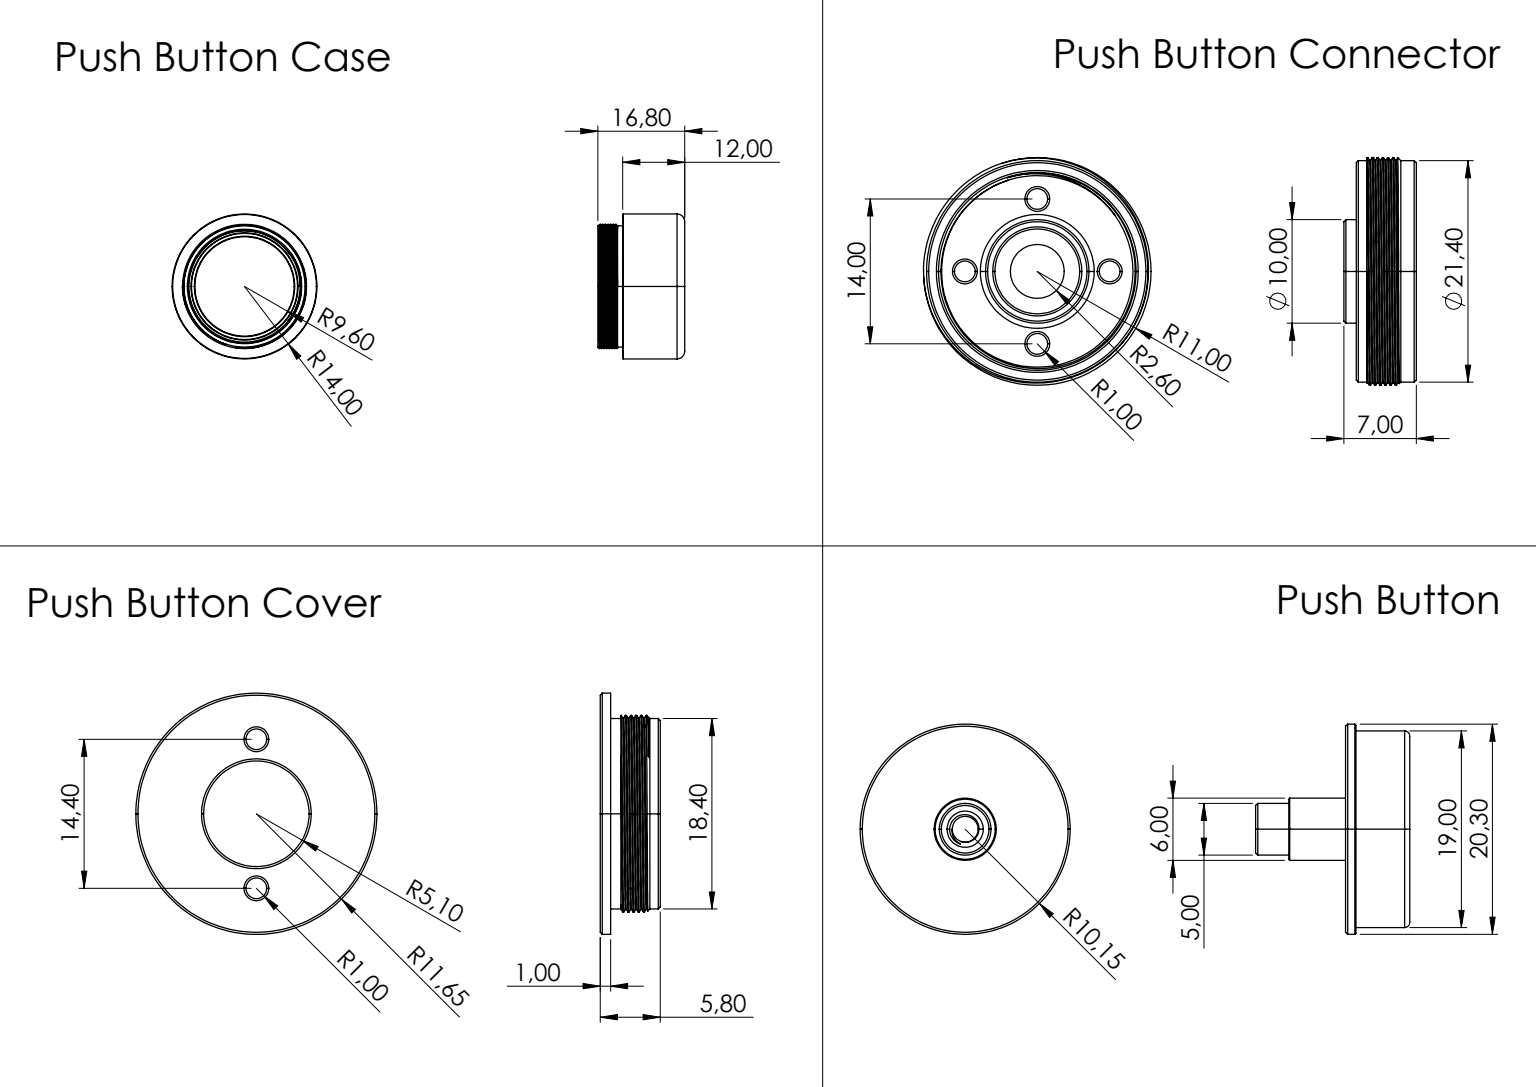
ISO-10303-21;
HEADER;
FILE_DESCRIPTION (('STEP AP214'),
    '1' );
FILE_NAME ('Push Button Connector.step',
    '2026-10-07T19:06:49',
    ( '' ),
    ( '' ),
    'SwSTEP 2.0',
    'SolidWorks 2020',
    '' );
FILE_SCHEMA (( 'AUTOMOTIVE_DESIGN' ));
ENDSEC;

DATA;
#1=CIRCLE ( 'NONE', #2803, 1.199999999999999956 ) ;
#7=CARTESIAN_POINT ( 'NONE',  ( 5.443609589771999602, -77.26340414414998747, 9.675369385899999841 ) ) ;
#13=CARTESIAN_POINT ( 'NONE',  ( 8.944729675425000082, -79.55274183760799644, 3.923329690209000908 ) ) ;
#25=CARTESIAN_POINT ( 'NONE',  ( 8.240135455977000589, -77.95571942709864288, -5.125512367919999868 ) ) ;
#26=CARTESIAN_POINT ( 'NONE',  ( 6.712914363625387182, -79.91051976297769954, 6.366836982130202216 ) ) ;
#27=CARTESIAN_POINT ( 'NONE',  ( -10.75000000000000000, -80.44999999999998863, 5.225043809877999334E-10 ) ) ;
#29=CARTESIAN_POINT ( 'NONE',  ( 7.764258067048000811, -77.05084123326183487, 5.767450660628000492 ) ) ;
#34=B_SPLINE_SURFACE_WITH_KNOTS ( 'NONE', 3, 3, ( 
 ( #2089, #37490, #2662, #20656, #6495, #56101, #24505, #42521, #42233, #28631, #6789, #20087, #38079, #55512, #1505, #24796, #1797, #15059, #42810, #33053, #25080, #24214, #38655, #46967, #15646, #19794, #43104, #51683, #56674, #55808, #19495, #11231, #29210, #7079, #2374 ),
 ( #11521, #15360, #29498, #51101, #47553, #10652, #47257, #41935, #28333, #32758, #46681, #50806, #38365, #51387, #56387, #15937, #33925, #6201, #33354, #10944, #10350, #46384, #5908, #23917, #28924, #44244, #34791, #3513, #4087, #3796, #20938, #21798, #39803, #57525, #44532 ),
 ( #52815, #57816, #48399, #17375, #35362, #53387, #12933, #7650, #48682, #38940, #56957, #21514, #30931, #16518, #48971, #8512, #21224, #17086, #26506, #43963, #3233, #22085, #35069, #40099, #16230, #34209, #53105, #12654, #52246, #30648, #12085, #8226, #43380, #12370, #11803 ),
 ( #39520, #25649, #48118, #7364, #26228, #34499, #29777, #47833, #43675, #25364, #2939, #39229, #52528, #30067, #57242, #16806, #30358, #7936, #25938, #36844, #4690, #584, #41281, #27399, #45139, #46026, #18566, #5547, #54856, #9997, #36557, #54579, #14403, #14119, #53990 ) ),
 .UNSPECIFIED., .F., .F., .F.,
 ( 4, 4 ),
 ( 4, 1, 1, 1, 1, 1, 1, 1, 1, 1, 1, 1, 1, 1, 1, 1, 1, 1, 1, 1, 1, 1, 1, 1, 1, 1, 1, 1, 1, 1, 1, 1, 4 ),
 ( -0.1387574078320999993, 1.138757407831999968 ),
 ( 0.3298824860954999716, 0.3512342696267000131, 0.3725860531579999746, 0.3939378366892999916, 0.4152896202206000087, 0.4366414037517999946, 0.4579931872831000117, 0.4793449708143999732, 0.5006967543456000147, 0.5220485378768999762, 0.5434003214082000488, 0.5647521049395000103, 0.5861038884707000518, 0.6074556720019999023, 0.6288074555332999749, 0.6501592390646000474, 0.6715110225957999779, 0.6928628061271000504, 0.7142145896584000120, 0.7355663731896000535, 0.7569181567209000150, 0.7782699402522000875, 0.7996217237835000491, 0.8209735073147000906, 0.8423252908460000521, 0.8636770743773000136, 0.8850288579085000551, 0.9063806414398000166, 0.9277324249710999782, 0.9490842085024000507, 0.9704359920335999812, 0.9917877755649000537, 1.013139559096000175 ),
 .UNSPECIFIED. ) ;
#41=CARTESIAN_POINT ( 'NONE',  ( 9.855576673225998618, -79.76811006564999218, -5.230603033304000782 ) ) ;
#47=ORIENTED_EDGE ( 'NONE', *, *, #21166, .F. ) ;
#51=DIRECTION ( 'NONE',  ( 0.000000000000000000, 0.000000000000000000, -1.000000000000000000 ) ) ;
#66=CARTESIAN_POINT ( 'NONE',  ( -6.405050160242000246, -78.85473773677898635, 8.912875463421000788 ) ) ;
#67=CARTESIAN_POINT ( 'NONE',  ( 11.00000000000000000, -79.34999999999999432, -1.064824513673000067E-14 ) ) ;
#79=CARTESIAN_POINT ( 'NONE',  ( -5.793600105730999594, -78.22586176634699484, 9.408086495002001115 ) ) ;
#108=CARTESIAN_POINT ( 'NONE',  ( -6.065106684382000068, -77.35143450949497890, 9.224892016835999797 ) ) ;
#116=CARTESIAN_POINT ( 'NONE',  ( 9.009247259181924150, -78.72916666666665719, -2.421167930323326001 ) ) ;
#118=ORIENTED_EDGE ( 'NONE', *, *, #11311, .T. ) ;
#125=EDGE_CURVE ( 'NONE', #28960, #7174, #2934, .T. ) ;
#130=CARTESIAN_POINT ( 'NONE',  ( 11.22519961651999942, -80.38483504313998651, 1.998589004412999692 ) ) ;
#158=CARTESIAN_POINT ( 'NONE',  ( 0.000000000000000000, -75.19999999999998863, -4.999999999999962697 ) ) ;
#163=CARTESIAN_POINT ( 'NONE',  ( -5.539808784079908399, -79.51666666666666572, 9.611650271896829523 ) ) ;
#170=AXIS2_PLACEMENT_3D ( 'NONE', #825, #36799, #54241 ) ;
#173=CARTESIAN_POINT ( 'NONE',  ( -6.000000000000000000, -81.99999999999998579, 0.000000000000000000 ) ) ;
#189=CARTESIAN_POINT ( 'NONE',  ( -7.843978203195000276, -77.65945010111499869, 5.713380375430999969 ) ) ;
#192=DIRECTION ( 'NONE',  ( 0.000000000000000000, -1.000000000000000000, 0.000000000000000000 ) ) ;
#206=CYLINDRICAL_SURFACE ( 'NONE', #36450, 4.100000000000000533 ) ;
#224=CARTESIAN_POINT ( 'NONE',  ( -0.5444512524326000635, -78.07738533478699594, -9.506521396690999381 ) ) ;
#235=CARTESIAN_POINT ( 'NONE',  ( 3.166366903731000271, -79.72244757809599491, 10.47195928638999973 ) ) ;
#236=LINE ( 'NONE', #58354, #29407 ) ;
#244=ORIENTED_EDGE ( 'NONE', *, *, #50771, .T. ) ;
#256=CARTESIAN_POINT ( 'NONE',  ( 7.620617093578522905, -78.80203626096795233, -5.244489908162002223 ) ) ;
#258=CARTESIAN_POINT ( 'NONE',  ( -7.396886230003165252, -77.65219327641052871, -5.684603129138253053 ) ) ;
#262=VECTOR ( 'NONE', #19954, 1000.000000000000000 ) ;
#267=EDGE_CURVE ( 'NONE', #43339, #56949, #56033, .T. ) ;
#271=CARTESIAN_POINT ( 'NONE',  ( 8.599926684958175471, -79.81921486858095705, -3.562059774102686038 ) ) ;
#279=FACE_OUTER_BOUND ( 'NONE', #48060, .T. ) ;
#291=CARTESIAN_POINT ( 'NONE',  ( 0.8649477812003000254, -78.46126277754198952, -9.701111330267998767 ) ) ;
#292=VECTOR ( 'NONE', #35631, 1000.000000000000227 ) ;
#312=CARTESIAN_POINT ( 'NONE',  ( 8.944729675425000082, -79.61304476327899238, 3.923329690209000908 ) ) ;
#323=CARTESIAN_POINT ( 'NONE',  ( -7.203390125892000562, -78.80843430096776103, -6.502451851937000704 ) ) ;
#324=CARTESIAN_POINT ( 'NONE',  ( 8.238920321119756807, -79.88802510210236107, 4.204434926243399318 ) ) ;
#327=CARTESIAN_POINT ( 'NONE',  ( -9.497876546326999403, -77.25168256874098915, -0.2008509664869000122 ) ) ;
#328=CARTESIAN_POINT ( 'NONE',  ( 0.09829970619593025871, -77.22591789683764318, -9.271508350125035491 ) ) ;
#330=AXIS2_PLACEMENT_3D ( 'NONE', #48177, #7132, #57011 ) ;
#349=CARTESIAN_POINT ( 'NONE',  ( -7.229693382246000333, -78.82924743682598034, -6.526195624661000672 ) ) ;
#358=CARTESIAN_POINT ( 'NONE',  ( -9.091539081997000338, -78.88283009111098920, 6.148815634104000338 ) ) ;
#369=CARTESIAN_POINT ( 'NONE',  ( -7.138937464960999790, -79.17331078153999613, 8.574798629027000629 ) ) ;
#390=CARTESIAN_POINT ( 'NONE',  ( -3.539318067648058452, -78.19389790816430263, -8.545993076014068990 ) ) ;
#396=CARTESIAN_POINT ( 'NONE',  ( 1.433348699817989180, -77.46263244500043754, 9.138269204909326149 ) ) ;
#397=CARTESIAN_POINT ( 'NONE',  ( 7.528714304401000312, -78.05456459179299600, -8.074838600060001426 ) ) ;
#399=CARTESIAN_POINT ( 'NONE',  ( 4.186942200393000135, -78.55095460635199345, -8.754440266352000677 ) ) ;
#404=CARTESIAN_POINT ( 'NONE',  ( -10.78159125964999987, -79.41561974942199242, 1.856099740267000087 ) ) ;
#409=VERTEX_POINT ( 'NONE', #50221 ) ;
#410=EDGE_CURVE ( 'NONE', #18942, #44068, #5336, .T. ) ;
#420=CARTESIAN_POINT ( 'NONE',  ( -11.13667185325999931, -80.13800688576898779, -2.444338232200999439 ) ) ;
#426=AXIS2_PLACEMENT_3D ( 'NONE', #17397, #35382, #53716 ) ;
#427=CARTESIAN_POINT ( 'NONE',  ( 9.684822944874866835, -77.90969691107382289, -5.379607873393639217 ) ) ;
#435=AXIS2_PLACEMENT_3D ( 'NONE', #56778, #6892, #24899 ) ;
#444=CARTESIAN_POINT ( 'NONE',  ( 7.559982449049000408, -77.02655527933319490, -6.032732969207000195 ) ) ;
#448=DIRECTION ( 'NONE',  ( 0.000000000000000000, -1.000000000000000000, 0.000000000000000000 ) ) ;
#458=ORIENTED_EDGE ( 'NONE', *, *, #10797, .T. ) ;
#474=CARTESIAN_POINT ( 'NONE',  ( -1.959694873104000257, -77.31836415156699616, -9.504225410855001499 ) ) ;
#491=CARTESIAN_POINT ( 'NONE',  ( 10.25292700656883760, -77.20000000000000284, -3.413936412999044823 ) ) ;
#498=FACE_OUTER_BOUND ( 'NONE', #54806, .T. ) ;
#499=CARTESIAN_POINT ( 'NONE',  ( 3.414307247564000392, -79.67572032229998058, 9.134133468150000823 ) ) ;
#500=EDGE_CURVE ( 'NONE', #21107, #21244, #3663, .T. ) ;
#507=FACE_OUTER_BOUND ( 'NONE', #47869, .T. ) ;
#510=CARTESIAN_POINT ( 'NONE',  ( 1.825776387079000029, -78.88028063292298953, 9.234594473601999809 ) ) ;
#518=PRODUCT_DEFINITION ( 'UNKNOWN', '', #41419, #21544 ) ;
#522=CARTESIAN_POINT ( 'NONE',  ( -10.75843888410000027, -79.38533932610398836, -1.985902594052000092 ) ) ;
#541=CARTESIAN_POINT ( 'NONE',  ( 0.000000000000000000, -74.99999999999998579, 0.000000000000000000 ) ) ;
#547=CARTESIAN_POINT ( 'NONE',  ( -1.374291557126987362, -78.71317509820548253, -9.148177845238967265 ) ) ;
#552=CARTESIAN_POINT ( 'NONE',  ( -9.250401410528953150, -77.61051319238347901, -1.210813435511432834 ) ) ;
#560=CARTESIAN_POINT ( 'NONE',  ( 2.902193781656972504, -80.00000000000000000, 8.901354151454830443 ) ) ;
#568=EDGE_CURVE ( 'NONE', #9279, #11445, #48735, .T. ) ;
#575=B_SPLINE_SURFACE_WITH_KNOTS ( 'NONE', 3, 3, ( 
 ( #12579, #9256, #48608, #54128, #29991, #34424, #52454, #57162, #48044, #8155, #7577, #25576, #21148, #39156, #26155, #46752, #46163, #1286, #33424, #51461, #37270, #11015, #28406, #50289, #28112, #9843, #10723, #36691, #23698, #15430, #1871, #41125, #19565, #36981, #27823, #50582, #28999, #41711, #18989, #45869, #28701, #19280, #54994, #47039, #33127, #19865, #5688, #1004, #6271, #24287, #10136, #23410, #6569, #55285, #42304, #14833, #37859, #55880, #719, #18697, #37566, #14543, #51169, #54706, #14250, #32536, #32830 ),
 ( #50875, #10421, #32246, #46453, #5402, #23988, #5981, #42004, #1572, #41421, #55581, #15129, #56458, #34575, #29282, #39020, #12159, #52608, #20445, #20159, #21300, #11301, #39308, #34863, #48195, #11594, #57318, #2158, #43753, #38441, #47910, #38148, #16012, #25728, #21014, #12443, #25441, #52893, #29855, #34001, #52037, #15718, #43460, #47331, #42886, #34289, #56748, #42596, #2732, #7149, #29570, #20731, #57032, #33714, #47626, #25151, #52323, #6860, #30438, #38729, #7442, #43177, #48469, #11877, #16308, #3017, #16591 ),
 ( #30145, #7727, #3306, #16882, #24580, #56170, #51751, #24868, #2443, #13596, #18336, #36328, #4752, #39595, #49044, #30719, #31886, #48754, #44315, #44035, #40764, #8301, #40472, #8590, #4460, #45204, #54353, #66, #358, #54060, #57892, #53767, #13892, #3871, #22754, #22460, #26578, #31593, #36036, #9182, #21871, #17448, #13006, #8012, #44905, #35736, #44612, #4167, #53464, #22165, #13303, #26009, #49635, #12726, #27167, #3585, #49340, #21588, #40172, #57598, #26301, #17159, #35145, #53176, #39879, #35435, #31006 ),
 ( #58185, #17748, #31296, #8886, #26881, #18044, #32756, #41932, #10348, #1217, #23914, #27461, #41637, #50509, #55510, #46676, #28331, #46381, #6199, #5905, #45796, #1503, #18630, #28042, #24212, #45499, #5331, #5614, #1795, #14179, #42231, #19493, #37199, #14758, #50803, #37488, #19208, #55212, #645, #51098, #15057, #33051, #10649, #28629, #19792, #46088, #37786, #23625, #54641, #36907, #55806, #15358, #49930, #9475, #23044, #32463, #32176, #5046, #50216, #27752, #41059, #36622, #9764, #23338, #10062, #41350, #932 ) ),
 .UNSPECIFIED., .F., .F., .F.,
 ( 4, 4 ),
 ( 4, 1, 1, 1, 1, 1, 1, 1, 1, 1, 1, 1, 1, 1, 1, 1, 1, 1, 1, 1, 1, 1, 1, 1, 1, 1, 1, 1, 1, 1, 1, 1, 1, 1, 1, 1, 1, 1, 1, 1, 1, 1, 1, 1, 1, 1, 1, 1, 1, 1, 1, 1, 1, 1, 1, 1, 1, 1, 1, 1, 1, 1, 1, 1, 4 ),
 ( -0.4045438850611000059, 1.404543885061000141 ),
 ( -0.02000000000000000042, -0.003749999999999999861, 0.01250000000000000069, 0.02875000000000000125, 0.04499999999999999833, 0.06124999999999999889, 0.07749999999999999944, 0.09375000000000000000, 0.1100000000000000006, 0.1262500000000000011, 0.1424999999999999878, 0.1587500000000000022, 0.1749999999999999889, 0.1912500000000000033, 0.2074999999999999900, 0.2237500000000000044, 0.2399999999999999911, 0.2562499999999999778, 0.2725000000000000200, 0.2887500000000000067, 0.3049999999999999933, 0.3212499999999999800, 0.3375000000000000222, 0.3537500000000000089, 0.3699999999999999956, 0.3862499999999999822, 0.4025000000000000244, 0.4187500000000000111, 0.4349999999999999978, 0.4512499999999999845, 0.4675000000000000266, 0.4837500000000000133, 0.5000000000000000000, 0.5162499999999999867, 0.5324999999999999734, 0.5487499999999999600, 0.5649999999999999467, 0.5812500000000000444, 0.5975000000000000311, 0.6137500000000000178, 0.6300000000000000044, 0.6462499999999999911, 0.6624999999999999778, 0.6787499999999999645, 0.6949999999999999512, 0.7112500000000000488, 0.7275000000000000355, 0.7437500000000000222, 0.7600000000000000089, 0.7762499999999999956, 0.7924999999999999822, 0.8087499999999999689, 0.8249999999999999556, 0.8412500000000000533, 0.8575000000000000400, 0.8737500000000000266, 0.8900000000000000133, 0.9062500000000000000, 0.9224999999999999867, 0.9387499999999999734, 0.9549999999999999600, 0.9712499999999999467, 0.9875000000000000444, 1.003749999999999920, 1.020000000000000018 ),
 .UNSPECIFIED. ) ;
#577=AXIS2_PLACEMENT_3D ( 'NONE', #17957, #12922, #35948 ) ;
#582=CARTESIAN_POINT ( 'NONE',  ( -8.623695280723000067, -78.29071980276798115, 4.526762133323999571 ) ) ;
#584=CARTESIAN_POINT ( 'NONE',  ( 5.916979755548000597, -79.44684362032798219, -7.926218594775000348 ) ) ;
#591=ADVANCED_FACE ( 'NONE', ( #7938 ), #54289, .F. ) ;
#596=CARTESIAN_POINT ( 'NONE',  ( -7.370930946996000266, -78.06097405823999225, -8.448440252239999282 ) ) ;
#603=CARTESIAN_POINT ( 'NONE',  ( -4.465297566879000257, -79.92309116543150083, 8.686876450551999085 ) ) ;
#604=VERTEX_POINT ( 'NONE', #30650 ) ;
#614=CARTESIAN_POINT ( 'NONE',  ( 7.027773501905277165, -79.90642805933067905, 6.014294227121073533 ) ) ;
#617=CARTESIAN_POINT ( 'NONE',  ( 2.632967082928999947, -77.10305996719816335, 9.306700570505000769 ) ) ;
#638=CARTESIAN_POINT ( 'NONE',  ( -9.375068251199000002, -78.22531894259199703, -2.204836785425999590 ) ) ;
#645=CARTESIAN_POINT ( 'NONE',  ( 10.74341457190999982, -79.22405656010899122, -2.245675826504000216 ) ) ;
#658=CARTESIAN_POINT ( 'NONE',  ( 10.92979202429999930, -79.06863239632698992, 1.617881315982000245 ) ) ;
#661=VECTOR ( 'NONE', #54709, 1000.000000000000000 ) ;
#665=CARTESIAN_POINT ( 'NONE',  ( 8.318716844523411424, -78.25665627052904938, 7.160083125396178083 ) ) ;
#668=ORIENTED_EDGE ( 'NONE', *, *, #34683, .T. ) ;
#684=ORIENTED_EDGE ( 'NONE', *, *, #58361, .T. ) ;
#687=CARTESIAN_POINT ( 'NONE',  ( -1.468596516428545717, -77.48775315375499417, 9.132634440082403771 ) ) ;
#688=CARTESIAN_POINT ( 'NONE',  ( -10.79754810892000094, -77.44686363549098473, -2.301543980133000211 ) ) ;
#690=CARTESIAN_POINT ( 'NONE',  ( 7.405962610586999340, -77.52424149029599221, -6.270759699041999369 ) ) ;
#695=CARTESIAN_POINT ( 'NONE',  ( -3.661365483191000081, -79.33134268642398013, 10.30932680317000028 ) ) ;
#707=CARTESIAN_POINT ( 'NONE',  ( 0.000000000000000000, -75.19999999999998863, 0.000000000000000000 ) ) ;
#710=CARTESIAN_POINT ( 'NONE',  ( -9.163349670171998085, -78.09756746102598868, -2.155044623588000086 ) ) ;
#719=CARTESIAN_POINT ( 'NONE',  ( 9.233664981878000333, -79.60499486974998717, 5.933249305785000871 ) ) ;
#720=CIRCLE ( 'NONE', #32727, 1.000000000000000000 ) ;
#728=CARTESIAN_POINT ( 'NONE',  ( -11.25716098398999954, -78.18238734777798982, -0.4530573336216000002 ) ) ;
#731=CARTESIAN_POINT ( 'NONE',  ( 7.764258067048000811, -77.13099274720589449, 5.767450660628000492 ) ) ;
#734=CARTESIAN_POINT ( 'NONE',  ( -1.297526016723000053, -78.46556992798305430, -10.89864408161000142 ) ) ;
#735=DIRECTION ( 'NONE',  ( -1.000000000000000000, 0.000000000000000000, 0.000000000000000000 ) ) ;
#753=CARTESIAN_POINT ( 'NONE',  ( 3.185848383111141935, -78.25305747739967899, -8.692436244180706595 ) ) ;
#763=CARTESIAN_POINT ( 'NONE',  ( 2.260091721765999928, -78.85325092453199147, -9.437303113984999214 ) ) ;
#779=CARTESIAN_POINT ( 'NONE',  ( 0.04837777540751588695, -77.19999999999998863, -10.99285280508881080 ) ) ;
#780=EDGE_LOOP ( 'NONE', ( #684, #45447, #45553, #30245 ) ) ;
#781=CARTESIAN_POINT ( 'NONE',  ( -1.439896632895311113, -78.31458333333333144, -11.00000000000000355 ) ) ;
#784=CARTESIAN_POINT ( 'NONE',  ( 5.348414924440999307, -79.50038437275298975, -8.153793349671000001 ) ) ;
#787=EDGE_CURVE ( 'NONE', #12448, #10446, #50841, .T. ) ;
#789=CYLINDRICAL_SURFACE ( 'NONE', #25534, 11.00000000000000000 ) ;
#792=CARTESIAN_POINT ( 'NONE',  ( -11.06454125523000087, -77.73236022357899344, 1.497041118686999850 ) ) ;
#795=CARTESIAN_POINT ( 'NONE',  ( 4.459991035765999534, -77.79314704349698673, 8.413017068390001185 ) ) ;
#804=EDGE_LOOP ( 'NONE', ( #53108, #929, #5072, #12373 ) ) ;
#825=CARTESIAN_POINT ( 'NONE',  ( 0.000000000000000000, -74.64999999999999147, 0.000000000000000000 ) ) ;
#833=CARTESIAN_POINT ( 'NONE',  ( 0.03267024647290020511, -78.72542977318258295, -9.249861488902391571 ) ) ;
#836=CARTESIAN_POINT ( 'NONE',  ( -9.170121691637055150, -80.14671525588798318, -6.075096402074364299 ) ) ;
#841=CIRCLE ( 'NONE', #12100, 9.250000000000000000 ) ;
#854=FACE_OUTER_BOUND ( 'NONE', #17770, .T. ) ;
#870=VECTOR ( 'NONE', #48376, 1000.000000000000000 ) ;
#878=CARTESIAN_POINT ( 'NONE',  ( 8.003872304214999289, -77.24441679105500214, -8.008117534469000987 ) ) ;
#884=CARTESIAN_POINT ( 'NONE',  ( 6.728605944993000243, -79.69578255762351660, -7.080011783993000130 ) ) ;
#897=CARTESIAN_POINT ( 'NONE',  ( 9.249687267056886597, -79.85225412240586707, 0.2014328667283708241 ) ) ;
#910=CARTESIAN_POINT ( 'NONE',  ( 9.386754667005000385, -79.85238712864799027, 6.031619700400000283 ) ) ;
#922=ADVANCED_FACE ( 'NONE', ( #50957, #28492, #5484, #46543, #10509, #6065 ), #55373, .F. ) ;
#925=CARTESIAN_POINT ( 'NONE',  ( 8.177883213696999221, -77.91265682217398592, -5.086790354254000057 ) ) ;
#929=ORIENTED_EDGE ( 'NONE', *, *, #4950, .T. ) ;
#931=CARTESIAN_POINT ( 'NONE',  ( 5.684875707061095795, -77.92308321104999891, 7.397310562483891516 ) ) ;
#932=CARTESIAN_POINT ( 'NONE',  ( -10.69701368780000017, -79.98255012709098821, 1.066019776055000090 ) ) ;
#933=CARTESIAN_POINT ( 'NONE',  ( -10.71369944335147473, -79.12083333333333712, -2.879226727952079123 ) ) ;
#951=CARTESIAN_POINT ( 'NONE',  ( -2.421167930323375295, -79.89583333333331439, 9.009247259181911716 ) ) ;
#952=CARTESIAN_POINT ( 'NONE',  ( -0.5194061720425894313, -79.07133454617610369, -10.96348649343952353 ) ) ;
#955=EDGE_LOOP ( 'NONE', ( #118, #10532, #10822 ) ) ;
#960=CARTESIAN_POINT ( 'NONE',  ( 10.63539757175482059, -80.28072916675431259, -2.857308679526295414 ) ) ;
#971=CARTESIAN_POINT ( 'NONE',  ( 8.041760575514985021, -77.39131006114457989, 4.573409923808502420 ) ) ;
#972=CARTESIAN_POINT ( 'NONE',  ( -11.00724581733999941, -77.92400926547099971, 0.8512868710715000287 ) ) ;
#979=DIRECTION ( 'NONE',  ( 0.000000000000000000, 0.000000000000000000, -1.000000000000000000 ) ) ;
#980=CARTESIAN_POINT ( 'NONE',  ( 5.312973029106999867, -78.26383322178199364, 9.563478878364000124 ) ) ;
#988=FACE_OUTER_BOUND ( 'NONE', #44636, .T. ) ;
#994=FACE_OUTER_BOUND ( 'NONE', #35902, .T. ) ;
#997=FACE_OUTER_BOUND ( 'NONE', #46850, .T. ) ;
#999=ORIENTED_EDGE ( 'NONE', *, *, #41614, .F. ) ;
#1000=EDGE_CURVE ( 'NONE', #57298, #36426, #32062, .T. ) ;
#1001=CARTESIAN_POINT ( 'NONE',  ( 0.000000000000000000, -77.49999999999998579, 0.000000000000000000 ) ) ;
#1004=CARTESIAN_POINT ( 'NONE',  ( -10.81649518602000093, -79.29597897209099244, 1.862108609190000097 ) ) ;
#1033=VERTEX_POINT ( 'NONE', #32844 ) ;
#1040=CARTESIAN_POINT ( 'NONE',  ( 6.432069509746887626, -78.28619479064511211, -6.649389305992823296 ) ) ;
#1043=VERTEX_POINT ( 'NONE', #41143 ) ;
#1049=CARTESIAN_POINT ( 'NONE',  ( 4.545264886168000729, -77.60605771026999378, 8.573871732259998879 ) ) ;
#1065=B_SPLINE_CURVE_WITH_KNOTS ( 'NONE', 3,
 ( #13567, #49605, #16421, #24978, #38844, #21128, #30263, #34404, #16710, #29972, #33825, #29683, #34692, #38265, #33540, #29398, #51864, #11709, #47158 ),
 .UNSPECIFIED., .F., .F.,
 ( 4, 1, 1, 1, 1, 1, 1, 1, 1, 1, 1, 1, 1, 1, 1, 1, 4 ),
 ( 0.000000000000000000, 0.04500013125675292325, 0.1100001148193760075, 0.1750000983819555711, 0.2400000819445786693, 0.3050000655072017119, 0.3700000490698248656, 0.4350000326324479638, 0.5000000161948968680, 0.5649999997576505839, 0.6299999833204042998, 0.6949999668831581268, 0.7599999504454763022, 0.8249999340082300181, 0.8899999175709837340, 0.9549999011333020205, 1.000000000000000000 ),
 .UNSPECIFIED. ) ;
#1066=VERTEX_POINT ( 'NONE', #5137 ) ;
#1072=CARTESIAN_POINT ( 'NONE',  ( -0.09271117443256000901, -79.70494298055800186, 9.750963687110999700 ) ) ;
#1077=DIRECTION ( 'NONE',  ( 0.000000000000000000, 0.000000000000000000, -1.000000000000000000 ) ) ;
#1078=CARTESIAN_POINT ( 'NONE',  ( 4.884263559594000270, -77.83984273478799309, -10.16119218727999929 ) ) ;
#1079=EDGE_CURVE ( 'NONE', #43122, #24529, #36790, .T. ) ;
#1083=CARTESIAN_POINT ( 'NONE',  ( 3.151000900302999952, -78.36865170860198759, 8.870309342620000592 ) ) ;
#1088=CARTESIAN_POINT ( 'NONE',  ( 0.000000000000000000, -80.99999999999998579, 0.000000000000000000 ) ) ;
#1094=ORIENTED_EDGE ( 'NONE', *, *, #7570, .F. ) ;
#1108=CIRCLE ( 'NONE', #35958, 5.000000000000000000 ) ;
#1111=CARTESIAN_POINT ( 'NONE',  ( 6.983681292383111305, -78.53882967120196668, -6.738102358712994011 ) ) ;
#1117=CARTESIAN_POINT ( 'NONE',  ( 0.3203968975889366910, -78.72793535945164933, -9.244731248301008009 ) ) ;
#1121=CARTESIAN_POINT ( 'NONE',  ( -9.147467037885974150, -80.14699925185365714, -6.109202993256466208 ) ) ;
#1129=CARTESIAN_POINT ( 'NONE',  ( 9.499693205731109202, -80.00008708754018016, -1.997583897032410100E-06 ) ) ;
#1131=EDGE_CURVE ( 'NONE', #31999, #28960, #48632, .T. ) ;
#1138=CARTESIAN_POINT ( 'NONE',  ( 10.68454778250440640, -77.21060221147246239, 1.377222071623238620 ) ) ;
#1141=CARTESIAN_POINT ( 'NONE',  ( -2.928603948516999900, -78.74649347130959143, 10.57767911663000149 ) ) ;
#1148=CARTESIAN_POINT ( 'NONE',  ( 8.244325742278693525, -78.31259323136428918, -4.194771269908470934 ) ) ;
#1152=CARTESIAN_POINT ( 'NONE',  ( 1.867960828343000035, -78.75252915135698117, 9.447959161044998666 ) ) ;
#1153=DIRECTION ( 'NONE',  ( 0.000000000000000000, -1.000000000000000000, 0.000000000000000000 ) ) ;
#1165=CARTESIAN_POINT ( 'NONE',  ( -11.07550907487999936, -77.92372890012597964, 0.7607607059370000702 ) ) ;
#1172=CARTESIAN_POINT ( 'NONE',  ( 9.523132023602000729, -80.26946618684752366, 1.108936319727999997 ) ) ;
#1178=EDGE_CURVE ( 'NONE', #29062, #16887, #38796, .T. ) ;
#1183=CARTESIAN_POINT ( 'NONE',  ( 9.707557378189999753, -77.00399869373629258, -2.082535605504000298 ) ) ;
#1207=CARTESIAN_POINT ( 'NONE',  ( -2.552693750765000047, -78.31059042997900121, -9.286385980553001573 ) ) ;
#1211=ORIENTED_EDGE ( 'NONE', *, *, #32322, .T. ) ;
#1214=CARTESIAN_POINT ( 'NONE',  ( 4.658318423525466656, -77.93349885897991669, 8.082338094468221712 ) ) ;
#1217=CARTESIAN_POINT ( 'NONE',  ( -5.755176823513999729, -78.40937828446098479, 9.345691860246999383 ) ) ;
#1224=AXIS2_PLACEMENT_3D ( 'NONE', #7015, #33862, #6432 ) ;
#1231=CARTESIAN_POINT ( 'NONE',  ( 0.000000000000000000, -77.19999999999998863, 0.000000000000000000 ) ) ;
#1236=CARTESIAN_POINT ( 'NONE',  ( 9.694993915875986801, -79.66127398716234609, -5.145377715137363417 ) ) ;
#1237=LINE ( 'NONE', #18653, #57315 ) ;
#1238=ORIENTED_EDGE ( 'NONE', *, *, #38746, .F. ) ;
#1256=CARTESIAN_POINT ( 'NONE',  ( 8.765487326333861517, -77.37590140598007338, 2.954454027020771978 ) ) ;
#1264=LINE ( 'NONE', #48090, #9187 ) ;
#1265=CARTESIAN_POINT ( 'NONE',  ( 7.294482259529999624, -79.61226622975098621, -8.153425347847999660 ) ) ;
#1274=CARTESIAN_POINT ( 'NONE',  ( 0.000000000000000000, -80.35000000001998899, 0.000000000000000000 ) ) ;
#1277=CARTESIAN_POINT ( 'NONE',  ( -2.495045882587000108, -78.18283894841299286, -9.076670124625998426 ) ) ;
#1286=CARTESIAN_POINT ( 'NONE',  ( 2.550499813263000348, -78.45320834210998839, -10.67515654612000020 ) ) ;
#1288=EDGE_CURVE ( 'NONE', #26886, #33815, #5598, .T. ) ;
#1297=CARTESIAN_POINT ( 'NONE',  ( -2.226613147434000073, -78.07001793044798887, 11.04405396508999893 ) ) ;
#1305=VECTOR ( 'NONE', #37563, 1000.000000000000000 ) ;
#1308=CONICAL_SURFACE ( 'NONE', #57824, 9.431249999994999911, 0.7853981633972997312 ) ;
#1313=EDGE_LOOP ( 'NONE', ( #17606, #9356, #29670, #17047, #4604 ) ) ;
#1316=ORIENTED_EDGE ( 'NONE', *, *, #31004, .F. ) ;
#1323=CARTESIAN_POINT ( 'NONE',  ( 1.902005808056935310, -78.24161995856391627, -9.052334553967094521 ) ) ;
#1327=CARTESIAN_POINT ( 'NONE',  ( -8.805853231905880207, -77.57526559296016444, 2.831825794683833220 ) ) ;
#1331=CARTESIAN_POINT ( 'NONE',  ( -6.766389538252999714, -77.83344834330198125, -6.956053621355001049 ) ) ;
#1332=DIRECTION ( 'NONE',  ( -1.000000000000000000, 0.000000000000000000, 0.000000000000000000 ) ) ;
#1346=CARTESIAN_POINT ( 'NONE',  ( -1.210648453353548426, -79.48564454928481382, 9.248615044363743820 ) ) ;
#1349=CARTESIAN_POINT ( 'NONE',  ( 9.865351076058296087, -77.19999999999998863, -4.411030472467261987 ) ) ;
#1350=EDGE_LOOP ( 'NONE', ( #56104, #21727, #7177, #50239 ) ) ;
#1353=CARTESIAN_POINT ( 'NONE',  ( 1.439896632895317108, -79.06458333333331723, 10.99999999999999822 ) ) ;
#1357=DIRECTION ( 'NONE',  ( 0.000000000000000000, 0.000000000000000000, -1.000000000000000000 ) ) ;
#1359=CARTESIAN_POINT ( 'NONE',  ( -6.565417933280000895, -77.81803934957498825, -9.031084880605000365 ) ) ;
#1363=CARTESIAN_POINT ( 'NONE',  ( -8.420145992286000691, -77.48751300560297750, 3.744741888101000171 ) ) ;
#1383=ORIENTED_EDGE ( 'NONE', *, *, #50103, .T. ) ;
#1385=ORIENTED_EDGE ( 'NONE', *, *, #17552, .F. ) ;
#1394=CARTESIAN_POINT ( 'NONE',  ( 9.703646361260002351, -77.60084330994595803, 0.1143463288009116258 ) ) ;
#1397=B_SPLINE_CURVE_WITH_KNOTS ( 'NONE', 3,
 ( #16488, #34467, #48651, #35328, #26198, #53356, #25907, #12337, #48937, #12902, #30902, #39194, #43644, #8479, #43930, #16776, #22052, #21193, #52497, #39491, #48088, #57493, #3202, #12622, #30326, #40061, #48367, #17056, #35037, #53072, #14366, #49826, #14656, #54541, #37096, #41243, #23523, #9372, #40663, #36227, #35927, #27939, #54249, #256, #32654, #50706, #18239, #55112, #58374, #10246, #45987, #41534, #13782, #5233, #53957, #40957, #28229, #19104, #17936, #36805, #31783, #27362, #4942, #46281, #54824, #45694, #13494, #5806, #5514, #18524, #23237, #23813, #1117, #4655, #31485, #49530, #833, #9076, #36516, #27063, #22653, #32077, #45101, #45399, #22947, #547, #14082, #32366, #50118, #9662, #18814, #27652, #50409, #9959, #20561, #46867, #42711, #24982, #11138, #28818, #29685, #42127, #11711, #47737, #33828, #51866, #41831, #15252, #11419, #46575, #56289, #29400, #47453, #37687, #37388, #38559, #28526, #56575, #52153, #6978, #19987, #16133, #7270, #10842, #34110, #32949, #6394, #6101, #37976, #15840, #50993, #24409, #33244, #29114, #24110, #1405, #19396, #15546, #6690, #33542, #51581, #47160, #24699, #10542, #43003, #2560, #55407, #1693, #14952, #19686, #2277, #42425, #55703, #20274, #51287, #1994, #55999, #38268, #25271, #3704, #21130, #34695, #30265, #17578, #21708, #12562, #43290, #44438, #53299, #43874, #30560, #13130, #12844, #29974, #30843, #48877, #8137, #53591, #3423, #40001, #48025, #57439, #26416, #3990, #8419, #21993, #16712, #57719, #7559, #25558, #48591, #58016, #43578, #35565 ),
 .UNSPECIFIED., .F., .F.,
 ( 4, 2, 2, 1, 1, 1, 1, 1, 2, 2, 2, 2, 2, 1, 1, 1, 1, 1, 2, 2, 2, 2, 2, 1, 1, 1, 1, 2, 2, 2, 2, 2, 2, 2, 2, 1, 1, 1, 1, 2, 2, 2, 2, 2, 2, 2, 1, 1, 1, 1, 1, 2, 2, 2, 2, 2, 1, 1, 1, 2, 2, 2, 2, 1, 1, 1, 2, 2, 2, 2, 1, 1, 1, 1, 1, 2, 2, 2, 2, 2, 1, 1, 1, 2, 2, 2, 1, 2, 2, 1, 1, 2, 2, 2, 2, 2, 1, 2, 2, 2, 2, 2, 2, 2, 2, 1, 1, 1, 2, 2, 2, 2, 2, 2, 2, 2, 1, 1, 2, 4 ),
 ( 0.000000000000000000, 0.03124999999998840511, 0.04687499999998261807, 0.05468749999997975231, 0.05859374999997830208, 0.06054687499997758043, 0.06152343749997721267, 0.06201171874997703226, 0.06225585937497695593, 0.06249999999997687961, 0.09374999999996236344, 0.1093749999999550915, 0.1171874999999514694, 0.1210937499999496514, 0.1230468749999487216, 0.1240234374999482914, 0.1245117187499480693, 0.1247558593749479861, 0.1248779296874479167, 0.1249999999999478612, 0.1562499999999539535, 0.1718749999999570344, 0.1796874999999586442, 0.1835937499999594491, 0.1855468749999598932, 0.1865234374999601152, 0.1870117187499601985, 0.1872558593749602263, 0.1874999999999602263, 0.2031249999999644174, 0.2109374999999664713, 0.2148437499999675537, 0.2187499999999686362, 0.2343749999999729661, 0.2421874999999751310, 0.2460937499999762690, 0.2480468749999769074, 0.2490234374999772959, 0.2495117187499775180, 0.2497558593749775180, 0.2499999999999775180, 0.3124999999999837352, 0.3749999999999899525, 0.4374999999999962252, 0.4687499999999993894, 0.4843750000000009437, 0.4921875000000017208, 0.4960937500000021094, 0.4980468750000022760, 0.4990234375000023870, 0.4995117187500023870, 0.4997558593750024425, 0.5000000000000024425, 0.5312500000000072164, 0.5468750000000095479, 0.5546875000000107692, 0.5585937500000113243, 0.5605468750000116573, 0.5615234375000117684, 0.5620117187500118794, 0.5625000000000118794, 0.5937500000000155431, 0.6093750000000173195, 0.6171875000000182077, 0.6210937500000186517, 0.6230468750000188738, 0.6240234375000189848, 0.6250000000000189848, 0.6562500000000210942, 0.6718750000000220934, 0.6796875000000224265, 0.6835937500000226485, 0.6855468750000228706, 0.6865234375000229816, 0.6870117187500229816, 0.6872558593750229816, 0.6875000000000229816, 0.7187500000000279776, 0.7343750000000304201, 0.7421875000000316414, 0.7460937500000323075, 0.7480468750000325295, 0.7490234375000327516, 0.7495117187500327516, 0.7500000000000327516, 0.7812500000000329736, 0.7851562500000329736, 0.7856445312500329736, 0.7861328125000330846, 0.7871093750000330846, 0.7890625000000331957, 0.7968750000000335287, 0.8125000000000343059, 0.8203125000000346390, 0.8212890625000344169, 0.8222656250000343059, 0.8242187500000338618, 0.8281250000000331957, 0.8437500000000311973, 0.8515625000000301981, 0.8593750000000291989, 0.8750000000000273115, 0.8906250000000254241, 0.8925781250000250910, 0.8930664062500248690, 0.8935546875000247580, 0.8945312500000244249, 0.8984375000000235367, 0.9062500000000217604, 0.9375000000000144329, 0.9453125000000125455, 0.9492187500000116573, 0.9531250000000107692, 0.9687500000000071054, 0.9726562500000062172, 0.9736328125000059952, 0.9746093750000057732, 0.9765625000000053291, 0.9843750000000035527, 1.000000000000000000 ),
 .UNSPECIFIED. ) ;
#1398=CARTESIAN_POINT ( 'NONE',  ( -8.771427373352999268, -77.78517645232463451, -4.151237309591000013 ) ) ;
#1405=CARTESIAN_POINT ( 'NONE',  ( -7.198099468258734035, -78.65408334510459554, -5.809580251814940866 ) ) ;
#1408=DIRECTION ( 'NONE',  ( 1.000000000000000000, 0.000000000000000000, 0.000000000000000000 ) ) ;
#1418=CARTESIAN_POINT ( 'NONE',  ( 1.101534974885716833, -79.99999999999997158, 9.249201346533595824 ) ) ;
#1423=CARTESIAN_POINT ( 'NONE',  ( 9.250054636821570142, -79.84526209104460293, -0.6055073710143449306 ) ) ;
#1431=CARTESIAN_POINT ( 'NONE',  ( 9.233664981878000333, -79.64544880995556753, 5.933249305785000871 ) ) ;
#1436=CARTESIAN_POINT ( 'NONE',  ( 7.548260755434943903, -78.30112507871334060, -5.346425350760562800 ) ) ;
#1440=CARTESIAN_POINT ( 'NONE',  ( 6.930806504809000401, -78.58198617658298701, -6.687086896242999678 ) ) ;
#1442=CARTESIAN_POINT ( 'NONE',  ( -1.000000000000000000, -81.99999999999998579, -7.000000000000000000 ) ) ;
#1443=DIRECTION ( 'NONE',  ( 0.000000000000000000, 1.000000000000000000, 0.000000000000000000 ) ) ;
#1447=ORIENTED_EDGE ( 'NONE', *, *, #10114, .F. ) ;
#1453=CARTESIAN_POINT ( 'NONE',  ( -8.699139934798001406, -77.54738813692499377, -7.073312318721999503 ) ) ;
#1461=CARTESIAN_POINT ( 'NONE',  ( -9.687172913667000174, -80.02050914020550465, -1.248753675804000096 ) ) ;
#1465=EDGE_CURVE ( 'NONE', #49740, #9279, #54779, .T. ) ;
#1471=CARTESIAN_POINT ( 'NONE',  ( -1.850935023731000051, -77.10928756760588954, 9.663325317366000533 ) ) ;
#1489=CARTESIAN_POINT ( 'NONE',  ( 7.792609338710000166, -77.13002767319579789, 5.788510568612999840 ) ) ;
#1494=CARTESIAN_POINT ( 'NONE',  ( -4.491587152465999822, -78.85767126595499121, -8.642068059767000321 ) ) ;
#1501=CARTESIAN_POINT ( 'NONE',  ( 9.250000000000000000, -77.84999999999999432, 0.000000000000000000 ) ) ;
#1503=CARTESIAN_POINT ( 'NONE',  ( 10.94409238582999855, -78.74648653645297713, 0.8311789410725000105 ) ) ;
#1505=CARTESIAN_POINT ( 'NONE',  ( -6.756755724436000143, -79.51665000578398690, 6.762936965852000881 ) ) ;
#1509=ADVANCED_FACE ( 'NONE', ( #10204 ), #6533, .F. ) ;
#1520=CARTESIAN_POINT ( 'NONE',  ( 10.92224869643393070, -78.20263265991563628, 0.3426835237561569047 ) ) ;
#1524=VERTEX_POINT ( 'NONE', #16378 ) ;
#1541=CARTESIAN_POINT ( 'NONE',  ( 8.744325593625859483, -77.37646171839476494, 3.016781543199777094 ) ) ;
#1544=CARTESIAN_POINT ( 'NONE',  ( 4.545264886168000729, -77.72666356161099088, 8.573871732259998879 ) ) ;
#1549=CARTESIAN_POINT ( 'NONE',  ( -6.447812191272999982, -78.91764840355199340, 8.972380486426999369 ) ) ;
#1562=CARTESIAN_POINT ( 'NONE',  ( -9.411482030169999291, -78.58077255621898871, -0.1876179646513999877 ) ) ;
#1572=CARTESIAN_POINT ( 'NONE',  ( -2.169167664939000151, -78.26068007878699007, 10.75912301088999889 ) ) ;
#1573=DIRECTION ( 'NONE',  ( 0.000000000000000000, -1.000000000000000000, 0.000000000000000000 ) ) ;
#1585=CARTESIAN_POINT ( 'NONE',  ( 9.267785752250999209, -77.88273556822998955, -6.128505448192000493 ) ) ;
#1590=DIRECTION ( 'NONE',  ( -1.000000000000000000, 0.000000000000000000, 0.000000000000000000 ) ) ;
#1603=VERTEX_POINT ( 'NONE', #57101 ) ;
#1609=CARTESIAN_POINT ( 'NONE',  ( 6.558477970958472625, -78.28771851464713905, -6.522947137475199497 ) ) ;
#1611=EDGE_CURVE ( 'NONE', #3961, #32937, #13372, .T. ) ;
#1613=VERTEX_POINT ( 'NONE', #15795 ) ;
#1620=CARTESIAN_POINT ( 'NONE',  ( 9.051070938631999852, -77.54921005201198625, 3.499832029064999794 ) ) ;
#1638=DIRECTION ( 'NONE',  ( 0.000000000000000000, 1.000000000000000000, 0.000000000000000000 ) ) ;
#1640=CARTESIAN_POINT ( 'NONE',  ( 3.469760739495959978, -77.20000000000000284, -10.38643556155824577 ) ) ;
#1645=CARTESIAN_POINT ( 'NONE',  ( 6.760013919724070064, -79.02291666666666003, 8.796335266379978535 ) ) ;
#1647=CARTESIAN_POINT ( 'NONE',  ( 1.640398859540999954, -80.09569838644598860, -9.391438764149000917 ) ) ;
#1653=CARTESIAN_POINT ( 'NONE',  ( -8.051994348227001552, -77.30396459359899097, -7.735023745693999864 ) ) ;
#1656=CARTESIAN_POINT ( 'NONE',  ( -5.004442145019999622, -77.60120832211899256, -7.972877152348999630 ) ) ;
#1662=VECTOR ( 'NONE', #23671, 1000.000000000000000 ) ;
#1664=DIRECTION ( 'NONE',  ( 0.000000000000000000, 0.000000000000000000, -1.000000000000000000 ) ) ;
#1680=ORIENTED_EDGE ( 'NONE', *, *, #30027, .T. ) ;
#1689=CARTESIAN_POINT ( 'NONE',  ( 7.658860137759998743, -78.55261983880677690, 5.959242465009999989 ) ) ;
#1693=CARTESIAN_POINT ( 'NONE',  ( -7.826484408841155371, -78.64491150884613546, -4.930180270834215506 ) ) ;
#1696=CYLINDRICAL_SURFACE ( 'NONE', #3139, 1.000000000000000000 ) ;
#1697=CARTESIAN_POINT ( 'NONE',  ( -3.823994368487737994, -80.19708611470613846, -10.32339281103722328 ) ) ;
#1706=CARTESIAN_POINT ( 'NONE',  ( 0.7369903609914696396, -80.00000000000000000, 9.280290198084212960 ) ) ;
#1716=CARTESIAN_POINT ( 'NONE',  ( 6.075386672233462626, -78.12318722923399150, -8.895901220742821636 ) ) ;
#1719=CARTESIAN_POINT ( 'NONE',  ( 6.718030245586000149, -79.02741701463656909, -8.679405866825000260 ) ) ;
#1729=CARTESIAN_POINT ( 'NONE',  ( -3.549595971449000409, -78.23387214450998783, 9.069733410961998032 ) ) ;
#1741=DIRECTION ( 'NONE',  ( 0.000000000000000000, 1.000000000000000000, 0.000000000000000000 ) ) ;
#1744=CARTESIAN_POINT ( 'NONE',  ( -8.784718048239000154, -77.61126387770899271, -7.142896292375000122 ) ) ;
#1751=CARTESIAN_POINT ( 'NONE',  ( 8.249323304235000265, -80.09549224630299591, -5.229696851825000437 ) ) ;
#1763=CARTESIAN_POINT ( 'NONE',  ( -1.834092791198999928, -77.05770150572999455, 9.575395719654000715 ) ) ;
#1785=CARTESIAN_POINT ( 'NONE',  ( 9.546865209729000767, -78.00495639208598675, -1.927967938976999918 ) ) ;
#1788=CARTESIAN_POINT ( 'NONE',  ( 3.747727186550271483, -77.85250684441733426, -10.42547443909606919 ) ) ;
#1795=CARTESIAN_POINT ( 'NONE',  ( -9.091539081997000338, -78.94313301678198513, 6.148815634104000338 ) ) ;
#1797=CARTESIAN_POINT ( 'NONE',  ( 1.463649432154999985, -79.44195468926798753, 9.447158020454001104 ) ) ;
#1815=CARTESIAN_POINT ( 'NONE',  ( 0.9090516009123569274, -78.81850335718206679, 10.93807314156140542 ) ) ;
#1817=ORIENTED_EDGE ( 'NONE', *, *, #6048, .F. ) ;
#1818=ORIENTED_EDGE ( 'NONE', *, *, #32581, .T. ) ;
#1823=ADVANCED_FACE ( 'NONE', ( #39668 ), #54136, .F. ) ;
#1829=CARTESIAN_POINT ( 'NONE',  ( -11.00000000000000000, -77.19999999999998863, 5.688460190305999883E-13 ) ) ;
#1833=DIRECTION ( 'NONE',  ( 0.7071067811865474617, -0.7071067811865474617, 3.010143267812197750E-10 ) ) ;
#1835=CARTESIAN_POINT ( 'NONE',  ( 9.215540093376933584, -77.35694448704265369, 0.7975452914727456655 ) ) ;
#1836=CARTESIAN_POINT ( 'NONE',  ( -0.5413127449341000874, -78.11155102580298148, -11.02683867434999954 ) ) ;
#1845=CARTESIAN_POINT ( 'NONE',  ( 11.04877620194000087, -78.24343189956698552, 0.05135089858452999978 ) ) ;
#1851=CARTESIAN_POINT ( 'NONE',  ( -10.82422835087974278, -77.20000000000001705, 1.830986660789992504 ) ) ;
#1859=CARTESIAN_POINT ( 'NONE',  ( -6.987523971486999663, -78.63762021447698203, -6.307590925213999888 ) ) ;
#1871=CARTESIAN_POINT ( 'NONE',  ( -10.90760146693999921, -78.81840894843499257, -1.219937219691999974 ) ) ;
#1890=CIRCLE ( 'NONE', #16031, 9.549999999999998934 ) ;
#1898=ORIENTED_EDGE ( 'NONE', *, *, #44653, .F. ) ;
#1907=CARTESIAN_POINT ( 'NONE',  ( 6.614009670233677696, -78.28839456110405592, -6.466760316368186601 ) ) ;
#1909=ORIENTED_EDGE ( 'NONE', *, *, #16619, .F. ) ;
#1916=CARTESIAN_POINT ( 'NONE',  ( 4.186942200393000135, -78.43034875501000158, -8.754440266352000677 ) ) ;
#1931=DIRECTION ( 'NONE',  ( 0.000000000000000000, 1.000000000000000000, 0.000000000000000000 ) ) ;
#1938=CARTESIAN_POINT ( 'NONE',  ( 9.611650271896843734, -78.40833333333330302, -5.539808784079876425 ) ) ;
#1942=CARTESIAN_POINT ( 'NONE',  ( -9.629491761460998944, -79.38892416398799412, 0.5011777547001000643 ) ) ;
#1947=FACE_OUTER_BOUND ( 'NONE', #780, .T. ) ;
#1948=CARTESIAN_POINT ( 'NONE',  ( -7.895114074556000006, -77.43171607516499932, -7.584319138910000646 ) ) ;
#1953=CARTESIAN_POINT ( 'NONE',  ( -9.163349670171998085, -78.53919468337598175, -2.155044623588000086 ) ) ;
#1961=CARTESIAN_POINT ( 'NONE',  ( 4.999999999872000167, -80.49999999987198862, -4.857398774947999725E-10 ) ) ;
#1988=CARTESIAN_POINT ( 'NONE',  ( 0.8618009059429999619, -78.38207686403322327, -9.665816497589000633 ) ) ;
#1994=CARTESIAN_POINT ( 'NONE',  ( -8.040862526687783784, -78.64132310946500581, -4.575129970445035887 ) ) ;
#1997=CARTESIAN_POINT ( 'NONE',  ( -7.031989167851816269, -80.17030741383769055, -8.461875502256187787 ) ) ;
#2006=CARTESIAN_POINT ( 'NONE',  ( -6.969094100096229205, -79.65772208930626164, -6.112482804795786429 ) ) ;
#2012=CARTESIAN_POINT ( 'NONE',  ( 0.3028628213633383637, -77.57767551470611522, -10.76873991355842008 ) ) ;
#2014=CARTESIAN_POINT ( 'NONE',  ( 3.915498778898000687, -79.19597114063257948, 10.25343288338999947 ) ) ;
#2019=CARTESIAN_POINT ( 'NONE',  ( 9.235083398947233846, -78.34478105551114879, -0.6060572195536756412 ) ) ;
#2023=CARTESIAN_POINT ( 'NONE',  ( 9.546865209729000767, -78.06332916973599367, -1.927967938976999918 ) ) ;
#2027=ORIENTED_EDGE ( 'NONE', *, *, #34529, .T. ) ;
#2031=CARTESIAN_POINT ( 'NONE',  ( -1.306188688584000168, -78.42250824667499387, -10.97140668998000024 ) ) ;
#2032=CARTESIAN_POINT ( 'NONE',  ( -3.586137557470999937, -80.27811558971397687, -10.61272749461999965 ) ) ;
#2036=CARTESIAN_POINT ( 'NONE',  ( -2.871267467966999831, -78.16153450768899802, -10.95208408865000216 ) ) ;
#2044=CARTESIAN_POINT ( 'NONE',  ( 9.226480760116999136, -79.24116534201449724, -2.263195259622999611 ) ) ;
#2045=ORIENTED_EDGE ( 'NONE', *, *, #38374, .F. ) ;
#2049=AXIS2_PLACEMENT_3D ( 'NONE', #57784, #26474, #30619 ) ;
#2057=CARTESIAN_POINT ( 'NONE',  ( -6.202661310057998811, -77.14850630154218436, 7.637685261898999656 ) ) ;
#2059=CARTESIAN_POINT ( 'NONE',  ( -10.71369944335147117, -79.62083333333332291, -2.879226727952084453 ) ) ;
#2069=MECHANICAL_DESIGN_GEOMETRIC_PRESENTATION_REPRESENTATION('',(#22777),#23708);
#2074=DIRECTION ( 'NONE',  ( 0.000000000000000000, 1.000000000000000000, 0.000000000000000000 ) ) ;
#2078=CARTESIAN_POINT ( 'NONE',  ( -6.791097082272000485, -77.83441341731199259, -6.981453725808999700 ) ) ;
#2080=CARTESIAN_POINT ( 'NONE',  ( 8.140362823347699006, -77.89063355552166001, -7.514683589434229205 ) ) ;
#2088=CARTESIAN_POINT ( 'NONE',  ( -10.95971813569178188, -80.09360419250441510, 0.9376767887256405309 ) ) ;
#2089=CARTESIAN_POINT ( 'NONE',  ( -5.225954845719999575, -80.00216956313799699, 7.590213850110999694 ) ) ;
#2124=CARTESIAN_POINT ( 'NONE',  ( 9.218103714844254171, -77.35667536906545649, 0.7669798150075999299 ) ) ;
#2125=CARTESIAN_POINT ( 'NONE',  ( 10.71768947918000059, -78.22818662424299418, -1.656903943290000125 ) ) ;
#2132=CARTESIAN_POINT ( 'NONE',  ( -4.306297750730000651, -79.08620252954798957, -10.17515077672999979 ) ) ;
#2138=CARTESIAN_POINT ( 'NONE',  ( -10.81093112166862724, -77.19999999999998863, 1.902172181339564450 ) ) ;
#2147=CARTESIAN_POINT ( 'NONE',  ( 7.038692338534999315, -77.38697173280098696, 6.250440358128999563 ) ) ;
#2158=CARTESIAN_POINT ( 'NONE',  ( -6.405050160242000246, -78.79443481110797620, 8.912875463421000788 ) ) ;
#2161=EDGE_CURVE ( 'NONE', #4986, #1613, #46217, .T. ) ;
#2169=CARTESIAN_POINT ( 'NONE',  ( 11.16390912141999792, -79.41845093841598668, -1.515278025736000123 ) ) ;
#2171=DIRECTION ( 'NONE',  ( 1.000000000000000000, 0.000000000000000000, 0.000000000000000000 ) ) ;
#2177=VERTEX_POINT ( 'NONE', #16317 ) ;
#2179=AXIS2_PLACEMENT_3D ( 'NONE', #21470, #21177, #30603 ) ;
#2181=DIRECTION ( 'NONE',  ( 0.000000000000000000, 0.000000000000000000, -1.000000000000000000 ) ) ;
#2186=CARTESIAN_POINT ( 'NONE',  ( 7.733411907489287529, -79.95018592149614278, -5.588733307671408745 ) ) ;
#2202=CARTESIAN_POINT ( 'NONE',  ( -4.475245744599999576, -78.85670619194497988, -8.610626265545000990 ) ) ;
#2208=EDGE_CURVE ( 'NONE', #30305, #55096, #33018, .T. ) ;
#2211=AXIS2_PLACEMENT_3D ( 'NONE', #47537, #6478, #46952 ) ;
#2215=CARTESIAN_POINT ( 'NONE',  ( 7.000000000000000000, -81.10000000285099020, -1.099999997148999986 ) ) ;
#2218=CARTESIAN_POINT ( 'NONE',  ( 10.78580061008000079, -80.22182239623498390, -2.949165541278000013 ) ) ;
#2226=CARTESIAN_POINT ( 'NONE',  ( 9.223408614079000145, -79.68658117083499803, -2.412288579557000379 ) ) ;
#2233=VECTOR ( 'NONE', #46759, 1000.000000000000000 ) ;
#2235=CARTESIAN_POINT ( 'NONE',  ( 10.67692985166999797, -77.60307432715698894, -2.420308236818999870 ) ) ;
#2238=CARTESIAN_POINT ( 'NONE',  ( -2.117690490098999678, -77.91387044253798422, 9.172054377053999730 ) ) ;
#2241=CARTESIAN_POINT ( 'NONE',  ( 0.000000000000000000, -80.99999999999998579, -7.000000000000000000 ) ) ;
#2262=EDGE_CURVE ( 'NONE', #3901, #1043, #4923, .T. ) ;
#2269=CARTESIAN_POINT ( 'NONE',  ( 0.000000000000000000, -81.99999999999998579, 7.000000000000000000 ) ) ;
#2277=CARTESIAN_POINT ( 'NONE',  ( -7.837416255276716370, -78.64473494204541737, -4.912785058267089333 ) ) ;
#2280=CARTESIAN_POINT ( 'NONE',  ( -3.321932689531000182, -80.44999999999998863, -10.22385755016999909 ) ) ;
#2288=CARTESIAN_POINT ( 'NONE',  ( 6.000000000000000000, -81.19999999999998863, 0.000000000000000000 ) ) ;
#2295=CARTESIAN_POINT ( 'NONE',  ( 10.75486844802039244, -77.71022976309595265, 1.335108088061891074 ) ) ;
#2297=CARTESIAN_POINT ( 'NONE',  ( -3.673218652927999539, -79.25215584929806312, 10.34270183799000087 ) ) ;
#2302=CARTESIAN_POINT ( 'NONE',  ( 8.735034027244228838, -78.32339736695811894, -3.043218161446495706 ) ) ;
#2306=CARTESIAN_POINT ( 'NONE',  ( 9.084121021304000010, -77.60854790367199030, 3.512611703280999809 ) ) ;
#2312=EDGE_CURVE ( 'NONE', #6792, #52990, #25456, .T. ) ;
#2322=CARTESIAN_POINT ( 'NONE',  ( -6.206998376855000110, -77.97811096436200273, 9.469182112634999982 ) ) ;
#2327=CARTESIAN_POINT ( 'NONE',  ( -0.6514213267380000172, -80.13032419407451812, 9.745581310452999801 ) ) ;
#2337=FACE_OUTER_BOUND ( 'NONE', #49503, .T. ) ;
#2345=EDGE_CURVE ( 'NONE', #55096, #24152, #22472, .T. ) ;
#2360=CARTESIAN_POINT ( 'NONE',  ( -6.496683922195000349, -78.20392319598897757, 7.256224481198000120 ) ) ;
#2361=EDGE_CURVE ( 'NONE', #17717, #11974, #17560, .T. ) ;
#2363=CARTESIAN_POINT ( 'NONE',  ( 4.741624722535068948, -77.03333333334457222, 8.228481285277691626 ) ) ;
#2369=CARTESIAN_POINT ( 'NONE',  ( 9.169855720791529663, -79.02165581492216972, 2.557895400793727347 ) ) ;
#2373=CARTESIAN_POINT ( 'NONE',  ( -10.47195525230314139, -80.07542197283444807, 3.366853175460504666 ) ) ;
#2374=CARTESIAN_POINT ( 'NONE',  ( 8.860884805193000702, -78.80704449888298768, -2.531140219154000004 ) ) ;
#2376=CARTESIAN_POINT ( 'NONE',  ( -9.250000000000001776, -79.01041666666667140, -1.210822168571065616 ) ) ;
#2404=ORIENTED_EDGE ( 'NONE', *, *, #30223, .T. ) ;
#2407=CARTESIAN_POINT ( 'NONE',  ( 3.850229173358457491, -77.25920432106504165, -8.419659690126449547 ) ) ;
#2417=CARTESIAN_POINT ( 'NONE',  ( 9.088959790636000236, -78.19661130901299373, -6.010253266999000310 ) ) ;
#2430=CARTESIAN_POINT ( 'NONE',  ( -1.160011803644999784, -78.75834361351799373, -9.451177169703999681 ) ) ;
#2432=EDGE_CURVE ( 'NONE', #9068, #28511, #35808, .T. ) ;
#2443=CARTESIAN_POINT ( 'NONE',  ( -2.169167664939000151, -78.32098300445798600, 10.75912301088999889 ) ) ;
#2451=CARTESIAN_POINT ( 'NONE',  ( 9.009247259181913492, -78.22916666666667140, -2.421167930323368633 ) ) ;
#2453=AXIS2_PLACEMENT_3D ( 'NONE', #33184, #1638, #41479 ) ;
#2454=CARTESIAN_POINT ( 'NONE',  ( -10.13316084080999957, -79.64318977307699754, 4.924182635666999985 ) ) ;
#2457=DIRECTION ( 'NONE',  ( 0.000000000000000000, 0.000000000000000000, -1.000000000000000000 ) ) ;
#2476=CARTESIAN_POINT ( 'NONE',  ( -9.250000000000000000, -79.49999999999998579, 1.813240672189999963E-14 ) ) ;
#2478=ORIENTED_EDGE ( 'NONE', *, *, #43659, .F. ) ;
#2479=CARTESIAN_POINT ( 'NONE',  ( -7.487847511170848236, -77.55006124278669688, 5.430885747604098590 ) ) ;
#2483=CARTESIAN_POINT ( 'NONE',  ( 6.983565664416999219, -78.51907550980999417, -6.737990796766999857 ) ) ;
#2497=CARTESIAN_POINT ( 'NONE',  ( 3.562066907208550237, -79.44390867633869391, 8.599352349090708003 ) ) ;
#2506=DIRECTION ( 'NONE',  ( 0.000000000000000000, 1.000000000000000000, 0.000000000000000000 ) ) ;
#2508=CARTESIAN_POINT ( 'NONE',  ( -8.479436900434727420, -77.15903440364206745, -3.916278883261680388 ) ) ;
#2509=CARTESIAN_POINT ( 'NONE',  ( 7.742394642564000229, -79.65735851257699096, -5.562888445052999842 ) ) ;
#2513=FACE_OUTER_BOUND ( 'NONE', #36211, .T. ) ;
#2514=CARTESIAN_POINT ( 'NONE',  ( -1.439896632895311113, -77.31458333333333144, -11.00000000000000355 ) ) ;
#2515=EDGE_CURVE ( 'NONE', #44715, #45083, #42414, .T. ) ;
#2517=CARTESIAN_POINT ( 'NONE',  ( -9.137594394056998581, -77.91723112247599659, -6.029850034859999930 ) ) ;
#2523=CARTESIAN_POINT ( 'NONE',  ( -0.8405563561534999950, -76.88792425275799758, -9.635375415708001157 ) ) ;
#2533=ORIENTED_EDGE ( 'NONE', *, *, #10356, .T. ) ;
#2535=VERTEX_POINT ( 'NONE', #33649 ) ;
#2557=CARTESIAN_POINT ( 'NONE',  ( -5.173679449032695388, -79.93013575167898921, -8.224241350002412076 ) ) ;
#2560=CARTESIAN_POINT ( 'NONE',  ( -7.779924306592839400, -78.64565599839535537, -5.003626092249043644 ) ) ;
#2568=CARTESIAN_POINT ( 'NONE',  ( -11.00000000000000000, -74.64999999999999147, 0.000000000000000000 ) ) ;
#2579=CARTESIAN_POINT ( 'NONE',  ( -0.3888001762888235735, -77.57257727438346251, -10.76536887735824877 ) ) ;
#2580=CARTESIAN_POINT ( 'NONE',  ( 1.179538764136264906, -78.23344348886517707, -11.01565543437853734 ) ) ;
#2593=CARTESIAN_POINT ( 'NONE',  ( -9.520207861471000399, -78.95852403778498285, -0.1897854149113999966 ) ) ;
#2599=CARTESIAN_POINT ( 'NONE',  ( 10.69999999999999929, -81.79999999999998295, 0.000000000000000000 ) ) ;
#2600=CARTESIAN_POINT ( 'NONE',  ( -7.000000000000000000, -81.19999999999998863, 0.000000000000000000 ) ) ;
#2603=CARTESIAN_POINT ( 'NONE',  ( 0.1299632413661999941, -79.18100181365798562, 11.04812215732000169 ) ) ;
#2609=CARTESIAN_POINT ( 'NONE',  ( -4.690256031270999770, -77.64794858637398534, -10.30503454587000078 ) ) ;
#2610=ORIENTED_EDGE ( 'NONE', *, *, #23773, .F. ) ;
#2614=CARTESIAN_POINT ( 'NONE',  ( -9.358268528169000788, -79.53341926633650871, -2.797054701638000296 ) ) ;
#2635=B_SPLINE_CURVE_WITH_KNOTS ( 'NONE', 3,
 ( #33452, #42620, #51489, #11047, #38468, #2186, #38177, #56198, #15745, #33742, #11330, #47357, #6886, #21613, #57342, #13033, #40499, #17774, #57627, #26036, #12465, #53202, #26905, #30465, #8915, #48496, #39903, #39335, #25758, #18070, #44061, #44933, #44639, #48781, #35764, #58212, #31322, #3608, #39619, #35169, #22488, #17475, #48222, #49365 ),
 .UNSPECIFIED., .F., .F.,
 ( 4, 2, 2, 2, 2, 2, 2, 2, 2, 2, 2, 2, 2, 2, 2, 2, 2, 2, 2, 2, 2, 4 ),
 ( 1.714264432196704922E-08, 0.03125001607122906977, 0.06250001499981379383, 0.09375001392839851788, 0.1250000128569832558, 0.1562500117855679937, 0.1875000107141527039, 0.2187500096427374141, 0.2500000085713221520, 0.2812500074999068067, 0.3125000064284915724, 0.3281250058927839830, 0.3437500053570763381, 0.3593750048213686932, 0.3750000042856610483, 0.3906250037499534589, 0.4062500032142458140, 0.4218750026785381690, 0.4375000021428305241, 0.4687500010714153453, 0.4843750005357077004, 0.5000000000000000000 ),
 .UNSPECIFIED. ) ;
#2649=CARTESIAN_POINT ( 'NONE',  ( -3.921497456393000292, -77.86283724644100346, -8.915242756422999904 ) ) ;
#2657=CARTESIAN_POINT ( 'NONE',  ( 0.5334414343224818111, -79.12052801969377924, 9.504702743072071414 ) ) ;
#2662=CARTESIAN_POINT ( 'NONE',  ( -1.274026893842000074, -79.96482190487999731, 9.474508900323998617 ) ) ;
#2679=CARTESIAN_POINT ( 'NONE',  ( -4.465297566879000257, -79.62232954496899140, 8.686876450551999085 ) ) ;
#2688=CARTESIAN_POINT ( 'NONE',  ( -2.879226727952121312, -77.59583333333331723, 10.71369944335146052 ) ) ;
#2693=DIRECTION ( 'NONE',  ( 0.000000000000000000, 1.000000000000000000, 0.000000000000000000 ) ) ;
#2700=CARTESIAN_POINT ( 'NONE',  ( 3.557252205646057597, -77.25651624396304840, -8.541931941478511092 ) ) ;
#2704=EDGE_CURVE ( 'NONE', #10810, #35609, #51353, .T. ) ;
#2705=FACE_OUTER_BOUND ( 'NONE', #2996, .T. ) ;
#2709=CARTESIAN_POINT ( 'NONE',  ( -3.697742159549999741, -79.39521842720699851, 10.41175280961999938 ) ) ;
#2722=CARTESIAN_POINT ( 'NONE',  ( 2.813750093493999849, -77.79193342313199366, -9.096877851405000825 ) ) ;
#2732=CARTESIAN_POINT ( 'NONE',  ( -10.79326785783000098, -79.38437425209399123, -1.992331681952000055 ) ) ;
#2740=DIRECTION ( 'NONE',  ( 0.000000000000000000, 1.000000000000000000, 0.000000000000000000 ) ) ;
#2741=CARTESIAN_POINT ( 'NONE',  ( 10.45148855949000044, -78.02152425389999735, 3.906137931512999817 ) ) ;
#2764=CARTESIAN_POINT ( 'NONE',  ( -1.769489979047951467, -78.20976201800445438, -9.079134725190300514 ) ) ;
#2768=CARTESIAN_POINT ( 'NONE',  ( -3.474029939969885739, -77.50579965437593444, 8.573561196712942589 ) ) ;
#2771=CARTESIAN_POINT ( 'NONE',  ( 3.248345031021000029, -78.17798956026199164, 9.144340540792999406 ) ) ;
#2774=CARTESIAN_POINT ( 'NONE',  ( 10.52776997023000050, -80.08830587811999635, 3.979665013433000720 ) ) ;
#2782=CARTESIAN_POINT ( 'NONE',  ( -1.210889911462935231, -78.48544186924020494, 9.249751145355588733 ) ) ;
#2785=CARTESIAN_POINT ( 'NONE',  ( 4.535769924631999572, -80.15130006555698117, -10.22046309969000077 ) ) ;
#2792=ADVANCED_FACE ( 'NONE', ( #12523 ), #11625, .F. ) ;
#2794=CARTESIAN_POINT ( 'NONE',  ( -8.024068383896736378, -77.16415510318682891, -4.770143147090037949 ) ) ;
#2796=B_SPLINE_CURVE_WITH_KNOTS ( 'NONE', 3,
 ( #22569, #49745, #9286, #40581, #8694, #50033, #26685, #58292, #17855, #27276, #35844, #45313, #5150, #55614, #51492, #20188, #45899, #24610, #37012 ),
 .UNSPECIFIED., .F., .F.,
 ( 4, 1, 1, 1, 1, 1, 1, 1, 1, 1, 1, 1, 1, 1, 1, 1, 4 ),
 ( 0.000000000000000000, 0.04500074405000878408, 0.1100006377635261434, 0.1750005314770704257, 0.2400004251906146802, 0.3050003189042128082, 0.3700002126177032169, 0.4350001063311936811, 0.5000000000446841453, 0.5649998937584436165, 0.6299997874719340807, 0.6949996811854246559, 0.7599995748989150091, 0.8249994686124054732, 0.8899993623258959374, 0.9549992560396556307, 1.000000000000000000 ),
 .UNSPECIFIED. ) ;
#2797=CARTESIAN_POINT ( 'NONE',  ( 9.328744840303000885, -79.62270543005199386, -2.439838196641999524 ) ) ;
#2800=CARTESIAN_POINT ( 'NONE',  ( -8.874863966699559015, -79.31646010331650132, 3.954991475770741172 ) ) ;
#2803=AXIS2_PLACEMENT_3D ( 'NONE', #36723, #54737, #54161 ) ;
#2806=CARTESIAN_POINT ( 'NONE',  ( -0.9683059680012998660, -77.42495975171298994, -11.01410536002000029 ) ) ;
#2813=CARTESIAN_POINT ( 'NONE',  ( -9.611650271896857944, -77.55833333333332291, 5.539808784079855997 ) ) ;
#2823=ORIENTED_EDGE ( 'NONE', *, *, #41511, .T. ) ;
#2832=VERTEX_POINT ( 'NONE', #26664 ) ;
#2835=AXIS2_PLACEMENT_3D ( 'NONE', #55220, #42238, #28637 ) ;
#2838=CIRCLE ( 'NONE', #47153, 2.799999999999999822 ) ;
#2843=CARTESIAN_POINT ( 'NONE',  ( 11.00000000000000000, -78.44999999999998863, 0.000000000000000000 ) ) ;
#2848=CARTESIAN_POINT ( 'NONE',  ( -10.90550475849158119, -80.11063224077452105, -1.438076737588118048 ) ) ;
#2868=ORIENTED_EDGE ( 'NONE', *, *, #53910, .F. ) ;
#2874=CARTESIAN_POINT ( 'NONE',  ( 8.381176496771999496, -78.18405256877699117, 4.744374615790000860 ) ) ;
#2876=DIRECTION ( 'NONE',  ( 0.000000000000000000, -1.000000000000000000, 0.000000000000000000 ) ) ;
#2885=CARTESIAN_POINT ( 'NONE',  ( 9.274475910318999539, -79.07632342844499362, -5.802750462065000114 ) ) ;
#2887=CARTESIAN_POINT ( 'NONE',  ( -10.56934456194000127, -80.33626512904898220, -4.081628045126000082 ) ) ;
#2893=CARTESIAN_POINT ( 'NONE',  ( -9.699833017908000343, -79.62079945152900962, 1.146274062705999963 ) ) ;
#2903=EDGE_CURVE ( 'NONE', #17089, #55354, #15444, .T. ) ;
#2912=CARTESIAN_POINT ( 'NONE',  ( 2.166634614239063377E-07, -77.01246206852036380, -9.437473063691797392 ) ) ;
#2920=CARTESIAN_POINT ( 'NONE',  ( 5.114889623276000385, -77.12723231992129058, -7.994241842339000037 ) ) ;
#2921=DIRECTION ( 'NONE',  ( 0.000000000000000000, 0.000000000000000000, -1.000000000000000000 ) ) ;
#2925=CARTESIAN_POINT ( 'NONE',  ( -1.966850719965000494, -77.37963215124798921, -9.538930191946999315 ) ) ;
#2930=ORIENTED_EDGE ( 'NONE', *, *, #10786, .F. ) ;
#2933=CARTESIAN_POINT ( 'NONE',  ( -0.7090885217563500653, -79.13093592298157830, 9.493073439722991225 ) ) ;
#2934=B_SPLINE_CURVE_WITH_KNOTS ( 'NONE', 3,
 ( #13704, #26114, #3969, #35246 ),
 .UNSPECIFIED., .F., .F.,
 ( 4, 4 ),
 ( 0.000000000000000000, 1.000000000000000000 ),
 .UNSPECIFIED. ) ;
#2936=CARTESIAN_POINT ( 'NONE',  ( -4.889775958634938746, -79.99999999999998579, -8.013494230838169585 ) ) ;
#2939=CARTESIAN_POINT ( 'NONE',  ( -4.561872603918999403, -79.85766786116599292, -8.776383598921000839 ) ) ;
#2940=DIRECTION ( 'NONE',  ( 0.000000000000000000, 1.000000000000000000, 0.000000000000000000 ) ) ;
#2941=CARTESIAN_POINT ( 'NONE',  ( -9.611650271896833075, -78.64166666666667993, -5.539808784079895077 ) ) ;
#2958=CARTESIAN_POINT ( 'NONE',  ( -8.448510849392999233, -79.16771232935798253, 4.901364000006999788 ) ) ;
#2965=DIRECTION ( 'NONE',  ( 9.386928511358000402E-11, -1.000000000000000000, -5.363054260619999949E-10 ) ) ;
#2969=FACE_OUTER_BOUND ( 'NONE', #53859, .T. ) ;
#2973=CARTESIAN_POINT ( 'NONE',  ( -1.180921238786448946, -79.98531230651158808, 9.176345860435365154 ) ) ;
#2978=CARTESIAN_POINT ( 'NONE',  ( 10.99934742197999960, -79.88817051509798262, 2.437886521773999782 ) ) ;
#2979=ADVANCED_FACE ( 'NONE', ( #42608, #27837 ), #24000, .F. ) ;
#2980=CARTESIAN_POINT ( 'NONE',  ( 7.560074365901553683, -77.30122887067066983, -5.329858952455061250 ) ) ;
#2987=DIRECTION ( 'NONE',  ( 1.000000000000000000, 0.000000000000000000, 0.000000000000000000 ) ) ;
#2990=CARTESIAN_POINT ( 'NONE',  ( -10.61618518222999796, -78.53204647501199531, 3.433396544298999764 ) ) ;
#2996=EDGE_LOOP ( 'NONE', ( #7749, #43806, #51269, #17557 ) ) ;
#3007=CARTESIAN_POINT ( 'NONE',  ( 9.412698430168999764, -77.33012407454400261, 0.1109178415545999941 ) ) ;
#3017=CARTESIAN_POINT ( 'NONE',  ( -10.57157196544999955, -79.85258015763899664, 2.324769239444999691 ) ) ;
#3028=B_SPLINE_CURVE_WITH_KNOTS ( 'NONE', 3,
 ( #36962, #32810, #19545, #32517, #55560, #1851, #2138, #50561, #55859, #10402, #51442, #15109, #33105, #51149, #10704, #28681, #15411, #6252, #10994, #28977, #47019, #38419, #38709, #17141, #29836, #7130, #56438, #16861, #11859, #25131, #39576, #21280, #7993, #34268, #47606, #57299, #34842, #56729, #11571, #57579, #7419, #15992, #47308, #52872, #29551, #25991 ),
 .UNSPECIFIED., .F., .F.,
 ( 4, 1, 1, 1, 1, 1, 2, 2, 1, 1, 1, 1, 1, 1, 2, 2, 1, 1, 1, 1, 2, 2, 1, 2, 2, 2, 2, 2, 2, 2, 4 ),
 ( 0.000000000000000000, 0.06249999999999175659, 0.09374999999998766265, 0.1093749999999855810, 0.1171874999999845679, 0.1210937499999840405, 0.1230468749999838324, 0.1249999999999835965, 0.1874999999999750477, 0.2187499999999706901, 0.2343749999999685807, 0.2421874999999675815, 0.2460937499999671374, 0.2480468749999668876, 0.2490234374999668598, 0.2499999999999668043, 0.3124999999999651945, 0.3437499999999644729, 0.3593749999999639733, 0.3671874999999638067, 0.3710937499999638067, 0.3749999999999638622, 0.4374999999999673594, 0.4687499999999691913, 0.4999999999999710232, 0.6249999999999783507, 0.6874999999999820144, 0.7499999999999856781, 0.8124999999999893419, 0.8749999999999928946, 1.000000000000000000 ),
 .UNSPECIFIED. ) ;
#3029=CARTESIAN_POINT ( 'NONE',  ( -11.19646453606000058, -78.68804972576597834, -1.252244488204000028 ) ) ;
#3032=DIRECTION ( 'NONE',  ( 1.000000000000000000, 0.000000000000000000, 0.000000000000000000 ) ) ;
#3055=VERTEX_POINT ( 'NONE', #8024 ) ;
#3057=CARTESIAN_POINT ( 'NONE',  ( -6.737926365805661177, -77.54008088401030818, 6.337568593985769994 ) ) ;
#3058=CARTESIAN_POINT ( 'NONE',  ( 1.160587285869999929, -77.67616457946799358, 10.97894289003999901 ) ) ;
#3060=CARTESIAN_POINT ( 'NONE',  ( -9.139898499914998808, -77.24602254130299173, 2.826942883852999966 ) ) ;
#3061=CARTESIAN_POINT ( 'NONE',  ( -1.000000000000000000, -81.19999999999998863, -7.000000000000000000 ) ) ;
#3064=CARTESIAN_POINT ( 'NONE',  ( -8.254612054926999676, -79.87482240675299749, 6.886499823760000361 ) ) ;
#3077=CARTESIAN_POINT ( 'NONE',  ( 5.389383425300000141, -80.26373015146698719, 9.671489469558000707 ) ) ;
#3087=CARTESIAN_POINT ( 'NONE',  ( 9.002331482469001500, -79.25367172123299042, -1.969766031707999909 ) ) ;
#3097=CARTESIAN_POINT ( 'NONE',  ( -10.93544969797999933, -77.37459665783399032, -0.5202540992781999885 ) ) ;
#3122=ORIENTED_EDGE ( 'NONE', *, *, #51295, .F. ) ;
#3139=AXIS2_PLACEMENT_3D ( 'NONE', #27654, #5235, #1408 ) ;
#3158=LINE ( 'NONE', #30285, #23867 ) ;
#3168=CARTESIAN_POINT ( 'NONE',  ( 8.731705537153999330, -78.67428574649498785, -3.798380529179000042 ) ) ;
#3174=CARTESIAN_POINT ( 'NONE',  ( 5.628103047462848174, -78.92394918533045711, 7.438029003534223804 ) ) ;
#3178=CARTESIAN_POINT ( 'NONE',  ( -4.428614322242999890, -79.71475654597799121, 10.12250943391000035 ) ) ;
#3181=CARTESIAN_POINT ( 'NONE',  ( 7.235133928286000327, -80.06358356157298317, 8.863387837910000400 ) ) ;
#3190=CARTESIAN_POINT ( 'NONE',  ( -4.373213035511999358, -79.71821742630301344, -8.733596771889999388 ) ) ;
#3198=DIRECTION ( 'NONE',  ( 0.000000000000000000, 1.000000000000000000, 0.000000000000000000 ) ) ;
#3202=CARTESIAN_POINT ( 'NONE',  ( 8.582624075744034187, -78.81972267989517889, -3.449750442334098555 ) ) ;
#3208=DIRECTION ( 'NONE',  ( 0.000000000000000000, 0.000000000000000000, -1.000000000000000000 ) ) ;
#3211=CARTESIAN_POINT ( 'NONE',  ( 4.299999999999999822, -74.99999999999998579, 0.000000000000000000 ) ) ;
#3215=CARTESIAN_POINT ( 'NONE',  ( 2.583569908777999746, -77.30999788869900158, 9.132097282893997914 ) ) ;
#3216=LINE ( 'NONE', #11785, #35157 ) ;
#3229=CARTESIAN_POINT ( 'NONE',  ( -9.499162930933517046, -79.25065129256583418, -0.07774627389065781602 ) ) ;
#3230=CARTESIAN_POINT ( 'NONE',  ( -6.855033324489887114, -79.99999999999998579, -6.359874399135010847 ) ) ;
#3233=CARTESIAN_POINT ( 'NONE',  ( 8.763152011282000942, -79.42031553780299191, -4.343982967351999847 ) ) ;
#3235=CARTESIAN_POINT ( 'NONE',  ( 9.250000000000001776, -79.23958333333332860, -1.210822168571047186 ) ) ;
#3246=CARTESIAN_POINT ( 'NONE',  ( 0.3759584291129999811, -77.55688181347299803, -11.09523831386000126 ) ) ;
#3252=CARTESIAN_POINT ( 'NONE',  ( 3.269429986698999979, -79.55738422845298885, 9.203886808668999109 ) ) ;
#3255=VERTEX_POINT ( 'NONE', #8313 ) ;
#3260=CARTESIAN_POINT ( 'NONE',  ( 6.760013919724038978, -77.52291666666664582, 8.796335266380001627 ) ) ;
#3267=CARTESIAN_POINT ( 'NONE',  ( 1.443912542026016155, -79.96302067931829072, 9.136300447085167420 ) ) ;
#3269=CARTESIAN_POINT ( 'NONE',  ( -10.82575263932852572, -79.93590035623954293, 1.999893313492130620 ) ) ;
#3271=CARTESIAN_POINT ( 'NONE',  ( 7.994753734545000157, -78.93303046778699184, 7.938063182512999916 ) ) ;
#3272=CARTESIAN_POINT ( 'NONE',  ( 7.757711236729307736, -77.30428715488800151, -5.039461175929132786 ) ) ;
#3278=CARTESIAN_POINT ( 'NONE',  ( 10.71369944335146762, -78.37083333333333712, 2.879226727952103548 ) ) ;
#3281=CARTESIAN_POINT ( 'NONE',  ( 10.14733453800999996, -78.84106237267099004, 4.639310447764000145 ) ) ;
#3285=DIRECTION ( 'NONE',  ( 0.000000000000000000, -1.000000000000000000, 0.000000000000000000 ) ) ;
#3296=CARTESIAN_POINT ( 'NONE',  ( 7.742244746672000133, -78.84361510090498371, -5.543281135378999913 ) ) ;
#3306=CARTESIAN_POINT ( 'NONE',  ( 10.31626776183999894, -78.15242887846198983, -3.746764721243999841 ) ) ;
#3314=CARTESIAN_POINT ( 'NONE',  ( -5.684557159767971157, -78.07291666666667140, -7.396918292183161547 ) ) ;
#3315=CARTESIAN_POINT ( 'NONE',  ( -10.61618518222999796, -78.21817073422899114, 3.433396544298999764 ) ) ;
#3327=ORIENTED_EDGE ( 'NONE', *, *, #33623, .T. ) ;
#3340=CARTESIAN_POINT ( 'NONE',  ( -5.503123143393462868, -77.52574563389143236, 7.434945069734956391 ) ) ;
#3341=CARTESIAN_POINT ( 'NONE',  ( -5.876696946710000091, -77.45018012715098621, -9.346046374399000101 ) ) ;
#3344=CARTESIAN_POINT ( 'NONE',  ( -9.669247687117000112, -77.83690361071398911, -0.8224101967608999919 ) ) ;
#3348=CARTESIAN_POINT ( 'NONE',  ( -10.55592303174000079, -79.95834473742999648, -3.904632140253000205 ) ) ;
#3350=FACE_OUTER_BOUND ( 'NONE', #46619, .T. ) ;
#3356=CARTESIAN_POINT ( 'NONE',  ( -5.684148906237979304, -78.52710219421626903, 7.396423488596521878 ) ) ;
#3359=CARTESIAN_POINT ( 'NONE',  ( -0.2870568347697000089, -80.17991464100198584, -11.28808005806000025 ) ) ;
#3372=CARTESIAN_POINT ( 'NONE',  ( 9.243445784771999740, -79.26341260731899752, -0.8678123785519999966 ) ) ;
#3375=CARTESIAN_POINT ( 'NONE',  ( 7.803382786781845049, -77.28749999999999432, -7.800872125332472429 ) ) ;
#3386=CARTESIAN_POINT ( 'NONE',  ( -0.8405563561534999950, -76.82762132708718639, -9.635375415708001157 ) ) ;
#3410=ORIENTED_EDGE ( 'NONE', *, *, #33798, .F. ) ;
#3416=EDGE_CURVE ( 'NONE', #34022, #43554, #16610, .T. ) ;
#3418=FACE_BOUND ( 'NONE', #15827, .T. ) ;
#3423=CARTESIAN_POINT ( 'NONE',  ( -9.122985626357428046, -78.61336444762311260, -1.527181035531375297 ) ) ;
#3425=CARTESIAN_POINT ( 'NONE',  ( -10.30336598198321951, -80.12884657563031965, -3.851716267939166549 ) ) ;
#3445=CARTESIAN_POINT ( 'NONE',  ( -8.527407416480999203, -78.35459554355099954, 4.476218573567000369 ) ) ;
#3450=AXIS2_PLACEMENT_3D ( 'NONE', #57488, #3198, #29175 ) ;
#3451=CARTESIAN_POINT ( 'NONE',  ( -11.00000000000000000, -78.71041666666667425, -1.439896632895320217 ) ) ;
#3455=CARTESIAN_POINT ( 'NONE',  ( -6.384381598444999639, -78.79539988511800175, 8.884114358872000849 ) ) ;
#3457=FACE_OUTER_BOUND ( 'NONE', #8183, .T. ) ;
#3459=ORIENTED_EDGE ( 'NONE', *, *, #1178, .F. ) ;
#3465=CARTESIAN_POINT ( 'NONE',  ( -0.5483576180056000116, -79.87054292801151689, -9.751923335751000010 ) ) ;
#3468=ORIENTED_EDGE ( 'NONE', *, *, #12887, .F. ) ;
#3493=CARTESIAN_POINT ( 'NONE',  ( -0.4970193761121000087, -77.33610725566698818, 9.477499788518001012 ) ) ;
#3508=CARTESIAN_POINT ( 'NONE',  ( 8.495067938628560356, -79.03726686963507575, 4.296429619035287750 ) ) ;
#3511=CARTESIAN_POINT ( 'NONE',  ( -6.760013919724099374, -79.02708333333332291, 8.796335266379958995 ) ) ;
#3513=CARTESIAN_POINT ( 'NONE',  ( -7.959955112152999668, -79.09500618921398996, 5.491262329125000008 ) ) ;
#3523=ORIENTED_EDGE ( 'NONE', *, *, #28250, .F. ) ;
#3530=CARTESIAN_POINT ( 'NONE',  ( -9.358268528169000788, -79.35326349721498218, -2.797054701638000296 ) ) ;
#3547=CARTESIAN_POINT ( 'NONE',  ( 1.444432371921226865, -79.96301603591265916, 9.136218687011998796 ) ) ;
#3548=CARTESIAN_POINT ( 'NONE',  ( -9.813001901106970237, -79.91600936110660314, 4.522963347059401507 ) ) ;
#3550=CARTESIAN_POINT ( 'NONE',  ( -9.332307860560000279, -79.07349223945099936, 6.311653060910999535 ) ) ;
#3551=CARTESIAN_POINT ( 'NONE',  ( 5.130170376780485597, -77.27182112023126592, -7.706256298038600683 ) ) ;
#3554=DIRECTION ( 'NONE',  ( -1.000000000000000000, 0.000000000000000000, 0.000000000000000000 ) ) ;
#3560=CARTESIAN_POINT ( 'NONE',  ( 4.105747930350998942, -79.71192535698398274, -10.37470161445000016 ) ) ;
#3561=EDGE_CURVE ( 'NONE', #38384, #40940, #53340, .T. ) ;
#3564=CARTESIAN_POINT ( 'NONE',  ( 0.000000000000000000, -74.64999999999999147, 0.000000000000000000 ) ) ;
#3575=CARTESIAN_POINT ( 'NONE',  ( 5.376158796547000129, -78.87906701255899122, -7.990628517496999983 ) ) ;
#3585=CARTESIAN_POINT ( 'NONE',  ( 9.694840914897000062, -79.64132365809399516, -5.145296513660000848 ) ) ;
#3593=CARTESIAN_POINT ( 'NONE',  ( 5.539808784079905735, -77.76666666666665151, -9.611650271896829523 ) ) ;
#3594=CARTESIAN_POINT ( 'NONE',  ( 9.791822688510999129, -79.03284900987598860, 5.349000663092000174 ) ) ;
#3596=CARTESIAN_POINT ( 'NONE',  ( 10.69999999999999929, -77.19999999999998863, 0.000000000000000000 ) ) ;
#3608=CARTESIAN_POINT ( 'NONE',  ( 6.152927464707564020, -79.56974109780976789, 7.410766869306328886 ) ) ;
#3614=CARTESIAN_POINT ( 'NONE',  ( -6.538910319532891258, -78.16269370453200338, -6.542411771513464203 ) ) ;
#3619=CARTESIAN_POINT ( 'NONE',  ( -5.441782793747363733, -77.52508094701889263, 7.479905722084790654 ) ) ;
#3620=CARTESIAN_POINT ( 'NONE',  ( 10.77519778174000109, -77.05057364238318485, -1.228540277667999892 ) ) ;
#3622=CARTESIAN_POINT ( 'NONE',  ( 9.662203867310999783, -79.08755209238998418, 0.9012207007054000574 ) ) ;
#3628=CARTESIAN_POINT ( 'NONE',  ( -11.09141466634999951, -79.85628064642098423, 1.909950515085000022 ) ) ;
#3632=CARTESIAN_POINT ( 'NONE',  ( -8.082524092276882399, -78.54166666666665719, -4.658475568430820779 ) ) ;
#3646=CARTESIAN_POINT ( 'NONE',  ( -6.760013919724102038, -80.12708333335245925, 8.796335266379953666 ) ) ;
#3653=CARTESIAN_POINT ( 'NONE',  ( 4.297451186800683942, -78.10789250826600494, -9.948289673926124621 ) ) ;
#3654=CARTESIAN_POINT ( 'NONE',  ( -7.313922093392000612, -79.57512096206998820, -5.944137246278000219 ) ) ;
#3663=B_SPLINE_CURVE_WITH_KNOTS ( 'NONE', 3,
 ( #11805, #3235, #52817, #16808, #29779, #42523, #47555, #52248, #42812, #24507, #25366, #21226, #43382, #43106, #51966, #30069, #2376, #7366 ),
 .UNSPECIFIED., .F., .F.,
 ( 4, 2, 2, 2, 2, 2, 2, 2, 4 ),
 ( 0.000000000000000000, 0.1250000000000000278, 0.2500000000000000555, 0.3750000000000001665, 0.5000000000000001110, 0.6250000000000001110, 0.7500000000000002220, 0.8750000000000001110, 1.000000000000000000 ),
 .UNSPECIFIED. ) ;
#3664=B_SPLINE_CURVE_WITH_KNOTS ( 'NONE', 3,
 ( #5749, #33183, #15777, #29057, #24352, #23757, #10781, #41770, #1346, #19339, #34343, #11650, #2497, #21354, #16363, #29627, #44092, #25786, #12498, #38785, #52092 ),
 .UNSPECIFIED., .F., .F.,
 ( 4, 2, 2, 2, 2, 2, 1, 2, 2, 2, 4 ),
 ( 0.000000000000000000, 0.1249999999999999167, 0.2499999999999998335, 0.3749999999999997780, 0.4999999999999996669, 0.5624999999999996669, 0.6249999999999995559, 0.6874999999999996669, 0.7499999999999996669, 0.8749999999999998890, 1.000000000000000000 ),
 .UNSPECIFIED. ) ;
#3678=ORIENTED_EDGE ( 'NONE', *, *, #787, .T. ) ;
#3680=ORIENTED_EDGE ( 'NONE', *, *, #26432, .F. ) ;
#3689=CARTESIAN_POINT ( 'NONE',  ( 10.22358047590571317, -78.07468344508760083, -3.366618272953084468 ) ) ;
#3704=CARTESIAN_POINT ( 'NONE',  ( -8.329046064005918737, -78.63589279464400761, -4.024567744346438936 ) ) ;
#3705=ADVANCED_FACE ( 'NONE', ( #39815 ), #12666, .F. ) ;
#3706=AXIS2_PLACEMENT_3D ( 'NONE', #9262, #26954, #35817 ) ;
#3710=CIRCLE ( 'NONE', #17882, 10.69999999999999929 ) ;
#3717=CARTESIAN_POINT ( 'NONE',  ( 11.00000000000000711, -79.43958333333333144, -1.439896632895300010 ) ) ;
#3730=CARTESIAN_POINT ( 'NONE',  ( 10.50000000000000000, -81.99999999999998579, 0.000000000000000000 ) ) ;
#3731=CARTESIAN_POINT ( 'NONE',  ( 6.193386186315999353, -78.21247639790598782, 7.375308638433999420 ) ) ;
#3736=LINE ( 'NONE', #52187, #48479 ) ;
#3737=CARTESIAN_POINT ( 'NONE',  ( -6.983600593180121052, -79.04328884231583174, 6.095355805603315247 ) ) ;
#3742=CARTESIAN_POINT ( 'NONE',  ( 10.70874647057999951, -79.10441578277699648, -2.238429218213000116 ) ) ;
#3744=DIRECTION ( 'NONE',  ( 0.000000000000000000, 1.000000000000000000, 0.000000000000000000 ) ) ;
#3747=ORIENTED_EDGE ( 'NONE', *, *, #22853, .F. ) ;
#3753=CARTESIAN_POINT ( 'NONE',  ( 9.630577183392999174, -79.51334368717353129, 1.628483183780000010 ) ) ;
#3761=CARTESIAN_POINT ( 'NONE',  ( 9.499178638196321245, -79.00092112126561972, 0.1004274591880019996 ) ) ;
#3764=CARTESIAN_POINT ( 'NONE',  ( 4.100000000000000533, -81.79999999999998295, 0.000000000000000000 ) ) ;
#3766=CARTESIAN_POINT ( 'NONE',  ( 0.000000000000000000, -81.19999999999998863, 7.000000000000000000 ) ) ;
#3775=CARTESIAN_POINT ( 'NONE',  ( -2.826502466506999767, -77.05760734133949086, -8.941232880334000654 ) ) ;
#3786=CARTESIAN_POINT ( 'NONE',  ( 8.000000000000000000, -81.19999999999998863, 0.000000000000000000 ) ) ;
#3796=CARTESIAN_POINT ( 'NONE',  ( -0.2732314027492999675, -79.02031087269799059, 9.666450061188999854 ) ) ;
#3800=DIRECTION ( 'NONE',  ( 0.000000000000000000, -1.000000000000000000, 0.000000000000000000 ) ) ;
#3817=CARTESIAN_POINT ( 'NONE',  ( -2.217000330786000450, -79.16306993851199536, 9.512392227823999846 ) ) ;
#3819=VERTEX_POINT ( 'NONE', #57450 ) ;
#3826=CARTESIAN_POINT ( 'NONE',  ( -9.669407782331445489, -77.85665777210621741, -0.8224238135324427601 ) ) ;
#3835=CARTESIAN_POINT ( 'NONE',  ( 3.242578276031594875, -79.94660715946710638, 8.663862471309647262 ) ) ;
#3837=ORIENTED_EDGE ( 'NONE', *, *, #36437, .T. ) ;
#3838=CARTESIAN_POINT ( 'NONE',  ( -10.40633193566000081, -78.65210692446099472, -4.317081191017999586 ) ) ;
#3844=DIRECTION ( 'NONE',  ( 0.000000000000000000, -0.7071067811866525998, -0.7071067811864425456 ) ) ;
#3846=CARTESIAN_POINT ( 'NONE',  ( -8.192247052095000370, -78.61632353800997919, -7.574872137178000564 ) ) ;
#3847=DIRECTION ( 'NONE',  ( 0.000000000000000000, 1.000000000000000000, 0.000000000000000000 ) ) ;
#3861=CARTESIAN_POINT ( 'NONE',  ( 8.977320902561999105, -78.98328771936498072, 3.091814932086999868 ) ) ;
#3871=CARTESIAN_POINT ( 'NONE',  ( -4.277738290159001089, -79.02329186277498252, -10.10766895494000117 ) ) ;
#3879=CARTESIAN_POINT ( 'NONE',  ( -2.868749083076024498, -77.39991823718625596, 8.824073868535768028 ) ) ;
#3880=CARTESIAN_POINT ( 'NONE',  ( 9.611650271896847286, -77.80833333333332291, -5.539808784079878201 ) ) ;
#3881=CARTESIAN_POINT ( 'NONE',  ( -11.03994916103999913, -78.31013882934497872, -0.4443153950920000206 ) ) ;
#3888=EDGE_LOOP ( 'NONE', ( #26253, #33918, #22380, #11114, #9128, #48558, #52479 ) ) ;
#3897=CARTESIAN_POINT ( 'NONE',  ( -3.528673621653970471, -78.19399569326179744, -8.550395938606023094 ) ) ;
#3901=VERTEX_POINT ( 'NONE', #47749 ) ;
#3903=CARTESIAN_POINT ( 'NONE',  ( 1.394768719700775872, -77.46297058018842563, 9.144265183523252460 ) ) ;
#3905=CARTESIAN_POINT ( 'NONE',  ( -1.996894868142000012, -77.19901894948809229, 10.85801781015000067 ) ) ;
#3907=CIRCLE ( 'NONE', #45448, 4.299999999999999822 ) ;
#3908=CARTESIAN_POINT ( 'NONE',  ( -7.843978203195000276, -77.84035887812699173, 5.713380375430999969 ) ) ;
#3912=CARTESIAN_POINT ( 'NONE',  ( -10.55592303174000079, -79.83773888608898517, -3.904632140253000205 ) ) ;
#3916=EDGE_LOOP ( 'NONE', ( #20829, #55857, #38689, #5037, #28740, #25102 ) ) ;
#3920=EDGE_CURVE ( 'NONE', #54465, #20866, #4378, .T. ) ;
#3925=CARTESIAN_POINT ( 'NONE',  ( -10.86942385660000099, -80.59640203517098200, 3.442886605850000059 ) ) ;
#3930=ORIENTED_EDGE ( 'NONE', *, *, #44181, .T. ) ;
#3936=CARTESIAN_POINT ( 'NONE',  ( -0.4701581901367999916, -79.39978501252298315, 9.413031935884999868 ) ) ;
#3938=CARTESIAN_POINT ( 'NONE',  ( 10.19329140123695154, -77.31875000000002274, -4.224121120694948495 ) ) ;
#3948=CARTESIAN_POINT ( 'NONE',  ( -2.880544446985999762, -76.99112385945399240, -9.112186890989001142 ) ) ;
#3950=CIRCLE ( 'NONE', #26562, 5.000000000000000000 ) ;
#3956=DIRECTION ( 'NONE',  ( 0.000000000000000000, -1.000000000000000000, 0.000000000000000000 ) ) ;
#3961=VERTEX_POINT ( 'NONE', #40013 ) ;
#3966=PRESENTATION_STYLE_ASSIGNMENT (( #45008 ) ) ;
#3969=CARTESIAN_POINT ( 'NONE',  ( -9.254189652385859333, -79.87418719991859462, 5.469689899798553689 ) ) ;
#3984=CARTESIAN_POINT ( 'NONE',  ( 9.367484565636001292, -78.93852241191899566, -2.533990228858999938 ) ) ;
#3990=CARTESIAN_POINT ( 'NONE',  ( -9.205306792771352775, -78.60791254279841667, -0.9089956325551382665 ) ) ;
#4009=ORIENTED_EDGE ( 'NONE', *, *, #33603, .T. ) ;
#4011=CARTESIAN_POINT ( 'NONE',  ( 5.626087561713998930, -77.01161118349268975, 9.492708140575000897 ) ) ;
#4014=CARTESIAN_POINT ( 'NONE',  ( 5.816771686847000744, -78.13423299304498926, -7.538935161885000014 ) ) ;
#4025=CARTESIAN_POINT ( 'NONE',  ( -7.579884289019999777, -79.80672464109399300, 7.888812675972000754 ) ) ;
#4027=CARTESIAN_POINT ( 'NONE',  ( 7.164651402987000317, -80.12745930235598735, 8.777043346749001884 ) ) ;
#4033=CIRCLE ( 'NONE', #5942, 1.000000000000000000 ) ;
#4076=EDGE_CURVE ( 'NONE', #13840, #8528, #52658, .T. ) ;
#4086=CARTESIAN_POINT ( 'NONE',  ( 2.799999999999999822, -78.69999999999998863, 0.000000000000000000 ) ) ;
#4087=CARTESIAN_POINT ( 'NONE',  ( -4.615667697956999938, -79.05765853095599027, 8.497672865486000759 ) ) ;
#4099=CARTESIAN_POINT ( 'NONE',  ( 5.272298825061000116, -77.59356652213799066, -9.769775999529000998 ) ) ;
#4106=CARTESIAN_POINT ( 'NONE',  ( 3.269429986698999979, -79.61768715412398478, 9.203886808668999109 ) ) ;
#4116=CARTESIAN_POINT ( 'NONE',  ( -9.497876546326999403, -77.35168256874098347, -0.2008509664869000122 ) ) ;
#4124=CARTESIAN_POINT ( 'NONE',  ( 1.356865283789024712, -79.96379466601229069, 9.149687343425433994 ) ) ;
#4125=CARTESIAN_POINT ( 'NONE',  ( -10.74912230115235801, -80.44221474356261581, 1.099349670086620989 ) ) ;
#4127=CARTESIAN_POINT ( 'NONE',  ( -5.907589619820999616, -78.53973750712998481, 9.593191298321000815 ) ) ;
#4128=B_SPLINE_CURVE_WITH_KNOTS ( 'NONE', 3,
 ( #5350, #6218, #1520, #19812, #665, #54658, #14490, #23644, #18651, #5065, #36639, #23062, #19514, #28353, #14198, #33071, #37509, #41369, #15074, #32483, #46698, #23358, #41075, #5927, #1815, #23932, #27772, #24233, #55527, #32195, #41951, #41657, #55231, #952, #51116, #10670, #50236, #36926, #50527, #9784, #28648, #14778, #28942, #42251, #15377, #37805, #55825, #33370, #45814, #18936, #54940, #10082, #28062, #46108, #1236, #19225, #11818, #25095, #43118, #20954, #38095, #56116, #38671, #46985, #29793 ),
 .UNSPECIFIED., .F., .F.,
 ( 4, 1, 1, 1, 1, 1, 1, 1, 1, 1, 1, 1, 1, 1, 1, 1, 1, 1, 1, 1, 1, 1, 1, 1, 1, 1, 1, 1, 1, 1, 1, 1, 1, 1, 1, 1, 1, 1, 1, 1, 1, 1, 1, 1, 1, 1, 1, 1, 1, 1, 1, 1, 1, 1, 1, 1, 1, 1, 1, 1, 1, 1, 4 ),
 ( 0.000000000000000000, 0.01249975014491727481, 0.02874975858096980377, 0.04499976701702233101, 0.06124977545307485477, 0.07749978388912738547, 0.09374979232517990924, 0.1099998007612324469, 0.1262498091972849568, 0.1424998176333374944, 0.1587498260693900320, 0.1749998345054425419, 0.1912498429414950796, 0.2074998513775475895, 0.2237498598136001271, 0.2399998682496526647, 0.2562498766857052024, 0.2724998851217577678, 0.2887498935578102777, 0.3049999019938627876, 0.3212499104299152974, 0.3374999188659678628, 0.3537499273020203727, 0.3699999357380729381, 0.3862499441741254480, 0.4024999526101780134, 0.4187499610462305233, 0.4349999694822830332, 0.4512499779183355431, 0.4674999863543881085, 0.4837499947904406183, 0.5000000032264931837, 0.5162500116625455826, 0.5325000200985980925, 0.5487500285346506024, 0.5650000369707031123, 0.5812500454067557332, 0.5975000538428082431, 0.6137500622788607529, 0.6300000707149132628, 0.6462500791509657727, 0.6625000875870183936, 0.6787500960230709035, 0.6950001044591234134, 0.7112501128951760343, 0.7275001213312285442, 0.7437501297672810541, 0.7600001382033335640, 0.7762501466393860738, 0.7925001550754385837, 0.8087501635114910936, 0.8250001719475436035, 0.8412501803835962244, 0.8575001888196487343, 0.8737501972557012442, 0.8900002056917537541, 0.9062502141278062640, 0.9225002225638587738, 0.9387502309999112837, 0.9550002394359637936, 0.9712502478720163035, 0.9875002563080689244, 1.000000000000000000 ),
 .UNSPECIFIED. ) ;
#4133=CIRCLE ( 'NONE', #14501, 1.000000000000000000 ) ;
#4135=EDGE_CURVE ( 'NONE', #8528, #52835, #23749, .T. ) ;
#4139=CARTESIAN_POINT ( 'NONE',  ( 10.92153517268999963, -79.29054004199397809, -2.282908042080999955 ) ) ;
#4149=CARTESIAN_POINT ( 'NONE',  ( -7.000000000000000000, -81.10000000285099020, 0.000000000000000000 ) ) ;
#4150=CARTESIAN_POINT ( 'NONE',  ( 5.602396075985502932, -76.95000000000000284, -7.708428217489914580 ) ) ;
#4154=CARTESIAN_POINT ( 'NONE',  ( -7.400482488103000023, -78.65167637952700375, 6.163283938603000500 ) ) ;
#4167=CARTESIAN_POINT ( 'NONE',  ( -10.81649518602000093, -79.41658482343198955, 1.862108609190000097 ) ) ;
#4179=CARTESIAN_POINT ( 'NONE',  ( 9.014082483815000657, -78.44290956889000199, -6.575554473347999362 ) ) ;
#4188=ORIENTED_EDGE ( 'NONE', *, *, #30663, .T. ) ;
#4205=CARTESIAN_POINT ( 'NONE',  ( -0.04490943164332775878, -77.47554393188570998, 9.249810934786108163 ) ) ;
#4208=CARTESIAN_POINT ( 'NONE',  ( 6.240531904507999883, -78.20986865680399092, 7.431451467605000083 ) ) ;
#4226=CARTESIAN_POINT ( 'NONE',  ( -0.2898532571746000319, -80.24379038178499002, -11.39804518048999959 ) ) ;
#4231=ORIENTED_EDGE ( 'NONE', *, *, #10356, .F. ) ;
#4237=CARTESIAN_POINT ( 'NONE',  ( -9.412027495909001118, -79.51667564555398826, 0.4898595818372999400 ) ) ;
#4256=DIRECTION ( 'NONE',  ( -1.000000000000000000, 0.000000000000000000, 0.000000000000000000 ) ) ;
#4260=CARTESIAN_POINT ( 'NONE',  ( 10.71369944335147828, -79.37083333333336554, 2.879226727952053810 ) ) ;
#4265=CARTESIAN_POINT ( 'NONE',  ( 0.000000000000000000, -76.39999999999999147, 0.000000000000000000 ) ) ;
#4277=CARTESIAN_POINT ( 'NONE',  ( -10.47078769030999901, -77.87566818494818222, -3.499536356729999742 ) ) ;
#4283=CARTESIAN_POINT ( 'NONE',  ( -6.473047519705999342, -78.14265519630798451, 7.229824698717000508 ) ) ;
#4285=FACE_OUTER_BOUND ( 'NONE', #26466, .T. ) ;
#4295=CARTESIAN_POINT ( 'NONE',  ( 11.00000000000000000, -78.44999999999998863, 0.000000000000000000 ) ) ;
#4310=CARTESIAN_POINT ( 'NONE',  ( -8.835193196228999568, -77.12585001815408248, 7.003236733173999973 ) ) ;
#4314=CARTESIAN_POINT ( 'NONE',  ( -9.487842642213001554, -77.96369001827098089, -0.8069809344749999669 ) ) ;
#4338=CARTESIAN_POINT ( 'NONE',  ( 5.411006671257999834, -79.57828900368951963, 8.131518144102999557 ) ) ;
#4354=CARTESIAN_POINT ( 'NONE',  ( 4.658259624636106544, -77.76681350748577870, -8.082155137772446096 ) ) ;
#4370=DIRECTION ( 'NONE',  ( 0.000000000000000000, 1.000000000000000000, 0.000000000000000000 ) ) ;
#4378=CIRCLE ( 'NONE', #22283, 4.100000000000000533 ) ;
#4379=ORIENTED_EDGE ( 'NONE', *, *, #13017, .T. ) ;
#4389=CARTESIAN_POINT ( 'NONE',  ( 0.000000000000000000, -77.19999999999998863, 0.000000000000000000 ) ) ;
#4392=DIRECTION ( 'NONE',  ( -1.000000000000000000, 0.000000000000000000, 0.000000000000000000 ) ) ;
#4406=CARTESIAN_POINT ( 'NONE',  ( -9.387315177295000979, -79.80788071282599105, 2.697965643110000311 ) ) ;
#4408=VERTEX_POINT ( 'NONE', #38215 ) ;
#4423=CARTESIAN_POINT ( 'NONE',  ( 5.403870014527243804, -79.92583434048029289, 7.507032179181077680 ) ) ;
#4425=CARTESIAN_POINT ( 'NONE',  ( -10.84994315462449421, -79.96754507315236538, -2.381405434182155112 ) ) ;
#4430=VECTOR ( 'NONE', #18510, 1000.000000000000000 ) ;
#4449=CARTESIAN_POINT ( 'NONE',  ( -1.922928979007999750, -77.25188066968198086, -9.325916353809999393 ) ) ;
#4460=CARTESIAN_POINT ( 'NONE',  ( 4.634563706678000550, -78.77046067378098826, 9.949112313689999709 ) ) ;
#4462=CARTESIAN_POINT ( 'NONE',  ( 10.71369944335146585, -79.32916666666666572, -2.879226727952113318 ) ) ;
#4469=CARTESIAN_POINT ( 'NONE',  ( 8.572837821482822918, -77.28120002596543259, 3.549340890814673966 ) ) ;
#4473=CARTESIAN_POINT ( 'NONE',  ( -10.87436498444000144, -79.73515786819298512, 1.083693866698000052 ) ) ;
#4487=DIRECTION ( 'NONE',  ( -9.386985813191000447E-11, -1.000000000000000000, 5.363052387336999862E-10 ) ) ;
#4490=DIRECTION ( 'NONE',  ( 1.000000000000000000, 0.000000000000000000, 0.000000000000000000 ) ) ;
#4495=CARTESIAN_POINT ( 'NONE',  ( -7.396918292183162436, -79.55208333333334281, -5.684557159767966716 ) ) ;
#4497=CARTESIAN_POINT ( 'NONE',  ( -7.176767133925851638, -78.15496581618874927, -5.904501853725552252 ) ) ;
#4501=ORIENTED_EDGE ( 'NONE', *, *, #1465, .T. ) ;
#4502=CARTESIAN_POINT ( 'NONE',  ( 5.621132263311789501, -77.42329830751356212, 7.378911456533854718 ) ) ;
#4503=CARTESIAN_POINT ( 'NONE',  ( 7.528714304401000312, -78.11486751746299717, -8.074838600060001426 ) ) ;
#4504=CARTESIAN_POINT ( 'NONE',  ( 1.882180247600000245, -78.74992141025498427, 9.519879562373999349 ) ) ;
#4551=CARTESIAN_POINT ( 'NONE',  ( 0.000000000000000000, -80.99999999999998579, 0.000000000000000000 ) ) ;
#4555=EDGE_CURVE ( 'NONE', #24152, #11369, #34302, .T. ) ;
#4581=CARTESIAN_POINT ( 'NONE',  ( 3.248345031021000029, -78.05738370892098033, 9.144340540792999406 ) ) ;
#4584=EDGE_CURVE ( 'NONE', #46717, #24388, #36398, .T. ) ;
#4604=ORIENTED_EDGE ( 'NONE', *, *, #18299, .F. ) ;
#4606=CARTESIAN_POINT ( 'NONE',  ( -9.611650271896850839, -79.15833333333331723, 5.539808784079868431 ) ) ;
#4610=B_SPLINE_CURVE_WITH_KNOTS ( 'NONE', 3,
 ( #49132, #8684, #4260, #22256, #58282, #17845, #53861, #31395, #49435, #22559, #40570, #163, #18138, #54150, #9276, #27265, #24601, #37879 ),
 .UNSPECIFIED., .F., .F.,
 ( 4, 2, 2, 2, 2, 2, 2, 2, 4 ),
 ( 0.000000000000000000, 0.1250000000000000000, 0.2500000000000000000, 0.3750000000000000000, 0.5000000000000000000, 0.6250000000000000000, 0.7500000000000000000, 0.8750000000000000000, 1.000000000000000000 ),
 .UNSPECIFIED. ) ;
#4618=CARTESIAN_POINT ( 'NONE',  ( 9.086766343481999186, -79.24979041159998872, -2.458053382951000287 ) ) ;
#4623=ORIENTED_EDGE ( 'NONE', *, *, #23582, .T. ) ;
#4639=CARTESIAN_POINT ( 'NONE',  ( 11.00000000000000000, -79.44999999999998863, 0.000000000000000000 ) ) ;
#4641=ORIENTED_EDGE ( 'NONE', *, *, #55762, .T. ) ;
#4645=CARTESIAN_POINT ( 'NONE',  ( 9.250000000000000000, -79.34999999999999432, 0.000000000000000000 ) ) ;
#4653=ADVANCED_FACE ( 'NONE', ( #11510 ), #16523, .F. ) ;
#4655=CARTESIAN_POINT ( 'NONE',  ( 0.1948337121880240608, -78.72684273210919059, -9.247945775061792162 ) ) ;
#4658=CARTESIAN_POINT ( 'NONE',  ( 11.00000000000000000, -78.34999999999999432, 0.000000000000000000 ) ) ;
#4673=DIRECTION ( 'NONE',  ( -1.000000000000000000, 0.000000000000000000, 0.000000000000000000 ) ) ;
#4674=ADVANCED_FACE ( 'NONE', ( #31954 ), #27528, .T. ) ;
#4677=CARTESIAN_POINT ( 'NONE',  ( -6.364729966985086307, -78.17625342220868845, -9.067865724216229495 ) ) ;
#4678=VECTOR ( 'NONE', #2965, 1000.000000000000000 ) ;
#4687=CARTESIAN_POINT ( 'NONE',  ( 1.889053048974999927, -78.68865341057399121, 9.554641504766999915 ) ) ;
#4690=CARTESIAN_POINT ( 'NONE',  ( 8.862101803403000133, -79.48419127858598188, -4.393033378783998799 ) ) ;
#4695=AXIS2_PLACEMENT_3D ( 'NONE', #54251, #53073, #48652 ) ;
#4702=VERTEX_POINT ( 'NONE', #3786 ) ;
#4703=CARTESIAN_POINT ( 'NONE',  ( 3.757612933477000094, -77.84086580624799012, 10.56348085686000005 ) ) ;
#4707=EDGE_CURVE ( 'NONE', #34022, #43554, #33497, .T. ) ;
#4708=CARTESIAN_POINT ( 'NONE',  ( 3.366547962069000199, -79.48315413024698728, -9.168809063548000182 ) ) ;
#4712=ADVANCED_FACE ( 'NONE', ( #38646 ), #39510, .F. ) ;
#4720=CARTESIAN_POINT ( 'NONE',  ( -9.626984307556000431, -78.23995771838823998, 1.221426423741999834 ) ) ;
#4721=CARTESIAN_POINT ( 'NONE',  ( 7.994721076134334581, -79.89245675932635038, 4.654034487047796098 ) ) ;
#4725=CARTESIAN_POINT ( 'NONE',  ( -9.350291827225385433, -77.23092893528344405, 2.280442541072182916 ) ) ;
#4733=CARTESIAN_POINT ( 'NONE',  ( 7.439427647571000612, -79.74001771131699456, -8.315438409070999626 ) ) ;
#4752=CARTESIAN_POINT ( 'NONE',  ( -10.96673197750000206, -78.43335242178798694, -0.4413686857046000278 ) ) ;
#4761=CARTESIAN_POINT ( 'NONE',  ( 6.760013919724077169, -77.77708333333333712, -8.796335266379973206 ) ) ;
#4766=CARTESIAN_POINT ( 'NONE',  ( 10.14733453800999996, -78.52718663188798587, 4.639310447764000145 ) ) ;
#4775=ORIENTED_EDGE ( 'NONE', *, *, #51729, .T. ) ;
#4785=CARTESIAN_POINT ( 'NONE',  ( -5.555214266092813880, -78.17374655601618372, -7.396475742313247004 ) ) ;
#4792=ORIENTED_EDGE ( 'NONE', *, *, #40805, .T. ) ;
#4793=CARTESIAN_POINT ( 'NONE',  ( 1.552764912756553706, -77.46160601996280093, 9.119532399810527323 ) ) ;
#4794=CARTESIAN_POINT ( 'NONE',  ( 2.386167682861000117, -77.34811801783499163, 10.77916482977000001 ) ) ;
#4797=CARTESIAN_POINT ( 'NONE',  ( -7.203390125892000562, -78.94888821415699454, -6.502451851937000704 ) ) ;
#4802=CARTESIAN_POINT ( 'NONE',  ( 9.949629901056999515, -78.71331089110499590, 4.548920879513999260 ) ) ;
#4804=CARTESIAN_POINT ( 'NONE',  ( 0.000000000000000000, -81.10000000285099020, -7.000000000000000000 ) ) ;
#4836=B_SPLINE_CURVE_WITH_KNOTS ( 'NONE', 3,
 ( #22588, #44739, #9017, #22290 ),
 .UNSPECIFIED., .F., .F.,
 ( 4, 4 ),
 ( 0.000000000000000000, 0.2499999978686767710 ),
 .UNSPECIFIED. ) ;
#4843=CARTESIAN_POINT ( 'NONE',  ( -3.831287612370999796, -76.92211781146049532, -8.693171758988999187 ) ) ;
#4848=CARTESIAN_POINT ( 'NONE',  ( 0.000000000000000000, -80.99999999999998579, 0.000000000000000000 ) ) ;
#4870=ORIENTED_EDGE ( 'NONE', *, *, #27294, .F. ) ;
#4874=ADVANCED_FACE ( 'NONE', ( #31204 ), #31502, .F. ) ;
#4876=CARTESIAN_POINT ( 'NONE',  ( -2.572125540837000290, -78.31319817108199288, -9.357076443458000270 ) ) ;
#4893=CARTESIAN_POINT ( 'NONE',  ( 0.9151864714589287297, -77.20000000000000284, -10.94417769061167967 ) ) ;
#4910=CARTESIAN_POINT ( 'NONE',  ( -7.696817093642000174, -77.90684236001300178, 5.606191475415999825 ) ) ;
#4923=B_SPLINE_CURVE_WITH_KNOTS ( 'NONE', 3,
 ( #39029, #21024, #2451, #48205, #38450, #7736, #11602, #47048, #25736, #29010, #42604, #47635, #3314, #56178, #34010, #33725, #15727, #7158 ),
 .UNSPECIFIED., .F., .F.,
 ( 4, 2, 2, 2, 2, 2, 2, 2, 4 ),
 ( 0.000000000000000000, 0.1249999999999999722, 0.2500000000000000000, 0.3750000000000000000, 0.5000000000000001110, 0.6250000000000001110, 0.7500000000000000000, 0.8750000000000000000, 1.000000000000000000 ),
 .UNSPECIFIED. ) ;
#4926=EDGE_LOOP ( 'NONE', ( #39471, #21360, #44474, #39902, #44927, #40137 ) ) ;
#4928=DIRECTION ( 'NONE',  ( -1.000000000000000000, 0.000000000000000000, 0.000000000000000000 ) ) ;
#4929=DIRECTION ( 'NONE',  ( 0.000000000000000000, -1.000000000000000000, 0.000000000000000000 ) ) ;
#4942=CARTESIAN_POINT ( 'NONE',  ( 6.543182841190322563, -78.78770266721694782, -6.538132477336259463 ) ) ;
#4945=CARTESIAN_POINT ( 'NONE',  ( -11.00000000000000888, -78.58958333333332291, 1.439896632895276252 ) ) ;
#4950=EDGE_CURVE ( 'NONE', #31999, #30580, #20918, .T. ) ;
#4960=CARTESIAN_POINT ( 'NONE',  ( -7.000000000000000000, -80.99999999999998579, 0.000000000000000000 ) ) ;
#4973=AXIS2_PLACEMENT_3D ( 'NONE', #48728, #39567, #22432 ) ;
#4976=CARTESIAN_POINT ( 'NONE',  ( -1.000000000000000000, -81.19999999999998863, 7.000000000000000000 ) ) ;
#4978=ORIENTED_EDGE ( 'NONE', *, *, #43478, .F. ) ;
#4986=VERTEX_POINT ( 'NONE', #9977 ) ;
#4987=CARTESIAN_POINT ( 'NONE',  ( 3.570960563072000049, -77.14385634160659322, -10.62807481261000220 ) ) ;
#4990=ORIENTED_EDGE ( 'NONE', *, *, #14207, .F. ) ;
#4995=CARTESIAN_POINT ( 'NONE',  ( 5.411006671257999834, -79.15842754766698874, 8.131518144102999557 ) ) ;
#5007=CARTESIAN_POINT ( 'NONE',  ( 5.434802443507552816, -79.92549811133810067, 7.484660366369180196 ) ) ;
#5009=ORIENTED_EDGE ( 'NONE', *, *, #32647, .F. ) ;
#5010=CARTESIAN_POINT ( 'NONE',  ( -7.805809014822999714, -80.05672464109399300, 8.123945268076997905 ) ) ;
#5019=CARTESIAN_POINT ( 'NONE',  ( 10.89322882296999850, -79.82429477431499265, 2.414366480783999958 ) ) ;
#5025=VERTEX_POINT ( 'NONE', #36536 ) ;
#5028=CARTESIAN_POINT ( 'NONE',  ( -9.309367086190000862, -77.13855160546319212, -0.1968645694141999969 ) ) ;
#5030=CARTESIAN_POINT ( 'NONE',  ( 0.7461282319042067401, -76.94999999999998863, -9.500000001998314403 ) ) ;
#5033=CARTESIAN_POINT ( 'NONE',  ( 7.919085842678998510, -78.97136658247099206, -5.669895566145999766 ) ) ;
#5037=ORIENTED_EDGE ( 'NONE', *, *, #13444, .F. ) ;
#5046=CARTESIAN_POINT ( 'NONE',  ( 10.71556987377000070, -79.75781129242999157, 2.374990294079000197 ) ) ;
#5049=DIRECTION ( 'NONE',  ( 0.000000000000000000, -1.000000000000000000, 0.000000000000000000 ) ) ;
#5059=CARTESIAN_POINT ( 'NONE',  ( -9.501885680564001291, -79.34955593965399601, -5.638445012646999821 ) ) ;
#5065=CARTESIAN_POINT ( 'NONE',  ( -8.631516086050529779, -78.39711804219207636, 6.779730741015662865 ) ) ;
#5072=ORIENTED_EDGE ( 'NONE', *, *, #19257, .F. ) ;
#5073=CARTESIAN_POINT ( 'NONE',  ( -9.250000000000000000, -78.09999999999999432, 0.000000000000000000 ) ) ;
#5082=ORIENTED_EDGE ( 'NONE', *, *, #21481, .F. ) ;
#5084=ORIENTED_EDGE ( 'NONE', *, *, #36701, .F. ) ;
#5085=CARTESIAN_POINT ( 'NONE',  ( -0.4327165701982794155, -77.47889716067786026, 9.240429326102006513 ) ) ;
#5086=CARTESIAN_POINT ( 'NONE',  ( 10.90987126150000108, -77.19238596616818882, 1.690571823134000118 ) ) ;
#5089=CARTESIAN_POINT ( 'NONE',  ( -9.446433787353997857, -78.40883546070699595, -2.221620594898999990 ) ) ;
#5091=DIRECTION ( 'NONE',  ( 1.000000000000000000, 0.000000000000000000, 0.000000000000000000 ) ) ;
#5094=CARTESIAN_POINT ( 'NONE',  ( -8.032634178075001685, -78.48857205644399926, -7.427287829177999789 ) ) ;
#5105=CARTESIAN_POINT ( 'NONE',  ( 10.36935812844000004, -78.17876026662598576, -2.835297515976000327 ) ) ;
#5109=CARTESIAN_POINT ( 'NONE',  ( -9.379486438909999890, -77.58593853670399199, -0.7977647835019999745 ) ) ;
#5115=VERTEX_POINT ( 'NONE', #22671 ) ;
#5117=DIRECTION ( 'NONE',  ( 0.000000000000000000, -1.000000000000000000, 0.000000000000000000 ) ) ;
#5120=EDGE_CURVE ( 'NONE', #44860, #1033, #13413, .T. ) ;
#5123=CYLINDRICAL_SURFACE ( 'NONE', #36612, 9.250000000000000000 ) ;
#5131=CARTESIAN_POINT ( 'NONE',  ( -10.71960490440000058, -78.15429499344598696, 3.466843673432000283 ) ) ;
#5137=CARTESIAN_POINT ( 'NONE',  ( -4.100000000000000533, -77.49999999999998579, 0.000000000000000000 ) ) ;
#5150=CARTESIAN_POINT ( 'NONE',  ( -4.017143116098000455, -80.25404428795494027, 10.51352533724000082 ) ) ;
#5162=CARTESIAN_POINT ( 'NONE',  ( 9.583411031200000707, -77.97211222153399035, 1.526087275887999972 ) ) ;
#5163=CARTESIAN_POINT ( 'NONE',  ( 9.750000000000000000, -76.19999999999998863, 0.000000000000000000 ) ) ;
#5180=DIRECTION ( 'NONE',  ( 0.000000000000000000, -1.000000000000000000, 0.000000000000000000 ) ) ;
#5182=CARTESIAN_POINT ( 'NONE',  ( 11.00000000000000000, -78.94999999999998863, -1.064824513673000067E-14 ) ) ;
#5184=EDGE_CURVE ( 'NONE', #13151, #31999, #27297, .T. ) ;
#5186=CARTESIAN_POINT ( 'NONE',  ( 9.434081066526999848, -79.55882968926798071, -2.467387813727000001 ) ) ;
#5194=CARTESIAN_POINT ( 'NONE',  ( 10.85646270852000050, -77.97987769867899033, -1.809030205320999896 ) ) ;
#5198=CARTESIAN_POINT ( 'NONE',  ( -2.142155038640999987, -77.84999470175499425, 9.278014228403000274 ) ) ;
#5199=EDGE_CURVE ( 'NONE', #33222, #10301, #17262, .T. ) ;
#5207=ORIENTED_EDGE ( 'NONE', *, *, #1611, .F. ) ;
#5208=ORIENTED_EDGE ( 'NONE', *, *, #24516, .T. ) ;
#5223=CARTESIAN_POINT ( 'NONE',  ( -7.396672774822746987, -79.15237237872500486, -5.684931589052010459 ) ) ;
#5224=CARTESIAN_POINT ( 'NONE',  ( -6.473154694944447840, -78.28301520904093991, 7.229944404031765082 ) ) ;
#5233=CARTESIAN_POINT ( 'NONE',  ( 6.769093727302936792, -78.79047469916130808, -6.304424132926785163 ) ) ;
#5235=DIRECTION ( 'NONE',  ( 0.000000000000000000, 1.000000000000000000, 0.000000000000000000 ) ) ;
#5236=CARTESIAN_POINT ( 'NONE',  ( -4.186946963469314831, -80.19418132811986766, -10.17752948135066049 ) ) ;
#5244=CARTESIAN_POINT ( 'NONE',  ( 8.760175664411535834, -79.99999999999998579, 3.616861466383621160 ) ) ;
#5252=CARTESIAN_POINT ( 'NONE',  ( 6.768882593647018275, -77.27178109534467865, 8.462659279992045924 ) ) ;
#5272=CARTESIAN_POINT ( 'NONE',  ( 2.166634614239063377E-07, -77.01246206852036380, -9.437473063691797392 ) ) ;
#5284=CARTESIAN_POINT ( 'NONE',  ( 9.767191983224998708, -79.76072787413951914, 0.05162932631433000269 ) ) ;
#5296=CARTESIAN_POINT ( 'NONE',  ( 9.116782980790521407, -79.86451097818435585, 1.648924484312454419 ) ) ;
#5311=CARTESIAN_POINT ( 'NONE',  ( 10.58947069987000056, -78.34309102680099102, -3.845989281283999528 ) ) ;
#5312=DIRECTION ( 'NONE',  ( 0.000000000000000000, 1.000000000000000000, 0.000000000000000000 ) ) ;
#5324=CARTESIAN_POINT ( 'NONE',  ( 8.982692273745001899, -77.48629938523899341, 3.473391639513999429 ) ) ;
#5331=CARTESIAN_POINT ( 'NONE',  ( -2.928603948516999900, -78.88694830811698466, 10.57767911662999971 ) ) ;
#5336=LINE ( 'NONE', #55514, #41904 ) ;
#5343=CARTESIAN_POINT ( 'NONE',  ( -3.571993175857000491, -79.40574064831898227, -10.45556112308999985 ) ) ;
#5346=AXIS2_PLACEMENT_3D ( 'NONE', #35964, #1153, #14690 ) ;
#5350=CARTESIAN_POINT ( 'NONE',  ( 10.36935812844000004, -78.17876026662598576, -2.835297515976000327 ) ) ;
#5368=CARTESIAN_POINT ( 'NONE',  ( 10.61050599188999932, -77.92876026662598576, -2.901234667509999809 ) ) ;
#5370=CARTESIAN_POINT ( 'NONE',  ( 8.392153346702146521, -77.38471673975136866, 3.904227155189466725 ) ) ;
#5371=CARTESIAN_POINT ( 'NONE',  ( 5.341789944771999643, -77.70465779647399529, 9.661750877468000098 ) ) ;
#5377=CARTESIAN_POINT ( 'NONE',  ( 11.10498291493000167, -80.22745348979398727, -1.830582403018000015 ) ) ;
#5378=CARTESIAN_POINT ( 'NONE',  ( 0.2605153439964000284, -79.55608152108499098, -10.93709047653000077 ) ) ;
#5392=CARTESIAN_POINT ( 'NONE',  ( 4.409055568808000203, -77.41539556192998361, 8.316935944130001701 ) ) ;
#5402=CARTESIAN_POINT ( 'NONE',  ( 10.28103400416999946, -78.14831066145598015, 3.842432268884000024 ) ) ;
#5411=CARTESIAN_POINT ( 'NONE',  ( 10.58947069987000056, -77.90146380445199270, -3.845989281283999528 ) ) ;
#5423=CARTESIAN_POINT ( 'NONE',  ( -9.549999999999998934, -76.89999999999999147, 0.000000000000000000 ) ) ;
#5435=CARTESIAN_POINT ( 'NONE',  ( 5.154876033940102964, -78.27220474274599837, -7.680359545439894298 ) ) ;
#5441=CARTESIAN_POINT ( 'NONE',  ( 0.000000000000000000, -78.69999999999998863, 0.000000000000000000 ) ) ;
#5446=CARTESIAN_POINT ( 'NONE',  ( 2.260091721765999928, -78.91355385020298741, -9.437303113984999214 ) ) ;
#5466=ORIENTED_EDGE ( 'NONE', *, *, #32095, .T. ) ;
#5476=CARTESIAN_POINT ( 'NONE',  ( -2.009571257635000219, -77.19648208238979237, 10.87244111694000104 ) ) ;
#5479=CARTESIAN_POINT ( 'NONE',  ( -7.476203163627999970, -77.57278449298998169, -5.719923538308999689 ) ) ;
#5484=FACE_BOUND ( 'NONE', #26744, .T. ) ;
#5502=DIRECTION ( 'NONE',  ( 1.000000000000000000, 0.000000000000000000, 0.000000000000000000 ) ) ;
#5503=ORIENTED_EDGE ( 'NONE', *, *, #26459, .F. ) ;
#5504=EDGE_CURVE ( 'NONE', #3819, #56496, #27179, .T. ) ;
#5506=CARTESIAN_POINT ( 'NONE',  ( -1.959727320071604773, -77.45872416430094631, -9.504382773771103743 ) ) ;
#5511=CARTESIAN_POINT ( 'NONE',  ( -9.549999999953000085, -76.40000000004698677, 5.125988344190999543E-10 ) ) ;
#5514=CARTESIAN_POINT ( 'NONE',  ( 1.565620768230334470, -78.73876823178706275, -9.127934873522015380 ) ) ;
#5529=CARTESIAN_POINT ( 'NONE',  ( 10.36935812844000004, -78.17876026662598576, -2.835297515976000327 ) ) ;
#5532=CARTESIAN_POINT ( 'NONE',  ( -10.56885402377634797, -77.43492478567101500, 2.086924253389536243 ) ) ;
#5541=CARTESIAN_POINT ( 'NONE',  ( 8.333454457512889491, -78.31429970678456698, -4.014433121081317779 ) ) ;
#5545=CARTESIAN_POINT ( 'NONE',  ( 2.243017272178000177, -79.03676744264699039, -9.366006557871001448 ) ) ;
#5547=CARTESIAN_POINT ( 'NONE',  ( -8.141768944221999149, -79.22275767078099307, 5.616688595088000113 ) ) ;
#5551=CARTESIAN_POINT ( 'NONE',  ( -4.299999999999999822, -81.99999999999998579, 0.000000000000000000 ) ) ;
#5556=ORIENTED_EDGE ( 'NONE', *, *, #2903, .F. ) ;
#5562=CARTESIAN_POINT ( 'NONE',  ( -7.298419138992000121, -77.99709831745698807, -8.365328406272000805 ) ) ;
#5568=CARTESIAN_POINT ( 'NONE',  ( 9.767191983224998708, -79.64087503069099228, 0.05162932631433000269 ) ) ;
#5569=ORIENTED_EDGE ( 'NONE', *, *, #2704, .T. ) ;
#5578=CARTESIAN_POINT ( 'NONE',  ( -9.160649592606999292, -77.23931109735399048, 3.828331730729000348 ) ) ;
#5588=LINE ( 'NONE', #9454, #38341 ) ;
#5589=CARTESIAN_POINT ( 'NONE',  ( -0.6622892437428000711, -79.93666419164598835, 11.13790800686000004 ) ) ;
#5593=ORIENTED_EDGE ( 'NONE', *, *, #23115, .T. ) ;
#5596=CARTESIAN_POINT ( 'NONE',  ( -9.395951288910000088, -77.37666898275598726, 1.963411011382999893 ) ) ;
#5597=CARTESIAN_POINT ( 'NONE',  ( 7.000000000000000000, -81.19999999999998863, 0.000000000000000000 ) ) ;
#5598=CIRCLE ( 'NONE', #48969, 1.199999999999999956 ) ;
#5603=CARTESIAN_POINT ( 'NONE',  ( -9.612747958823000261, -77.20206109394898419, 0.5898851805584000019 ) ) ;
#5610=DIRECTION ( 'NONE',  ( 0.000000000000000000, 0.000000000000000000, -1.000000000000000000 ) ) ;
#5612=CARTESIAN_POINT ( 'NONE',  ( -5.684974983678790394, -78.02723969034931883, 7.397314429064029362 ) ) ;
#5614=CARTESIAN_POINT ( 'NONE',  ( -6.405050160242000246, -78.91504066244898752, 8.912875463421000788 ) ) ;
#5615=CARTESIAN_POINT ( 'NONE',  ( 2.879226727952061360, -79.24583333333333712, -10.71369944335147828 ) ) ;
#5622=CARTESIAN_POINT ( 'NONE',  ( -4.849178099734126057, -77.41866321790520544, 7.910227586308292480 ) ) ;
#5632=CARTESIAN_POINT ( 'NONE',  ( 9.250000000000000000, -79.74999999999998579, 1.907449677260999760E-14 ) ) ;
#5637=EDGE_LOOP ( 'NONE', ( #14200, #52764, #4231, #5593 ) ) ;
#5642=CARTESIAN_POINT ( 'NONE',  ( 0.000000000000000000, -74.64999999999999147, 0.000000000000000000 ) ) ;
#5654=CARTESIAN_POINT ( 'NONE',  ( 8.217637274874787678, -77.38807705323522157, 4.246385049674642254 ) ) ;
#5663=CARTESIAN_POINT ( 'NONE',  ( 9.203868716350999790, -79.72463564708098716, 5.914103205931999341 ) ) ;
#5677=CARTESIAN_POINT ( 'NONE',  ( 4.061470846528000500, -78.23968660667100039, -8.492093326754000415 ) ) ;
#5679=EDGE_CURVE ( 'NONE', #32058, #54228, #41317, .T. ) ;
#5688=CARTESIAN_POINT ( 'NONE',  ( -9.505686244346000180, -79.26788661775799483, 5.486888517706000279 ) ) ;
#5693=COLOUR_RGB ( '', 0.08235294, 0.09019608, 0.10196078) ;
#5710=( LENGTH_UNIT ( ) NAMED_UNIT ( * ) SI_UNIT ( .MILLI., .METRE. ) );
#5724=CARTESIAN_POINT ( 'NONE',  ( 3.903619169069028949, -78.25971142198206110, -8.387417762067762794 ) ) ;
#5728=CARTESIAN_POINT ( 'NONE',  ( -8.325424899317864558, -77.56401563986393910, 4.046370920615864009 ) ) ;
#5734=CIRCLE ( 'NONE', #22714, 1.199999999999999956 ) ;
#5735=CARTESIAN_POINT ( 'NONE',  ( -9.157500079073999544, -78.74301087542899324, 3.211059275314999795 ) ) ;
#5749=CARTESIAN_POINT ( 'NONE',  ( -9.250000000000000000, -79.59999999999999432, 0.000000000000000000 ) ) ;
#5756=CARTESIAN_POINT ( 'NONE',  ( 5.539808784079903070, -79.03333333333333144, 9.611650271896831299 ) ) ;
#5758=CARTESIAN_POINT ( 'NONE',  ( -3.587367123708000261, -79.73416563881599473, 9.067562258818998799 ) ) ;
#5761=DIRECTION ( 'NONE',  ( 0.000000000000000000, 1.000000000000000000, 0.000000000000000000 ) ) ;
#5764=CARTESIAN_POINT ( 'NONE',  ( 11.06229936814999881, -77.50388255425598061, 1.513518412900999977 ) ) ;
#5768=AXIS2_PLACEMENT_3D ( 'NONE', #27204, #30257, #35258 ) ;
#5769=CARTESIAN_POINT ( 'NONE',  ( 4.409055568808000203, -77.85702278427999090, 8.316935944130001701 ) ) ;
#5789=ORIENTED_EDGE ( 'NONE', *, *, #55973, .F. ) ;
#5798=CARTESIAN_POINT ( 'NONE',  ( 4.746119756384775457, -77.51557182255893963, -8.464524489953728192 ) ) ;
#5802=CARTESIAN_POINT ( 'NONE',  ( 6.983565664416999219, -78.43892452229077605, -6.737990796766999857 ) ) ;
#5806=CARTESIAN_POINT ( 'NONE',  ( 2.087132440259329424, -78.74332257418703307, -9.032315042655973514 ) ) ;
#5819=CARTESIAN_POINT ( 'NONE',  ( 7.650805994261745901, -79.99999999999998579, 5.540479312588552752 ) ) ;
#5835=EDGE_CURVE ( 'NONE', #45319, #27414, #3950, .T. ) ;
#5836=CARTESIAN_POINT ( 'NONE',  ( 7.585176102898188333, -78.30167758068601813, -5.294072734977127048 ) ) ;
#5840=CARTESIAN_POINT ( 'NONE',  ( -4.778484498315999751, -78.80937680961498870, 8.361775879827998637 ) ) ;
#5851=CARTESIAN_POINT ( 'NONE',  ( -10.83547269566999915, -79.70737966341999936, -4.008037460590999856 ) ) ;
#5854=CARTESIAN_POINT ( 'NONE',  ( 5.497693353104999403, -77.32727988493299165, 9.771496850480000163 ) ) ;
#5860=CARTESIAN_POINT ( 'NONE',  ( 5.496668217546000434, -80.06301958804498042, -8.073860231047000013 ) ) ;
#5889=CARTESIAN_POINT ( 'NONE',  ( -0.5083718267365000543, -77.20835577409998507, 9.693975953357998776 ) ) ;
#5895=CARTESIAN_POINT ( 'NONE',  ( 9.401690036064000111, -78.99979041159998872, -2.543243121375000193 ) ) ;
#5905=CARTESIAN_POINT ( 'NONE',  ( 8.867070753125000593, -78.69030182778799087, -6.468312982590000537 ) ) ;
#5908=CARTESIAN_POINT ( 'NONE',  ( 1.654508304067999980, -79.28174448050398837, -9.527719980787999532 ) ) ;
#5913=AXIS2_PLACEMENT_3D ( 'NONE', #42949, #2506, #20510 ) ;
#5918=AXIS2_PLACEMENT_3D ( 'NONE', #15638, #28916, #29203 ) ;
#5924=EDGE_CURVE ( 'NONE', #49174, #48925, #44490, .T. ) ;
#5927=CARTESIAN_POINT ( 'NONE',  ( 4.634636847927953163, -78.79041100284936761, 9.949269327501806259 ) ) ;
#5942=AXIS2_PLACEMENT_3D ( 'NONE', #27349, #9358, #4928 ) ;
#5947=CARTESIAN_POINT ( 'NONE',  ( 8.729031720696649899, -77.37686029687922940, 3.060862442712833698 ) ) ;
#5951=VECTOR ( 'NONE', #16160, 1000.000000000000114 ) ;
#5958=CARTESIAN_POINT ( 'NONE',  ( 3.902863791433999641, -79.27515797775897965, 10.22034591202999820 ) ) ;
#5962=VERTEX_POINT ( 'NONE', #5163 ) ;
#5971=CARTESIAN_POINT ( 'NONE',  ( -8.508571376020000798, -77.61436236583298864, -4.026835934908000070 ) ) ;
#5977=DIRECTION ( 'NONE',  ( -1.000000000000000000, 0.000000000000000000, 0.000000000000000000 ) ) ;
#5981=CARTESIAN_POINT ( 'NONE',  ( 5.330173052271000245, -78.20449537012198959, 9.594439332582000546 ) ) ;
#5995=CARTESIAN_POINT ( 'NONE',  ( 2.935661446561999899, -79.99999999999998579, -9.035036904803998681 ) ) ;
#6010=ORIENTED_EDGE ( 'NONE', *, *, #14252, .T. ) ;
#6012=DIRECTION ( 'NONE',  ( -1.000000000000000000, 0.000000000000000000, 0.000000000000000000 ) ) ;
#6017=CARTESIAN_POINT ( 'NONE',  ( 3.540263149936455633, -78.25629661996973141, -8.545667284253724461 ) ) ;
#6021=CARTESIAN_POINT ( 'NONE',  ( -7.544460730989308139, -77.55089713445312327, 5.352097458047992973 ) ) ;
#6025=CARTESIAN_POINT ( 'NONE',  ( -3.536681740116999872, -78.17453429284898903, 9.036735673663999435 ) ) ;
#6026=DIRECTION ( 'NONE',  ( 0.000000000000000000, 1.000000000000000000, 0.000000000000000000 ) ) ;
#6041=CARTESIAN_POINT ( 'NONE',  ( 4.769507551644696974, -80.00000000000000000, -8.276756506782131595 ) ) ;
#6044=CARTESIAN_POINT ( 'NONE',  ( 9.802742422367249020, -77.20000000000000284, -4.551162862351648464 ) ) ;
#6047=LINE ( 'NONE', #15198, #36080 ) ;
#6048=EDGE_CURVE ( 'NONE', #16887, #43630, #43401, .T. ) ;
#6051=CARTESIAN_POINT ( 'NONE',  ( -3.547312378341000549, -79.79804137959898469, 8.966318398112001375 ) ) ;
#6056=CARTESIAN_POINT ( 'NONE',  ( -7.421505610835000155, -77.61136506546499447, 8.486883608244999877 ) ) ;
#6065=FACE_OUTER_BOUND ( 'NONE', #41707, .T. ) ;
#6094=CARTESIAN_POINT ( 'NONE',  ( -6.473047519705999342, -78.18311006013023245, 7.229824698717000508 ) ) ;
#6101=CARTESIAN_POINT ( 'NONE',  ( -6.480567632827825442, -78.66327994001753154, -6.600377077318754004 ) ) ;
#6105=VECTOR ( 'NONE', #58216, 1000.000000000000114 ) ;
#6106=CARTESIAN_POINT ( 'NONE',  ( -5.531057285270385648, -80.18318348377982829, -9.508306399520915164 ) ) ;
#6113=CARTESIAN_POINT ( 'NONE',  ( 9.025284355001986114, -80.00000000000000000, 2.926013110658441274 ) ) ;
#6125=CARTESIAN_POINT ( 'NONE',  ( 4.634563706678000550, -78.69030876264459096, 9.949112313689999709 ) ) ;
#6134=CARTESIAN_POINT ( 'NONE',  ( -9.316314781052998484, -77.35273344151198671, -2.840095070410999956 ) ) ;
#6145=CARTESIAN_POINT ( 'NONE',  ( 9.012516225103091472, -77.72930688072841576, -2.404885370045733772 ) ) ;
#6158=CARTESIAN_POINT ( 'NONE',  ( -7.479908383216000267, -79.44603908114399360, -6.281056869080000382 ) ) ;
#6185=CARTESIAN_POINT ( 'NONE',  ( 5.231719136747999599, -76.99948083835489854, -8.176838819753999843 ) ) ;
#6190=CARTESIAN_POINT ( 'NONE',  ( -0.5568870975076999352, -77.89126107556998591, -9.723660445896001647 ) ) ;
#6195=ORIENTED_EDGE ( 'NONE', *, *, #54364, .T. ) ;
#6197=CARTESIAN_POINT ( 'NONE',  ( 9.008910651542503700, -77.87100497140035316, 2.420997400874941974 ) ) ;
#6199=CARTESIAN_POINT ( 'NONE',  ( 6.083963560182000130, -78.66220947345499326, -9.135064530700001129 ) ) ;
#6201=CARTESIAN_POINT ( 'NONE',  ( 5.642630579966001036, -79.46848277179400100, 7.853379265792000297 ) ) ;
#6216=FACE_OUTER_BOUND ( 'NONE', #31158, .T. ) ;
#6218=CARTESIAN_POINT ( 'NONE',  ( 10.62559031388325614, -78.18606552174667002, -1.896613003017499244 ) ) ;
#6225=ORIENTED_EDGE ( 'NONE', *, *, #2262, .F. ) ;
#6238=CARTESIAN_POINT ( 'NONE',  ( 9.097059317135745005, -77.36466295629431045, 1.675254618218271263 ) ) ;
#6245=CARTESIAN_POINT ( 'NONE',  ( -10.66249531825000041, -79.92128212740999516, 1.062579819291000094 ) ) ;
#6252=CARTESIAN_POINT ( 'NONE',  ( -10.17160039975009767, -77.19999999999998863, 4.054394401284254101 ) ) ;
#6261=CARTESIAN_POINT ( 'NONE',  ( 8.631984821280999753, -78.29653426492899371, -3.755001005681000148 ) ) ;
#6271=CARTESIAN_POINT ( 'NONE',  ( -10.79326785783000098, -79.32407132642299530, -1.992331681952000055 ) ) ;
#6290=VECTOR ( 'NONE', #43408, 1000.000000000000000 ) ;
#6301=ORIENTED_EDGE ( 'NONE', *, *, #18720, .T. ) ;
#6311=CARTESIAN_POINT ( 'NONE',  ( 5.769691659566330344, -78.27875186636556748, -7.231031389465585768 ) ) ;
#6320=CARTESIAN_POINT ( 'NONE',  ( -8.680270256945998852, -77.17624500592239656, 3.860428508128000313 ) ) ;
#6324=CARTESIAN_POINT ( 'NONE',  ( 7.000000000000000000, -81.19999999999998863, 0.000000000000000000 ) ) ;
#6333=DIRECTION ( 'NONE',  ( -2.708260965908999685E-12, 1.000000000000000000, -1.232643895471000067E-11 ) ) ;
#6334=LINE ( 'NONE', #2215, #39150 ) ;
#6345=CARTESIAN_POINT ( 'NONE',  ( 5.288697200961000711, -79.56426011353597971, -8.062752175145998734 ) ) ;
#6348=EDGE_CURVE ( 'NONE', #45667, #15896, #16228, .T. ) ;
#6352=CARTESIAN_POINT ( 'NONE',  ( -2.029340489805000036, -77.13260634160660345, 10.97939916177999997 ) ) ;
#6360=AXIS2_PLACEMENT_3D ( 'NONE', #27352, #28212, #5502 ) ;
#6370=ORIENTED_EDGE ( 'NONE', *, *, #57467, .F. ) ;
#6384=CARTESIAN_POINT ( 'NONE',  ( 3.561977969011698608, -79.25638847529646114, -8.599364659723994109 ) ) ;
#6389=CARTESIAN_POINT ( 'NONE',  ( -9.702231720816998362, -78.75158664270975351, -0.1934140619087000024 ) ) ;
#6391=CARTESIAN_POINT ( 'NONE',  ( 2.935661446561999899, -79.99999999999998579, -9.035036904803998681 ) ) ;
#6394=CARTESIAN_POINT ( 'NONE',  ( -6.420806408779561103, -78.66401051080144669, -6.658731949244796056 ) ) ;
#6397=CARTESIAN_POINT ( 'NONE',  ( -7.554596112399141639, -80.16517684970969526, -7.995309787463595441 ) ) ;
#6409=CARTESIAN_POINT ( 'NONE',  ( -1.210642416637526475, -79.71502597872630247, -9.250941057579437299 ) ) ;
#6415=CARTESIAN_POINT ( 'NONE',  ( -10.26045602449772964, -77.92435585664894404, 3.486900230140368873 ) ) ;
#6417=CARTESIAN_POINT ( 'NONE',  ( 0.1291013223160000223, -79.22406349496543498, 10.97485077030000333 ) ) ;
#6422=CARTESIAN_POINT ( 'NONE',  ( 7.537139175769687505, -78.30095851910974147, -5.362098310969546588 ) ) ;
#6426=CARTESIAN_POINT ( 'NONE',  ( 9.164371241867000251, -77.55170024541499174, -3.297574176498999865 ) ) ;
#6432=DIRECTION ( 'NONE',  ( 0.000000000000000000, 0.000000000000000000, -1.000000000000000000 ) ) ;
#6438=CARTESIAN_POINT ( 'NONE',  ( -7.369179516270000008, -79.74914082875798726, -8.897431359219000413 ) ) ;
#6441=CARTESIAN_POINT ( 'NONE',  ( -4.507968364102000081, -77.46452504304699005, 10.38607047735999878 ) ) ;
#6447=CARTESIAN_POINT ( 'NONE',  ( 9.202039358297998461, -80.51999609317051920, 2.360608321670000453 ) ) ;
#6455=DIRECTION ( 'NONE',  ( 0.000000000000000000, 1.000000000000000000, 0.000000000000000000 ) ) ;
#6460=CARTESIAN_POINT ( 'NONE',  ( -9.380723093181000394, -77.11069873435108946, 0.6187074708012999524 ) ) ;
#6465=ADVANCED_FACE ( 'NONE', ( #29253 ), #27588, .F. ) ;
#6475=VERTEX_POINT ( 'NONE', #56999 ) ;
#6477=CARTESIAN_POINT ( 'NONE',  ( 9.031968385043001035, -77.11557531307438751, -3.250018536810999947 ) ) ;
#6478=DIRECTION ( 'NONE',  ( 0.000000000000000000, 1.000000000000000000, 0.000000000000000000 ) ) ;
#6482=CARTESIAN_POINT ( 'NONE',  ( 7.686826547751000938, -78.57343297466498200, 5.981002702827999506 ) ) ;
#6494=LINE ( 'NONE', #29497, #51556 ) ;
#6495=CARTESIAN_POINT ( 'NONE',  ( 6.891029062618999390, -79.89012658836398373, 6.626049502339999897 ) ) ;
#6530=ORIENTED_EDGE ( 'NONE', *, *, #25865, .T. ) ;
#6531=CARTESIAN_POINT ( 'NONE',  ( 9.123750851018394670, -77.36332806067234458, 1.522676030713496331 ) ) ;
#6532=CARTESIAN_POINT ( 'NONE',  ( -9.808193611224998776, -77.95250248247700142, 5.067887917229000116 ) ) ;
#6533=CONICAL_SURFACE ( 'NONE', #48028, 1.099999997148999986, 0.7853981633972997312 ) ;
#6537=CARTESIAN_POINT ( 'NONE',  ( 9.549999999953000085, -76.40000000004698677, -5.125981083096999748E-10 ) ) ;
#6543=CARTESIAN_POINT ( 'NONE',  ( -11.03994916103999913, -78.49626308856198875, -0.4443153950920000206 ) ) ;
#6548=VERTEX_POINT ( 'NONE', #56430 ) ;
#6558=CARTESIAN_POINT ( 'NONE',  ( 2.217690073412000196, -78.78676744264699039, -9.260249588150999855 ) ) ;
#6561=DIRECTION ( 'NONE',  ( 0.000000000000000000, 0.000000000000000000, -1.000000000000000000 ) ) ;
#6569=CARTESIAN_POINT ( 'NONE',  ( 0.2613587267741000475, -79.43644074375399100, -10.97249781033000104 ) ) ;
#6577=CARTESIAN_POINT ( 'NONE',  ( 2.879226727952050258, -78.05416666666666003, 10.71369944335148361 ) ) ;
#6579=CARTESIAN_POINT ( 'NONE',  ( 3.390474011741000382, -78.82851149742998587, -10.74400392503999946 ) ) ;
#6591=CARTESIAN_POINT ( 'NONE',  ( 1.199999999999999956, -80.99999999999998579, 7.000000000000000000 ) ) ;
#6592=ORIENTED_EDGE ( 'NONE', *, *, #9898, .F. ) ;
#6598=ORIENTED_EDGE ( 'NONE', *, *, #11428, .T. ) ;
#6603=CARTESIAN_POINT ( 'NONE',  ( 6.550831367461507071, -78.28762608587432226, -6.530619802353137437 ) ) ;
#6605=EDGE_LOOP ( 'NONE', ( #30821, #8062, #25259, #28652 ) ) ;
#6606=AXIS2_PLACEMENT_3D ( 'NONE', #37594, #33153, #14279 ) ;
#6613=CARTESIAN_POINT ( 'NONE',  ( 8.444976262095000408, -78.06083897633399715, 4.780490068936999570 ) ) ;
#6614=CARTESIAN_POINT ( 'NONE',  ( -9.247932426686000795, -77.50168256874098915, -0.1955654147372000162 ) ) ;
#6631=CARTESIAN_POINT ( 'NONE',  ( 10.90030694484000051, -80.19320782078999343, 1.940743536767000066 ) ) ;
#6640=CARTESIAN_POINT ( 'NONE',  ( -7.635222642325999232, -80.00803041167199581, -5.709097800406000012 ) ) ;
#6642=CARTESIAN_POINT ( 'NONE',  ( -4.837304822058766440, -79.43335073634851540, -8.426485034531916440 ) ) ;
#6645=CARTESIAN_POINT ( 'NONE',  ( 0.000000000000000000, -80.74999999986198418, 0.000000000000000000 ) ) ;
#6646=CARTESIAN_POINT ( 'NONE',  ( -9.228378915705999219, -77.85335538169299241, -6.089758258776999611 ) ) ;
#6649=CARTESIAN_POINT ( 'NONE',  ( -6.279067761433998918, -78.45392319598897757, 7.013166371532999932 ) ) ;
#6652=DIRECTION ( 'NONE',  ( 0.000000000000000000, -1.000000000000000000, 0.000000000000000000 ) ) ;
#6665=CIRCLE ( 'NONE', #47229, 4.799999999999999822 ) ;
#6669=AXIS2_PLACEMENT_3D ( 'NONE', #20384, #38380, #55824 ) ;
#6684=ADVANCED_FACE ( 'NONE', ( #39276 ), #35111, .T. ) ;
#6685=CARTESIAN_POINT ( 'NONE',  ( -9.157500079073999544, -78.72316281358077106, 3.211059275314999795 ) ) ;
#6690=CARTESIAN_POINT ( 'NONE',  ( -7.239079175163887214, -78.65352817696454224, -5.758258266944833892 ) ) ;
#6710=CARTESIAN_POINT ( 'NONE',  ( 8.244337278279383341, -77.75611392600042393, 6.933698818737298986 ) ) ;
#6718=CARTESIAN_POINT ( 'NONE',  ( 9.250000492344584657, -78.34738994167214798, -0.3032949936654210643 ) ) ;
#6722=CARTESIAN_POINT ( 'NONE',  ( -0.5568870975076999352, -77.94963385321997862, -9.723660445896001647 ) ) ;
#6731=CARTESIAN_POINT ( 'NONE',  ( -6.447812191272999982, -78.73152414433498336, 8.972380486426999369 ) ) ;
#6741=CARTESIAN_POINT ( 'NONE',  ( 1.841371367509999857, -80.39010546013851410, -9.592189096167999196 ) ) ;
#6750=AXIS2_PLACEMENT_3D ( 'NONE', #2269, #36800, #55397 ) ;
#6755=CARTESIAN_POINT ( 'NONE',  ( 7.097510073754000004, -77.08243616160899592, 6.942687883724000919 ) ) ;
#6757=CARTESIAN_POINT ( 'NONE',  ( 2.879226727952094222, -79.74583333333333712, -10.71369944335146940 ) ) ;
#6759=CARTESIAN_POINT ( 'NONE',  ( 0.7412195098092654311, -77.02812499985410000, -9.421875000738944905 ) ) ;
#6770=CARTESIAN_POINT ( 'NONE',  ( -6.317187036472000194, -77.26057450803698146, 7.370530927706999691 ) ) ;
#6775=CARTESIAN_POINT ( 'NONE',  ( 8.270224399031000928, -77.97653256295699009, -5.144228231339999624 ) ) ;
#6778=CARTESIAN_POINT ( 'NONE',  ( -10.76076152244900364, -77.71906335555217993, -2.634765227118816444 ) ) ;
#6784=CARTESIAN_POINT ( 'NONE',  ( -8.082941148289398470, -78.05848663413912902, 4.658681804407654781 ) ) ;
#6788=CARTESIAN_POINT ( 'NONE',  ( -9.469606800734000629, -80.05752053325198858, 5.597012331546999953 ) ) ;
#6789=CARTESIAN_POINT ( 'NONE',  ( -4.409065846835999558, -79.66604063881599984, -8.482405482233000171 ) ) ;
#6792=VERTEX_POINT ( 'NONE', #54327 ) ;
#6793=CIRCLE ( 'NONE', #39764, 10.69999999999999929 ) ;
#6806=CARTESIAN_POINT ( 'NONE',  ( 0.000000000000000000, -74.64999999999999147, 0.000000000000000000 ) ) ;
#6808=ORIENTED_EDGE ( 'NONE', *, *, #50924, .F. ) ;
#6822=CARTESIAN_POINT ( 'NONE',  ( 4.865965793551021434, -77.26911405462628579, -7.870456092190766917 ) ) ;
#6831=CARTESIAN_POINT ( 'NONE',  ( 9.759566573192998362, -79.70423432486698800, -5.179648052473000419 ) ) ;
#6836=ORIENTED_EDGE ( 'NONE', *, *, #11428, .F. ) ;
#6847=CARTESIAN_POINT ( 'NONE',  ( 7.515172033767000492, -78.44568149309900207, 5.847440938983000436 ) ) ;
#6860=CARTESIAN_POINT ( 'NONE',  ( 10.71556987377000070, -79.63720544108798549, 2.374990294079000197 ) ) ;
#6864=DIRECTION ( 'NONE',  ( 0.000000000000000000, -1.000000000000000000, 0.000000000000000000 ) ) ;
#6869=CARTESIAN_POINT ( 'NONE',  ( 11.14483649738000004, -78.94088091476099578, 1.649713251514000056 ) ) ;
#6879=CONICAL_SURFACE ( 'NONE', #46524, 10.84999999997999964, 0.7853981633972997312 ) ;
#6880=( NAMED_UNIT ( * ) SI_UNIT ( $, .STERADIAN. ) SOLID_ANGLE_UNIT ( ) );
#6886=CARTESIAN_POINT ( 'NONE',  ( -1.168698982885748139, -79.86530793566201680, -9.494534496902526044 ) ) ;
#6892=DIRECTION ( 'NONE',  ( 0.000000000000000000, 1.000000000000000000, 0.000000000000000000 ) ) ;
#6896=CARTESIAN_POINT ( 'NONE',  ( 1.157835957478192457, -79.36503902903432106, 9.256249544534666640 ) ) ;
#6899=CARTESIAN_POINT ( 'NONE',  ( -9.143293663829377138, -77.58804731730369042, 1.400502067634492365 ) ) ;
#6902=CARTESIAN_POINT ( 'NONE',  ( -9.282419925074000489, -77.29339558985098790, -2.829762163499999872 ) ) ;
#6912=CONICAL_SURFACE ( 'NONE', #49306, 10.59999999997999787, 0.7853981633972997312 ) ;
#6914=CARTESIAN_POINT ( 'NONE',  ( -10.99999999999000089, -80.20000000002698926, -2.639066790267999940E-09 ) ) ;
#6919=CARTESIAN_POINT ( 'NONE',  ( -10.72134522692999958, -80.50391171894298736, -1.470872915343000020 ) ) ;
#6925=MECHANICAL_DESIGN_GEOMETRIC_PRESENTATION_REPRESENTATION('',(#38679),#50950);
#6929=CARTESIAN_POINT ( 'NONE',  ( -0.09064084131274000034, -79.83269446212499076, 9.533214929259999693 ) ) ;
#6931=DIRECTION ( 'NONE',  ( 0.000000000000000000, -1.000000000000000000, 0.000000000000000000 ) ) ;
#6938=CARTESIAN_POINT ( 'NONE',  ( -4.775172515662999828, -77.39640004304698095, -9.972254548579000399 ) ) ;
#6943=CARTESIAN_POINT ( 'NONE',  ( 4.658475568430826108, -78.33333333333332860, 8.082524092276882399 ) ) ;
#6959=EDGE_CURVE ( 'NONE', #6475, #56949, #30906, .T. ) ;
#6975=CARTESIAN_POINT ( 'NONE',  ( 3.401992325571604692, -79.69635448561501789, 9.101187944220413328 ) ) ;
#6978=CARTESIAN_POINT ( 'NONE',  ( -5.318030017779740604, -78.67642921060232197, -7.571365619617901999 ) ) ;
#6999=CARTESIAN_POINT ( 'NONE',  ( 6.768311862815361124, -77.77140864696846734, 8.380151698724020548 ) ) ;
#7003=EDGE_LOOP ( 'NONE', ( #21110, #17908 ) ) ;
#7009=CARTESIAN_POINT ( 'NONE',  ( 9.191740907676001271, -79.18591467081699875, -2.486449962426000138 ) ) ;
#7015=CARTESIAN_POINT ( 'NONE',  ( 0.000000000000000000, -81.90000000002299885, 0.000000000000000000 ) ) ;
#7016=EDGE_CURVE ( 'NONE', #46260, #26583, #35042, .T. ) ;
#7018=ORIENTED_EDGE ( 'NONE', *, *, #50852, .T. ) ;
#7019=CARTESIAN_POINT ( 'NONE',  ( 10.81514082164000001, -79.04054004199397809, -2.260668630147000258 ) ) ;
#7024=CARTESIAN_POINT ( 'NONE',  ( 9.452928397550001804, -77.41834665783399316, 6.429943439921999904 ) ) ;
#7028=B_SPLINE_CURVE_WITH_KNOTS ( 'NONE', 3,
 ( #25401, #3548, #3269, #4425, #52852, #22424, #18007, #31259, #44277, #39267, #12688, #16842, #35998, #25687, #40438, #49004, #8852, #4125, #27 ),
 .UNSPECIFIED., .F., .F.,
 ( 4, 1, 1, 1, 1, 1, 1, 1, 1, 1, 1, 1, 1, 1, 1, 1, 4 ),
 ( 0.000000000000000000, 0.04500041259816049688, 0.1100003587311620262, 0.1750003048641954329, 0.2400002509971969622, 0.3050001971301984915, 0.3700001432631362386, 0.4350000893963608117, 0.5000000355292667509, 0.5649999816621725790, 0.6299999277953972632, 0.6949998739283032023, 0.7599998200612091415, 0.8249997661944337146, 0.8899997123273396538, 0.9549996584602455929, 1.000000000000000000 ),
 .UNSPECIFIED. ) ;
#7032=CARTESIAN_POINT ( 'NONE',  ( 9.647254834573999460, -80.36767059146200154, -1.526580663425000095 ) ) ;
#7066=CARTESIAN_POINT ( 'NONE',  ( 1.889053048974999927, -78.63028063292298953, 9.554641504766999915 ) ) ;
#7074=CARTESIAN_POINT ( 'NONE',  ( -5.872569646762852535, -79.32220536973464675, -7.509559151335658100 ) ) ;
#7079=CARTESIAN_POINT ( 'NONE',  ( 9.256860190652000497, -78.81949371830199880, -1.144930063865999825 ) ) ;
#7094=CARTESIAN_POINT ( 'NONE',  ( 0.000000000000000000, -76.19999999999998863, 0.000000000000000000 ) ) ;
#7117=CARTESIAN_POINT ( 'NONE',  ( 4.265386565970945121, -77.26315468739150560, -8.207862934106792352 ) ) ;
#7126=CARTESIAN_POINT ( 'NONE',  ( -10.51276546006999979, -78.46817073422899114, 3.399949415165999689 ) ) ;
#7130=CARTESIAN_POINT ( 'NONE',  ( -8.937783764417927657, -77.19999999999998863, 6.271596724013802415 ) ) ;
#7132=DIRECTION ( 'NONE',  ( 0.000000000000000000, -1.000000000000000000, 0.000000000000000000 ) ) ;
#7138=CARTESIAN_POINT ( 'NONE',  ( 9.333674174720000494, -77.87720491051898364, -1.884914489352999878 ) ) ;
#7149=CARTESIAN_POINT ( 'NONE',  ( -9.438868967565998247, -79.41246660642698885, -5.601050722391000214 ) ) ;
#7156=ORIENTED_EDGE ( 'NONE', *, *, #46008, .T. ) ;
#7158=CARTESIAN_POINT ( 'NONE',  ( -9.250000000000000000, -77.99999999999998579, 0.000000000000000000 ) ) ;
#7160=CARTESIAN_POINT ( 'NONE',  ( 8.456503675551001464, -78.04961660823299496, 7.278678959607000287 ) ) ;
#7170=DIRECTION ( 'NONE',  ( -1.000000000000000000, 0.000000000000000000, 0.000000000000000000 ) ) ;
#7172=SHAPE_REPRESENTATION_RELATIONSHIP ( 'NONE' , 'NONE' ,  #46016, #42678 ) ;
#7174=VERTEX_POINT ( 'NONE', #41253 ) ;
#7177=ORIENTED_EDGE ( 'NONE', *, *, #5835, .T. ) ;
#7184=CARTESIAN_POINT ( 'NONE',  ( -2.794094295877650680, -78.20065386029028787, -8.819927633509278664 ) ) ;
#7185=CARTESIAN_POINT ( 'NONE',  ( 8.040680144505948590, -79.29236773697583374, 4.729291971201980971 ) ) ;
#7189=CARTESIAN_POINT ( 'NONE',  ( -3.808885479938491248, -77.50893336096748953, 8.432746257839983883 ) ) ;
#7192=CARTESIAN_POINT ( 'NONE',  ( -9.702231720816998362, -78.83173763022898584, -0.1934140619087000024 ) ) ;
#7196=CARTESIAN_POINT ( 'NONE',  ( 7.117135278674999732, -80.13006704345897901, 8.718833803912000135 ) ) ;
#7205=CARTESIAN_POINT ( 'NONE',  ( 5.799999999999999822, -80.99999999999998579, 0.000000000000000000 ) ) ;
#7207=CARTESIAN_POINT ( 'NONE',  ( -4.999999999872000167, -80.49999999987198862, 4.857408280386999624E-10 ) ) ;
#7211=CONICAL_SURFACE ( 'NONE', #11938, 4.199999999676998996, 0.7853981633972997312 ) ;
#7219=CARTESIAN_POINT ( 'NONE',  ( 3.008644551092000352, -79.24281087269798718, 9.161133607876998042 ) ) ;
#7221=CARTESIAN_POINT ( 'NONE',  ( -7.540108831187442462, -79.40412807809049411, -6.127962695274685956 ) ) ;
#7224=CARTESIAN_POINT ( 'NONE',  ( -11.00000000000000000, -77.19999999999998863, 5.688460190305999883E-13 ) ) ;
#7226=CARTESIAN_POINT ( 'NONE',  ( 7.984952588555000119, -77.99615392501999622, -7.647802602006999351 ) ) ;
#7231=CARTESIAN_POINT ( 'NONE',  ( -0.5065222552852000071, -77.08871499676898509, 9.658707080791000266 ) ) ;
#7234=DIRECTION ( 'NONE',  ( 0.000000000000000000, 1.000000000000000000, 0.000000000000000000 ) ) ;
#7242=ADVANCED_FACE ( 'NONE', ( #19848, #988 ), #54977, .F. ) ;
#7244=ORIENTED_EDGE ( 'NONE', *, *, #36701, .T. ) ;
#7267=CARTESIAN_POINT ( 'NONE',  ( 0.9440756146772367741, -79.98258690118150582, -9.563528426713427066 ) ) ;
#7270=CARTESIAN_POINT ( 'NONE',  ( -6.009140664802340659, -78.66887010198279029, -7.034215166533324570 ) ) ;
#7298=CARTESIAN_POINT ( 'NONE',  ( -2.166619587182999851, -77.78611896097199008, 9.383974079751000730 ) ) ;
#7309=CARTESIAN_POINT ( 'NONE',  ( -11.05562359778000214, -79.85724572043098135, 1.903787264327999829 ) ) ;
#7311=ADVANCED_FACE ( 'NONE', ( #47608 ), #25133, .T. ) ;
#7316=CARTESIAN_POINT ( 'NONE',  ( 8.985706068735000329, -79.84810805933004474, -3.828549499589000149 ) ) ;
#7334=CARTESIAN_POINT ( 'NONE',  ( -2.421167930323375295, -77.89583333333331439, 9.009247259181911716 ) ) ;
#7337=AXIS2_PLACEMENT_3D ( 'NONE', #54988, #14536, #20151 ) ;
#7345=CARTESIAN_POINT ( 'NONE',  ( -0.8153671514888000127, -77.13888932676817944, -9.346629228026998248 ) ) ;
#7351=CARTESIAN_POINT ( 'NONE',  ( 1.492456682423999981, -77.40805598037698587, -9.624565956529000488 ) ) ;
#7356=EDGE_LOOP ( 'NONE', ( #54217, #9280, #21038, #49196 ) ) ;
#7360=CARTESIAN_POINT ( 'NONE',  ( -9.499053022854020867, -79.25075071779494351, -0.08961454088966377962 ) ) ;
#7364=CARTESIAN_POINT ( 'NONE',  ( 3.258261448710999986, -80.11910146897098173, 9.339172452763000010 ) ) ;
#7366=CARTESIAN_POINT ( 'NONE',  ( -9.250000000000000000, -78.99999999999998579, 0.000000000000000000 ) ) ;
#7380=CARTESIAN_POINT ( 'NONE',  ( -4.373213035511999358, -79.29760296238899286, -8.733596771889999388 ) ) ;
#7388=CARTESIAN_POINT ( 'NONE',  ( 5.539808784079868431, -77.53333333333331723, 9.611650271896850839 ) ) ;
#7395=B_SPLINE_CURVE_WITH_KNOTS ( 'NONE', 3,
 ( #16226, #25361, #57522, #48115, #44240, #34206, #29774, #52243, #43377, #57239, #11799, #2936, #20935, #38937, #16514, #34496, #43672, #3230, #21221, #39226, #16803, #52812, #18846, #31515, #8808, #49563, #41276, #45727 ),
 .UNSPECIFIED., .F., .F.,
 ( 4, 2, 2, 2, 2, 1, 2, 2, 1, 2, 2, 2, 2, 2, 4 ),
 ( 0.000000000000000000, 0.06249999999999986122, 0.1249999999999997224, 0.2499999999999994449, 0.3749999999999991673, 0.4374999999999991118, 0.4687499999999991118, 0.4999999999999991118, 0.5624999999999994449, 0.5937499999999994449, 0.6249999999999994449, 0.7499999999999996669, 0.8124999999999997780, 0.8749999999999997780, 1.000000000000000000 ),
 .UNSPECIFIED. ) ;
#7396=CARTESIAN_POINT ( 'NONE',  ( -0.7274841066961533764, -79.98136092145524856, 9.221286261669808582 ) ) ;
#7400=CARTESIAN_POINT ( 'NONE',  ( 9.951586773259000651, -79.83198580643298214, -5.281558014135000256 ) ) ;
#7401=CARTESIAN_POINT ( 'NONE',  ( 9.249992181567158411, -77.35008848816909222, 0.01013385650330413286 ) ) ;
#7413=CARTESIAN_POINT ( 'NONE',  ( 0.9151062594318000176, -78.86146369488598395, 11.01092521911999889 ) ) ;
#7419=CARTESIAN_POINT ( 'NONE',  ( -1.156736691641969017, -77.19999999999998863, 10.75377114862106787 ) ) ;
#7425=CONICAL_SURFACE ( 'NONE', #38529, 1.099999997149000430, 0.7853981633972997312 ) ;
#7428=CARTESIAN_POINT ( 'NONE',  ( -8.606866362194999454, -77.67823810661599282, -4.073355822332000109 ) ) ;
#7436=CARTESIAN_POINT ( 'NONE',  ( -1.210822168571097146, -78.88541666666667140, 9.249999999999992895 ) ) ;
#7442=CARTESIAN_POINT ( 'NONE',  ( 3.176617583302000281, -79.72148250408599779, 10.50586082162000068 ) ) ;
#7453=CARTESIAN_POINT ( 'NONE',  ( 6.788068531828999497, -79.50272800141398477, 8.991721824839000732 ) ) ;
#7470=ORIENTED_EDGE ( 'NONE', *, *, #55973, .T. ) ;
#7475=CARTESIAN_POINT ( 'NONE',  ( 1.142746755879123777, -78.23489730971330403, -9.184199345809689774 ) ) ;
#7479=CARTESIAN_POINT ( 'NONE',  ( -7.060961830176961662, -77.54418585273785425, 5.975330936113271818 ) ) ;
#7480=CARTESIAN_POINT ( 'NONE',  ( 2.386167682861000117, -77.16720924082279964, 10.77916482977000001 ) ) ;
#7482=CARTESIAN_POINT ( 'NONE',  ( 5.091895231007000255, -78.66119465545499168, 8.260951054388000259 ) ) ;
#7487=CARTESIAN_POINT ( 'NONE',  ( -7.054457466615000172, -80.44093696116098613, -8.769379688592000122 ) ) ;
#7499=CARTESIAN_POINT ( 'NONE',  ( -10.89465136399999956, -79.97499423886398517, 2.517158085631999942 ) ) ;
#7502=CARTESIAN_POINT ( 'NONE',  ( 2.421239052663348268, -79.74628264568268321, -9.008702010510926783 ) ) ;
#7510=CARTESIAN_POINT ( 'NONE',  ( -6.657338106343000383, -79.45823032903800254, 6.671287216456999403 ) ) ;
#7513=CARTESIAN_POINT ( 'NONE',  ( 9.250000000000000000, -79.34999999999999432, 0.000000000000000000 ) ) ;
#7514=DIRECTION ( 'NONE',  ( 0.000000000000000000, -1.000000000000000000, 0.000000000000000000 ) ) ;
#7519=CARTESIAN_POINT ( 'NONE',  ( 0.9847086833720000154, -77.93903450768898722, -11.01265208048999966 ) ) ;
#7524=CARTESIAN_POINT ( 'NONE',  ( 9.100722152916000951, -76.99236172063068295, -3.274758550341999808 ) ) ;
#7525=CARTESIAN_POINT ( 'NONE',  ( -4.658475568430831437, -78.41666666666665719, 8.082524092276877070 ) ) ;
#7543=EDGE_LOOP ( 'NONE', ( #21464, #37603, #20753, #46193 ) ) ;
#7545=CARTESIAN_POINT ( 'NONE',  ( 5.684557159767975598, -79.67708333333332860, -7.396918292183157106 ) ) ;
#7552=AXIS2_PLACEMENT_3D ( 'NONE', #19897, #24321, #28142 ) ;
#7559=CARTESIAN_POINT ( 'NONE',  ( -9.221951647947621566, -78.60624782743785488, -0.7198726630268430515 ) ) ;
#7561=CARTESIAN_POINT ( 'NONE',  ( -10.99980394231345926, -80.10023817985064909, 1.711188753626703361E-06 ) ) ;
#7570=EDGE_CURVE ( 'NONE', #27444, #47291, #43657, .T. ) ;
#7577=CARTESIAN_POINT ( 'NONE',  ( -8.631379868284000167, -78.25656186178198936, 6.779623747090999686 ) ) ;
#7583=EDGE_CURVE ( 'NONE', #56496, #21107, #56225, .T. ) ;
#7587=CARTESIAN_POINT ( 'NONE',  ( 7.515172033767000492, -78.75955723388199203, 5.847440938983000436 ) ) ;
#7589=CARTESIAN_POINT ( 'NONE',  ( 0.000000000000000000, -80.99999999999998579, 0.000000000000000000 ) ) ;
#7592=FACE_OUTER_BOUND ( 'NONE', #49775, .T. ) ;
#7593=CARTESIAN_POINT ( 'NONE',  ( -9.611650271896840181, -78.74166666666666003, -5.539808784079887083 ) ) ;
#7598=CARTESIAN_POINT ( 'NONE',  ( 3.968454646034999644, -79.96041464100198937, -10.61226005143999984 ) ) ;
#7602=ORIENTED_EDGE ( 'NONE', *, *, #35746, .T. ) ;
#7605=CARTESIAN_POINT ( 'NONE',  ( 9.226480760116999136, -79.36101818546501363, -2.263195259622999611 ) ) ;
#7632=CARTESIAN_POINT ( 'NONE',  ( 5.388524986465999866, -77.28388852172999179, 7.812415235880998843 ) ) ;
#7637=CARTESIAN_POINT ( 'NONE',  ( -9.549999999999998934, -76.39999999999999147, 0.000000000000000000 ) ) ;
#7638=LINE ( 'NONE', #43949, #34484 ) ;
#7641=CARTESIAN_POINT ( 'NONE',  ( 0.000000000000000000, -78.59999999921299718, 0.000000000000000000 ) ) ;
#7645=CARTESIAN_POINT ( 'NONE',  ( -5.226977690307169411, -79.32879368366329231, -7.969415024645670087 ) ) ;
#7650=CARTESIAN_POINT ( 'NONE',  ( 7.832365237661001345, -79.90583509515599303, -5.858077979548999892 ) ) ;
#7669=ORIENTED_EDGE ( 'NONE', *, *, #11311, .F. ) ;
#7675=EDGE_CURVE ( 'NONE', #51092, #54228, #24532, .T. ) ;
#7676=CARTESIAN_POINT ( 'NONE',  ( 1.439896632895284911, -77.56458333333331723, 11.00000000000000355 ) ) ;
#7679=EDGE_CURVE ( 'NONE', #26583, #3255, #13471, .T. ) ;
#7684=CARTESIAN_POINT ( 'NONE',  ( 5.046009951596436949, -79.92957980094915627, 7.753141342909813716 ) ) ;
#7686=DIRECTION ( 'NONE',  ( 0.000000000000000000, -1.000000000000000000, 0.000000000000000000 ) ) ;
#7687=ORIENTED_EDGE ( 'NONE', *, *, #43777, .F. ) ;
#7688=CARTESIAN_POINT ( 'NONE',  ( 3.260743090391000187, -79.97244757809599491, 10.78408470153000032 ) ) ;
#7689=CARTESIAN_POINT ( 'NONE',  ( 7.496060297333964506, -77.30026476220074017, -5.419471789427347197 ) ) ;
#7691=CARTESIAN_POINT ( 'NONE',  ( 0.000000000000000000, -80.99999999999998579, 5.800000000000029132 ) ) ;
#7694=DIRECTION ( 'NONE',  ( 0.000000000000000000, -1.000000000000000000, 0.000000000000000000 ) ) ;
#7696=CARTESIAN_POINT ( 'NONE',  ( -9.611650271896857944, -78.55833333333332291, 5.539808784079855997 ) ) ;
#7699=CARTESIAN_POINT ( 'NONE',  ( 0.000000000000000000, -75.10000000032299283, 0.000000000000000000 ) ) ;
#7700=CARTESIAN_POINT ( 'NONE',  ( -9.663285910017000546, -79.51527887665599792, 5.577858467032999812 ) ) ;
#7704=DIRECTION ( 'NONE',  ( 0.000000000000000000, -1.000000000000000000, 0.000000000000000000 ) ) ;
#7705=ORIENTED_EDGE ( 'NONE', *, *, #14252, .F. ) ;
#7716=CARTESIAN_POINT ( 'NONE',  ( 8.857396897828001769, -77.30170024541499174, -3.187116989308000026 ) ) ;
#7727=CARTESIAN_POINT ( 'NONE',  ( 9.028681611143001717, -78.13370064223998668, -5.970393136294000591 ) ) ;
#7729=CARTESIAN_POINT ( 'NONE',  ( 2.836859645505057426, -80.35885416666536685, 10.55930595257627047 ) ) ;
#7735=CARTESIAN_POINT ( 'NONE',  ( 3.549246799458173118, -77.34368329502935069, 8.572692145709080336 ) ) ;
#7736=CARTESIAN_POINT ( 'NONE',  ( 5.684557159767946288, -78.17708333333332860, -7.396918292183178423 ) ) ;
#7739=CARTESIAN_POINT ( 'NONE',  ( -10.85153605587000136, -79.66191800929898648, 2.386335476490000218 ) ) ;
#7749=ORIENTED_EDGE ( 'NONE', *, *, #38374, .T. ) ;
#7761=CARTESIAN_POINT ( 'NONE',  ( 1.464740467520374123, -78.23771836109808930, -9.139813437711902466 ) ) ;
#7766=CARTESIAN_POINT ( 'NONE',  ( -6.071607140531662061, -77.53210482738238341, 6.979269262791448547 ) ) ;
#7767=CARTESIAN_POINT ( 'NONE',  ( -0.5413127449341000874, -77.93064224879100266, -11.02683867434999954 ) ) ;
#7770=CARTESIAN_POINT ( 'NONE',  ( -5.159044788988000008, -77.35024324810899543, -8.219183903844999861 ) ) ;
#7774=CARTESIAN_POINT ( 'NONE',  ( -10.49924843836999955, -80.45947872149298519, -4.054558598941000014 ) ) ;
#7791=ORIENTED_EDGE ( 'NONE', *, *, #45287, .T. ) ;
#7792=DIRECTION ( 'NONE',  ( 0.000000000000000000, -1.000000000000000000, -8.830898975038999242E-14 ) ) ;
#7796=CARTESIAN_POINT ( 'NONE',  ( -7.548024343608999764, -80.07190615245599474, -5.643896870619999895 ) ) ;
#7799=CARTESIAN_POINT ( 'NONE',  ( 10.49438680834578719, -77.32500000000000284, -3.407966307000451334 ) ) ;
#7804=CIRCLE ( 'NONE', #40796, 5.500000000000000000 ) ;
#7805=CARTESIAN_POINT ( 'NONE',  ( -1.989802025464000090, -77.26035782317299550, 10.76548307208999944 ) ) ;
#7812=CARTESIAN_POINT ( 'NONE',  ( -5.539808784079933268, -77.51666666666667993, 9.611650271896811759 ) ) ;
#7822=LINE ( 'NONE', #57413, #22367 ) ;
#7838=CARTESIAN_POINT ( 'NONE',  ( -5.159044788988000008, -77.33039518626078745, -8.219183903844999861 ) ) ;
#7840=EDGE_CURVE ( 'NONE', #604, #4986, #39890, .T. ) ;
#7842=CARTESIAN_POINT ( 'NONE',  ( -1.439896632895359962, -78.58541666666666003, 10.99999999999999645 ) ) ;
#7844=EDGE_CURVE ( 'NONE', #21107, #27560, #3216, .T. ) ;
#7849=CARTESIAN_POINT ( 'NONE',  ( -10.98916705908266778, -80.10458660312347945, -0.5762717334662600388 ) ) ;
#7864=CARTESIAN_POINT ( 'NONE',  ( -11.00000000000000000, -79.71041666666664582, -1.439896632895322881 ) ) ;
#7868=CARTESIAN_POINT ( 'NONE',  ( -9.497876546326999403, -77.35168256874098347, -0.2008509664869000122 ) ) ;
#7872=CARTESIAN_POINT ( 'NONE',  ( 9.480930971721999612, -79.21433849994599541, 0.8843128721991000418 ) ) ;
#7877=CARTESIAN_POINT ( 'NONE',  ( -4.687312336529864787, -79.01734543862330895, 8.066552816164486828 ) ) ;
#7881=CARTESIAN_POINT ( 'NONE',  ( 8.838457456548999502, -78.57066105045699089, -6.447440276951000193 ) ) ;
#7884=CARTESIAN_POINT ( 'NONE',  ( -3.482343428915000150, -80.46974281206399837, -10.30556169736999905 ) ) ;
#7891=ADVANCED_FACE ( 'NONE', ( #20352 ), #6912, .T. ) ;
#7900=CARTESIAN_POINT ( 'NONE',  ( 7.000000000000000000, -80.99999999999998579, 0.000000000000000000 ) ) ;
#7911=CARTESIAN_POINT ( 'NONE',  ( 0.000000000000000000, -81.10000000285099020, 7.000000000000000000 ) ) ;
#7913=CARTESIAN_POINT ( 'NONE',  ( 5.155010784763280007, -79.93646688885499429, 9.790528303537310961 ) ) ;
#7918=CARTESIAN_POINT ( 'NONE',  ( -3.524583092881000024, -77.36221662263500320, 8.811773852426000531 ) ) ;
#7932=CARTESIAN_POINT ( 'NONE',  ( 6.206556651784778111, -79.06848936835629615, 7.218217299451517022 ) ) ;
#7934=CARTESIAN_POINT ( 'NONE',  ( 2.879226727952049814, -78.95416666666666572, 10.71369944335148183 ) ) ;
#7936=CARTESIAN_POINT ( 'NONE',  ( 5.771514257604000164, -79.59623425335998093, 8.032758792294998784 ) ) ;
#7938=FACE_OUTER_BOUND ( 'NONE', #37656, .T. ) ;
#7947=EDGE_LOOP ( 'NONE', ( #6301, #19384, #42979, #47826 ) ) ;
#7948=CARTESIAN_POINT ( 'NONE',  ( 0.5713819827555001174, -77.30008885281499431, 11.08689227811000144 ) ) ;
#7954=AXIS2_PLACEMENT_3D ( 'NONE', #9859, #37289, #735 ) ;
#7956=FACE_OUTER_BOUND ( 'NONE', #4926, .T. ) ;
#7963=ORIENTED_EDGE ( 'NONE', *, *, #34007, .T. ) ;
#7973=CARTESIAN_POINT ( 'NONE',  ( 1.425295968735332597, -79.96318692083401913, 9.139224115734268850 ) ) ;
#7977=CARTESIAN_POINT ( 'NONE',  ( 5.445998289199994957, -77.27523227367147740, -7.476759099558663912 ) ) ;
#7985=CARTESIAN_POINT ( 'NONE',  ( -9.875985572548097835, -80.44999999999996021, -4.392572548244121577 ) ) ;
#7986=CARTESIAN_POINT ( 'NONE',  ( -11.08844420678000020, -79.06580120733299566, -1.240163186867999867 ) ) ;
#7993=CARTESIAN_POINT ( 'NONE',  ( -7.154810283782063962, -77.19999999999998863, 8.208487408017942855 ) ) ;
#8012=CARTESIAN_POINT ( 'NONE',  ( 0.1291013223160000223, -79.30421540610097964, 10.97485077029999978 ) ) ;
#8021=DIRECTION ( 'NONE',  ( -1.000000000000000000, 0.000000000000000000, 0.000000000000000000 ) ) ;
#8023=CARTESIAN_POINT ( 'NONE',  ( 10.34967326289000056, -78.08539999468298731, 3.868085496227999798 ) ) ;
#8024=CARTESIAN_POINT ( 'NONE',  ( -10.69999999999999929, -80.49999999999998579, 0.000000000000000000 ) ) ;
#8044=CARTESIAN_POINT ( 'NONE',  ( -6.534469237059214564, -78.16274746009533203, -6.546848636492562434 ) ) ;
#8050=CARTESIAN_POINT ( 'NONE',  ( -7.383570525523341921, -77.54854952769156284, 5.573145937136878558 ) ) ;
#8051=CARTESIAN_POINT ( 'NONE',  ( 2.386167682861000117, -77.22751216649398032, 10.77916482977000001 ) ) ;
#8054=CARTESIAN_POINT ( 'NONE',  ( -1.959694873104000257, -77.37866707723799209, -9.504225410855001499 ) ) ;
#8058=CARTESIAN_POINT ( 'NONE',  ( 1.791008777272000030, -80.17182820879699534, 11.11143388882000060 ) ) ;
#8061=CARTESIAN_POINT ( 'NONE',  ( 7.396918292183175758, -78.69791666666665719, -5.684557159767951617 ) ) ;
#8062=ORIENTED_EDGE ( 'NONE', *, *, #14950, .T. ) ;
#8067=CARTESIAN_POINT ( 'NONE',  ( -8.082088197687879116, -78.55834743794827091, 4.658190788286820982 ) ) ;
#8075=CARTESIAN_POINT ( 'NONE',  ( 6.760013919724038978, -80.02291666667453285, 8.796335266380001627 ) ) ;
#8082=CARTESIAN_POINT ( 'NONE',  ( 2.977199900158871149, -78.09769602762067109, -10.42248997560320056 ) ) ;
#8083=CARTESIAN_POINT ( 'NONE',  ( -5.018480251613000043, -80.10112881071398760, -7.977531891197001457 ) ) ;
#8093=CARTESIAN_POINT ( 'NONE',  ( 9.499178638196321245, -79.00092112126561972, 0.1004274591880019996 ) ) ;
#8098=CARTESIAN_POINT ( 'NONE',  ( -3.591972190522999764, -77.17512728940789657, 8.980252640667000463 ) ) ;
#8120=CARTESIAN_POINT ( 'NONE',  ( -6.065106684382000068, -77.27128372030617243, 9.224892016835999797 ) ) ;
#8125=LINE ( 'NONE', #40294, #28207 ) ;
#8137=CARTESIAN_POINT ( 'NONE',  ( -9.109849427410853906, -78.61403873330360170, -1.603955441074990995 ) ) ;
#8151=CARTESIAN_POINT ( 'NONE',  ( 11.00000000000000000, -79.44999999999998863, 0.000000000000000000 ) ) ;
#8155=CARTESIAN_POINT ( 'NONE',  ( -5.755176823513999729, -78.22846950744899175, 9.345691860246999383 ) ) ;
#8160=CARTESIAN_POINT ( 'NONE',  ( -9.497662397991334160, -77.31834923540763782, -0.2008463566140032963 ) ) ;
#8161=CARTESIAN_POINT ( 'NONE',  ( 8.266198729575041426, -76.95520833333529254, -4.776057930356138570 ) ) ;
#8164=CARTESIAN_POINT ( 'NONE',  ( 9.630178197611998669, -77.64399981532699258, 0.1134805908624000048 ) ) ;
#8170=CARTESIAN_POINT ( 'NONE',  ( -9.191600602562143507, -79.08998696896227898, 1.206688570074718969 ) ) ;
#8175=CARTESIAN_POINT ( 'NONE',  ( -4.263934386054000214, -78.96395401111398371, -10.07505235160000012 ) ) ;
#8178=CARTESIAN_POINT ( 'NONE',  ( -8.802519067788999507, -80.25274279837199742, 7.133338619267999725 ) ) ;
#8183=EDGE_LOOP ( 'NONE', ( #48961, #58303, #34680, #34060 ) ) ;
#8208=CARTESIAN_POINT ( 'NONE',  ( 5.056474866540000335, -77.19110806070449371, -7.902943353631999734 ) ) ;
#8213=CARTESIAN_POINT ( 'NONE',  ( 0.000000000000000000, -77.19999999999998863, 0.000000000000000000 ) ) ;
#8222=CARTESIAN_POINT ( 'NONE',  ( -4.285131888247867060, -79.16215997888556899, 8.500474416186351689 ) ) ;
#8224=CARTESIAN_POINT ( 'NONE',  ( -11.00000000000000000, -79.09999999999999432, 0.000000000000000000 ) ) ;
#8226=CARTESIAN_POINT ( 'NONE',  ( 7.724294138338000160, -79.00949129696499540, 5.999925182671999480 ) ) ;
#8244=CARTESIAN_POINT ( 'NONE',  ( 9.534323188421000239, -79.01153086664199066, -1.008198710029000189 ) ) ;
#8246=VECTOR ( 'NONE', #10158, 1000.000000000000000 ) ;
#8256=AXIS2_PLACEMENT_3D ( 'NONE', #20300, #37715, #55737 ) ;
#8263=CARTESIAN_POINT ( 'NONE',  ( -2.226953637271548825, -79.99461437525772567, 9.002238948001519248 ) ) ;
#8265=EDGE_LOOP ( 'NONE', ( #22869, #31244, #57323, #16233 ) ) ;
#8274=CARTESIAN_POINT ( 'NONE',  ( -6.511242784100999437, -78.98152414433498336, 9.060646613982999753 ) ) ;
#8301=CARTESIAN_POINT ( 'NONE',  ( 10.94409238582999855, -78.68618361078299017, 0.8311789410725000105 ) ) ;
#8310=CARTESIAN_POINT ( 'NONE',  ( 10.86862532138017912, -77.93584017775066286, -1.957230818804968520 ) ) ;
#8312=CARTESIAN_POINT ( 'NONE',  ( -10.99582742793000101, -79.22949549020498239, 1.892981466416000069 ) ) ;
#8313=CARTESIAN_POINT ( 'NONE',  ( 7.000000000000000000, -81.19999999999998863, -1.000000000000000000 ) ) ;
#8318=CARTESIAN_POINT ( 'NONE',  ( -9.469606800734000629, -79.65752053325199711, 5.597012331546999953 ) ) ;
#8331=CARTESIAN_POINT ( 'NONE',  ( -9.235030002071850319, -78.10620107062753448, -0.6966500853201260668 ) ) ;
#8335=CARTESIAN_POINT ( 'NONE',  ( -4.200795967633649042, -77.51264282153384499, 8.241008886275963619 ) ) ;
#8339=CARTESIAN_POINT ( 'NONE',  ( 9.512131559252001267, -78.12459716941698673, -1.920953556448999899 ) ) ;
#8344=CARTESIAN_POINT ( 'NONE',  ( 7.117135278674999732, -80.25067289479999033, 8.718833803912000135 ) ) ;
#8347=CARTESIAN_POINT ( 'NONE',  ( 2.421167930323352646, -78.64583333333331439, -9.009247259181915268 ) ) ;
#8353=CARTESIAN_POINT ( 'NONE',  ( -9.250000000000000000, -78.59999999999999432, 0.000000000000000000 ) ) ;
#8356=CARTESIAN_POINT ( 'NONE',  ( 10.89190632572000084, -80.28569813701800229, -2.978178067245000005 ) ) ;
#8360=CARTESIAN_POINT ( 'NONE',  ( 2.879226727952050258, -80.05416666667792924, 10.71369944335148361 ) ) ;
#8395=ORIENTED_EDGE ( 'NONE', *, *, #57426, .F. ) ;
#8405=CARTESIAN_POINT ( 'NONE',  ( 10.69999999997999929, -81.80000000002199556, -2.760617010408999913E-10 ) ) ;
#8419=CARTESIAN_POINT ( 'NONE',  ( -9.210376165418230343, -78.60745015110788358, -0.8564966472666962760 ) ) ;
#8429=B_SPLINE_CURVE_WITH_KNOTS ( 'NONE', 3,
 ( #35743, #40480, #18052, #44912, #58193, #36044, #53774, #16889, #49347, #4469, #12167, #30153, #26308, #48204, #34870, #21307, #7735, #52901, #12450, #48476, #3879, #39886, #5622, #10354, #54068, #49938, #50225, #19500, #54928, #36917 ),
 .UNSPECIFIED., .F., .F.,
 ( 4, 2, 2, 2, 2, 2, 2, 2, 2, 2, 2, 2, 2, 2, 4 ),
 ( 0.000000000000000000, 0.06250000000000001388, 0.1250000000000000278, 0.1875000000000000555, 0.2500000000000000555, 0.3125000000000000555, 0.3750000000000001110, 0.4375000000000001110, 0.5000000000000001110, 0.6250000000000001110, 0.6875000000000001110, 0.7500000000000002220, 0.8750000000000001110, 0.9375000000000001110, 1.000000000000000000 ),
 .UNSPECIFIED. ) ;
#8434=CARTESIAN_POINT ( 'NONE',  ( 0.000000000000000000, -81.79999999999998295, 0.000000000000000000 ) ) ;
#8441=CARTESIAN_POINT ( 'NONE',  ( 9.468749999988999022, -76.98125000001098783, 2.084568677130999610E-09 ) ) ;
#8445=CARTESIAN_POINT ( 'NONE',  ( 9.400066902809999903, -78.76658531640698868, -0.4999367261865000356 ) ) ;
#8454=ORIENTED_EDGE ( 'NONE', *, *, #48239, .T. ) ;
#8457=CARTESIAN_POINT ( 'NONE',  ( -1.662118031109000027, -80.35591171894299123, -10.80109114220999977 ) ) ;
#8469=ORIENTED_EDGE ( 'NONE', *, *, #17541, .T. ) ;
#8479=CARTESIAN_POINT ( 'NONE',  ( 9.072454766260275250, -78.83445074300934152, -1.803379576545697471 ) ) ;
#8480=VECTOR ( 'NONE', #25913, 1000.000000000000000 ) ;
#8486=CARTESIAN_POINT ( 'NONE',  ( 5.800000004703999679, -81.00000000470399186, -2.775962740116999943E-08 ) ) ;
#8500=AXIS2_PLACEMENT_3D ( 'NONE', #37722, #1443, #14404 ) ;
#8501=CARTESIAN_POINT ( 'NONE',  ( 0.000000000000000000, -80.49999999999998579, 0.000000000000000000 ) ) ;
#8512=CARTESIAN_POINT ( 'NONE',  ( -3.035968726241000226, -79.60705382909299033, 9.297629541271000164 ) ) ;
#8514=DIRECTION ( 'NONE',  ( 0.000000000000000000, -1.000000000000000000, 0.000000000000000000 ) ) ;
#8516=FACE_OUTER_BOUND ( 'NONE', #34455, .T. ) ;
#8528=VERTEX_POINT ( 'NONE', #52597 ) ;
#8533=CARTESIAN_POINT ( 'NONE',  ( 1.841371367509999857, -79.97024400411599743, -9.592189096167999196 ) ) ;
#8554=CARTESIAN_POINT ( 'NONE',  ( 0.1325202778310999863, -79.49487755444098980, 11.26549478459000042 ) ) ;
#8563=CARTESIAN_POINT ( 'NONE',  ( -9.975891578018998729, -79.09389356166599327, -4.997317968730000004 ) ) ;
#8590=CARTESIAN_POINT ( 'NONE',  ( 7.788493169598000421, -78.74236831944799064, 7.733265204867000087 ) ) ;
#8602=CARTESIAN_POINT ( 'NONE',  ( 3.980415848809999879, -79.08903371854199804, 10.42342982551999953 ) ) ;
#8607=ORIENTED_EDGE ( 'NONE', *, *, #3416, .T. ) ;
#8615=CARTESIAN_POINT ( 'NONE',  ( 4.100000000000000533, -78.69999999999998863, 0.000000000000000000 ) ) ;
#8629=CARTESIAN_POINT ( 'NONE',  ( -0.003491213567336264294, -77.47518361382161345, 9.249907303942231707 ) ) ;
#8630=CARTESIAN_POINT ( 'NONE',  ( -9.177034484502000211, -77.32294129249000036, 6.137278520473000043 ) ) ;
#8633=CARTESIAN_POINT ( 'NONE',  ( -6.473047519705999342, -78.32356397331999176, 7.229824698717000508 ) ) ;
#8637=CARTESIAN_POINT ( 'NONE',  ( 10.52776997023000050, -80.26921465513198939, 3.979665013433000720 ) ) ;
#8642=CARTESIAN_POINT ( 'NONE',  ( -9.250000000000001776, -78.51041666666667140, -1.210822168571065616 ) ) ;
#8649=CARTESIAN_POINT ( 'NONE',  ( -4.658533681657620384, -78.51668711297222103, 8.082509443235778690 ) ) ;
#8652=CARTESIAN_POINT ( 'NONE',  ( -9.013126759186999237, -80.17326805110798205, -6.983032781201999661 ) ) ;
#8656=CARTESIAN_POINT ( 'NONE',  ( -10.71369944335148361, -80.17916666669142955, 2.879226727952040044 ) ) ;
#8657=EDGE_LOOP ( 'NONE', ( #48517, #17412, #3410, #29533 ) ) ;
#8662=CARTESIAN_POINT ( 'NONE',  ( 3.299939911277999460, -79.86734754465000208, 8.828171983641000864 ) ) ;
#8675=CARTESIAN_POINT ( 'NONE',  ( 9.670530767802999250, -77.07877401326959443, -0.1674091926992999912 ) ) ;
#8684=CARTESIAN_POINT ( 'NONE',  ( 11.00000000000000711, -79.36041666666665151, 1.439896632895290240 ) ) ;
#8690=ORIENTED_EDGE ( 'NONE', *, *, #21945, .F. ) ;
#8694=CARTESIAN_POINT ( 'NONE',  ( -7.179058446791997561, -79.91995496524606324, -8.667882172381000672 ) ) ;
#8702=CARTESIAN_POINT ( 'NONE',  ( 10.65102452230999930, -77.62119051562517313, 2.905137941167998950 ) ) ;
#8710=CARTESIAN_POINT ( 'NONE',  ( -5.351292223237999579, -77.63102627198600203, 8.095330809056001442 ) ) ;
#8740=CARTESIAN_POINT ( 'NONE',  ( -2.858407197967999913, -77.19999999999998863, -8.797272775729998884 ) ) ;
#8743=CARTESIAN_POINT ( 'NONE',  ( 9.403616370364000332, -78.21950448043199344, 1.497456306884999977 ) ) ;
#8757=DIRECTION ( 'NONE',  ( 7.074021373685000131E-10, -1.000000000000000000, 4.749368372333999376E-10 ) ) ;
#8758=EDGE_LOOP ( 'NONE', ( #17300, #15234, #55091 ) ) ;
#8760=ORIENTED_EDGE ( 'NONE', *, *, #54521, .F. ) ;
#8768=ORIENTED_EDGE ( 'NONE', *, *, #2161, .F. ) ;
#8782=CARTESIAN_POINT ( 'NONE',  ( 5.684625949311768345, -77.77723352849264415, -7.397146152607679603 ) ) ;
#8786=CARTESIAN_POINT ( 'NONE',  ( -9.611650271896857944, -78.05833333333333712, 5.539808784079855997 ) ) ;
#8788=CARTESIAN_POINT ( 'NONE',  ( 4.054145691792255590, -79.94511357774049998, 10.29526509435834214 ) ) ;
#8808=CARTESIAN_POINT ( 'NONE',  ( -8.942878731355392574, -80.00000000000000000, -2.529715217048958742 ) ) ;
#8811=CARTESIAN_POINT ( 'NONE',  ( 10.71369944335146762, -78.87083333333333712, 2.879226727952103548 ) ) ;
#8812=CARTESIAN_POINT ( 'NONE',  ( -7.484045594489000308, -78.77392489796099539, 6.232877124219999843 ) ) ;
#8822=DIRECTION ( 'NONE',  ( 1.000000000000000000, 0.000000000000000000, 0.000000000000000000 ) ) ;
#8823=EDGE_CURVE ( 'NONE', #36505, #604, #34066, .T. ) ;
#8831=ORIENTED_EDGE ( 'NONE', *, *, #7675, .F. ) ;
#8835=CARTESIAN_POINT ( 'NONE',  ( -2.116314338179000387, -79.93777134585798194, -9.535298106756000536 ) ) ;
#8837=ORIENTED_EDGE ( 'NONE', *, *, #36891, .T. ) ;
#8851=CARTESIAN_POINT ( 'NONE',  ( 8.961394318992308428, -79.87002398672908043, 2.292941110240554359 ) ) ;
#8852=CARTESIAN_POINT ( 'NONE',  ( -10.33718531723983425, -80.42232376127893190, 3.786698599999175130 ) ) ;
#8860=CARTESIAN_POINT ( 'NONE',  ( -8.035240867088845107, -80.44999999999998863, -7.229432123523354292 ) ) ;
#8861=CARTESIAN_POINT ( 'NONE',  ( -7.655192530954000318, -79.92897315952798465, 7.967190206674000130 ) ) ;
#8881=CARTESIAN_POINT ( 'NONE',  ( 5.684557159767942736, -78.82291666666664298, 7.396918292183182864 ) ) ;
#8886=CARTESIAN_POINT ( 'NONE',  ( 10.97550047727999889, -78.24082415846498861, 0.05101033830554000531 ) ) ;
#8895=CARTESIAN_POINT ( 'NONE',  ( -7.000000000000000000, -80.99999999999998579, 0.000000000000000000 ) ) ;
#8898=APPLICATION_CONTEXT ( 'automotive_design' ) ;
#8899=CARTESIAN_POINT ( 'NONE',  ( -4.472180980751999435, -79.65088080519498703, 10.22208999787000039 ) ) ;
#8912=CYLINDRICAL_SURFACE ( 'NONE', #18348, 9.549999999999998934 ) ;
#8915=CARTESIAN_POINT ( 'NONE',  ( -7.847895170810467391, -79.70206533371160162, 5.399415251817809569 ) ) ;
#8923=AXIS2_PLACEMENT_3D ( 'NONE', #39660, #35805, #48258 ) ;
#8926=CARTESIAN_POINT ( 'NONE',  ( 1.441789035861242851, -77.46255880455122167, 9.136936837248049059 ) ) ;
#8927=CARTESIAN_POINT ( 'NONE',  ( -9.808193611224998776, -77.83189663113499535, 5.067887917229000116 ) ) ;
#8930=CARTESIAN_POINT ( 'NONE',  ( 2.867548251969000095, -78.03932568202999676, -9.270807752789000489 ) ) ;
#8934=FACE_OUTER_BOUND ( 'NONE', #40439, .T. ) ;
#8938=FACE_OUTER_BOUND ( 'NONE', #16399, .T. ) ;
#8941=B_SPLINE_CURVE_WITH_KNOTS ( 'NONE', 3,
 ( #44449, #58028, #58326, #17589 ),
 .UNSPECIFIED., .F., .F.,
 ( 4, 4 ),
 ( 0.000000000000000000, 1.000000000000000000 ),
 .UNSPECIFIED. ) ;
#8946=CARTESIAN_POINT ( 'NONE',  ( 5.000000000000000000, -75.19999999999998863, 0.000000000000000000 ) ) ;
#8971=DIRECTION ( 'NONE',  ( 1.000000000000000000, 0.000000000000000000, 0.000000000000000000 ) ) ;
#8976=VECTOR ( 'NONE', #54820, 1000.000000000000114 ) ;
#8977=CARTESIAN_POINT ( 'NONE',  ( 9.100722152916000951, -77.05266464630139467, -3.274758550341999808 ) ) ;
#8981=DIRECTION ( 'NONE',  ( 1.000000000000000000, 0.000000000000000000, 0.000000000000000000 ) ) ;
#8986=ADVANCED_FACE ( 'NONE', ( #30793 ), #12092, .F. ) ;
#9001=CARTESIAN_POINT ( 'NONE',  ( 6.574300740938999077, -77.52576138962918151, -8.869200617850999890 ) ) ;
#9004=ORIENTED_EDGE ( 'NONE', *, *, #33623, .F. ) ;
#9009=CARTESIAN_POINT ( 'NONE',  ( 8.898653440358000211, -78.42689348759698476, -3.871004561473999850 ) ) ;
#9012=PLANE ( 'NONE',  #28001 ) ;
#9017=CARTESIAN_POINT ( 'NONE',  ( -0.9948376905992144525, -76.94999999999998863, -9.499999997335510926 ) ) ;
#9024=CARTESIAN_POINT ( 'NONE',  ( -2.799999998984000094, -78.69999999898398357, 6.819591523630000610E-10 ) ) ;
#9043=CARTESIAN_POINT ( 'NONE',  ( -8.751877897654001259, -79.05082360769699790, -3.466385404677000182 ) ) ;
#9057=ADVANCED_FACE ( 'NONE', ( #15130 ), #5123, .F. ) ;
#9063=ORIENTED_EDGE ( 'NONE', *, *, #29153, .T. ) ;
#9066=CARTESIAN_POINT ( 'NONE',  ( 9.534323188421000239, -79.49169524832855416, -1.008198710029000189 ) ) ;
#9067=ORIENTED_EDGE ( 'NONE', *, *, #34007, .F. ) ;
#9068=VERTEX_POINT ( 'NONE', #19866 ) ;
#9076=CARTESIAN_POINT ( 'NONE',  ( 0.01626845465039130842, -78.72528669419055802, -9.249899724983746907 ) ) ;
#9079=CARTESIAN_POINT ( 'NONE',  ( 2.879226727952049814, -78.45416666666666572, 10.71369944335148183 ) ) ;
#9087=CARTESIAN_POINT ( 'NONE',  ( 10.99999999999999822, -79.85864668888551421, 1.195232468347080079 ) ) ;
#9098=CARTESIAN_POINT ( 'NONE',  ( 0.000000000000000000, -78.59999999921299718, 0.000000000000000000 ) ) ;
#9112=CARTESIAN_POINT ( 'NONE',  ( 5.539808784079867543, -78.93333333333333712, 9.611650271896852615 ) ) ;
#9113=CARTESIAN_POINT ( 'NONE',  ( 7.009066229391000213, -78.51811043579999705, -6.762594642477000484 ) ) ;
#9128=ORIENTED_EDGE ( 'NONE', *, *, #2704, .F. ) ;
#9129=CARTESIAN_POINT ( 'NONE',  ( 9.157990535730000659, -77.69412697158699643, -6.468229441713999606 ) ) ;
#9134=CARTESIAN_POINT ( 'NONE',  ( 9.767191983224998708, -79.58057210502099110, 0.05162932631433000269 ) ) ;
#9139=ORIENTED_EDGE ( 'NONE', *, *, #17110, .T. ) ;
#9142=ADVANCED_FACE ( 'NONE', ( #52038 ), #29001, .F. ) ;
#9148=CARTESIAN_POINT ( 'NONE',  ( -7.843978203195000276, -77.69990496493777243, 5.713380375430999969 ) ) ;
#9149=CARTESIAN_POINT ( 'NONE',  ( 8.100245516517501798, -79.89060762577963715, 4.466210091324835929 ) ) ;
#9152=CARTESIAN_POINT ( 'NONE',  ( -10.13316084080999957, -80.08481699542699062, 4.924182635666999985 ) ) ;
#9160=LINE ( 'NONE', #44290, #52474 ) ;
#9174=CARTESIAN_POINT ( 'NONE',  ( -9.504204889957000191, -77.13818535316588054, 0.5832244475350000235 ) ) ;
#9182=CARTESIAN_POINT ( 'NONE',  ( 10.85730540529999999, -79.19184598877099290, 1.607151491820999922 ) ) ;
#9187=VECTOR ( 'NONE', #43072, 1000.000000000000000 ) ;
#9190=CARTESIAN_POINT ( 'NONE',  ( -9.611650271896833075, -77.64166666666667993, -5.539808784079895077 ) ) ;
#9195=CARTESIAN_POINT ( 'NONE',  ( -5.018808260229000062, -78.39441589234299101, -9.843244246394000641 ) ) ;
#9199=CARTESIAN_POINT ( 'NONE',  ( -4.658475568430852753, -79.91666666666665719, 8.082524092276868188 ) ) ;
#9214=CARTESIAN_POINT ( 'NONE',  ( -3.517582505936258208, -78.19409754089322462, -8.554969473927931389 ) ) ;
#9221=CARTESIAN_POINT ( 'NONE',  ( -0.9113069885316975594, -77.48300007202549011, 9.208075695052512444 ) ) ;
#9222=CARTESIAN_POINT ( 'NONE',  ( -3.203604947276999848, -77.82858013947499387, 10.56508708803000118 ) ) ;
#9224=CARTESIAN_POINT ( 'NONE',  ( -9.282419925074000489, -77.35369851552198384, -2.829762163499999872 ) ) ;
#9230=CARTESIAN_POINT ( 'NONE',  ( 9.274475910318999539, -79.13469620609498634, -5.802750462065000114 ) ) ;
#9245=CARTESIAN_POINT ( 'NONE',  ( -10.76455872347999865, -80.53252629438799204, 3.409670607742999682 ) ) ;
#9250=ORIENTED_EDGE ( 'NONE', *, *, #8823, .F. ) ;
#9256=CARTESIAN_POINT ( 'NONE',  ( 9.028681611143001717, -78.01309479089799481, -5.970393136294000591 ) ) ;
#9262=CARTESIAN_POINT ( 'NONE',  ( 0.000000000000000000, -74.64999999999999147, 0.000000000000000000 ) ) ;
#9268=CARTESIAN_POINT ( 'NONE',  ( 2.309272084855999996, -77.03463947106759235, -9.392260232199999948 ) ) ;
#9271=CARTESIAN_POINT ( 'NONE',  ( -10.96673197750000206, -78.35320051065244229, -0.4413686857046000278 ) ) ;
#9276=CARTESIAN_POINT ( 'NONE',  ( -9.611650271896852615, -79.55833333333332291, 5.539808784079869319 ) ) ;
#9279=VERTEX_POINT ( 'NONE', #20906 ) ;
#9280=ORIENTED_EDGE ( 'NONE', *, *, #12812, .T. ) ;
#9286=CARTESIAN_POINT ( 'NONE',  ( -11.03649469273005046, -79.84071565590951991, 1.313607443778667783 ) ) ;
#9293=CARTESIAN_POINT ( 'NONE',  ( 1.277168492611395978, -77.21571277153906010, 10.79911615156215099 ) ) ;
#9295=ORIENTED_EDGE ( 'NONE', *, *, #27197, .F. ) ;
#9299=CARTESIAN_POINT ( 'NONE',  ( -8.771427373352999268, -77.74472158850198866, -4.151237309591000013 ) ) ;
#9318=CARTESIAN_POINT ( 'NONE',  ( 6.677308892935373663, -77.19999999999997442, -8.580962954970415169 ) ) ;
#9323=CARTESIAN_POINT ( 'NONE',  ( -1.439896632895311113, -79.31458333333334565, -11.00000000000000355 ) ) ;
#9334=CARTESIAN_POINT ( 'NONE',  ( -9.254388464354001087, -79.80752053325198858, 5.469807505829999528 ) ) ;
#9338=CARTESIAN_POINT ( 'NONE',  ( -6.987523971486999663, -79.07924743682598034, -6.307590925213999888 ) ) ;
#9356=ORIENTED_EDGE ( 'NONE', *, *, #41685, .F. ) ;
#9358=DIRECTION ( 'NONE',  ( 0.000000000000000000, 1.000000000000000000, 0.000000000000000000 ) ) ;
#9362=EDGE_LOOP ( 'NONE', ( #9573, #21755, #38834, #16750 ) ) ;
#9368=DIRECTION ( 'NONE',  ( 3.675129103447999014E-09, -0.9999999999999997780, -2.168720766502999921E-08 ) ) ;
#9372=CARTESIAN_POINT ( 'NONE',  ( 7.747891071769697824, -78.80404215024988446, -5.053095730781000050 ) ) ;
#9377=CARTESIAN_POINT ( 'NONE',  ( -4.658611238344869676, -77.68345333943109665, -8.082910578726778539 ) ) ;
#9393=CARTESIAN_POINT ( 'NONE',  ( -6.189430218157277785, -77.37374590179841505, 8.895180375493302094 ) ) ;
#9394=DIRECTION ( 'NONE',  ( -1.000000000000000000, 0.000000000000000000, 0.000000000000000000 ) ) ;
#9398=CARTESIAN_POINT ( 'NONE',  ( 0.000000000000000000, -74.99999999999998579, 0.000000000000000000 ) ) ;
#9406=CARTESIAN_POINT ( 'NONE',  ( 9.401690036064000111, -79.05816318924999564, -2.543243121375000193 ) ) ;
#9421=CARTESIAN_POINT ( 'NONE',  ( 10.12378227972000033, -78.20771289290198069, -4.818073696357999758 ) ) ;
#9424=ADVANCED_FACE ( 'NONE', ( #14884 ), #19617, .F. ) ;
#9425=ORIENTED_EDGE ( 'NONE', *, *, #5504, .F. ) ;
#9428=CARTESIAN_POINT ( 'NONE',  ( 9.202039358297998461, -80.28029040626950064, 2.360608321670000453 ) ) ;
#9438=CARTESIAN_POINT ( 'NONE',  ( -6.766389538252999714, -77.81360028145363117, -6.956053621355001049 ) ) ;
#9439=CARTESIAN_POINT ( 'NONE',  ( 8.220005723591295776, -79.88839068397346921, 4.241318902065857266 ) ) ;
#9454=CARTESIAN_POINT ( 'NONE',  ( 4.099999999699000419, -75.20000000030088927, -8.298664203784000017E-10 ) ) ;
#9467=CARTESIAN_POINT ( 'NONE',  ( -7.784718833714999064, -77.65684236001300178, 5.670217160303000270 ) ) ;
#9474=AXIS2_PLACEMENT_3D ( 'NONE', #10433, #19292, #37284 ) ;
#9475=CARTESIAN_POINT ( 'NONE',  ( 4.038786804788999873, -79.64544187509899587, -10.20549938643999965 ) ) ;
#9476=CARTESIAN_POINT ( 'NONE',  ( 10.61050599188999932, -77.92876026662598576, -2.901234667509999809 ) ) ;
#9477=CARTESIAN_POINT ( 'NONE',  ( -10.99961599049050953, -80.09872922184305821, 0.2432713142634969350 ) ) ;
#9481=ORIENTED_EDGE ( 'NONE', *, *, #26362, .T. ) ;
#9513=CARTESIAN_POINT ( 'NONE',  ( 2.816423976644823579, -77.45055722664174880, 8.810706099923065082 ) ) ;
#9514=CARTESIAN_POINT ( 'NONE',  ( 10.42639159904000046, -77.16057625750279669, -2.617796444239999687 ) ) ;
#9516=CARTESIAN_POINT ( 'NONE',  ( -5.159044788988000008, -77.41054617377999136, -8.219183903844999861 ) ) ;
#9521=CARTESIAN_POINT ( 'NONE',  ( 10.70874647057999951, -79.16278856042799816, -2.238429218213000116 ) ) ;
#9536=DIRECTION ( 'NONE',  ( 1.000000000000000000, 0.000000000000000000, 0.000000000000000000 ) ) ;
#9539=CARTESIAN_POINT ( 'NONE',  ( -8.334831687997999339, -78.04071980276798115, 4.375131454052000102 ) ) ;
#9549=CARTESIAN_POINT ( 'NONE',  ( 2.879226727952094222, -79.84583333333331723, -10.71369944335146940 ) ) ;
#9551=CARTESIAN_POINT ( 'NONE',  ( 0.000000000000000000, -75.19999999999998863, 0.000000000000000000 ) ) ;
#9569=CARTESIAN_POINT ( 'NONE',  ( 11.00000000000000000, -79.44999999999998863, 0.000000000000000000 ) ) ;
#9573=ORIENTED_EDGE ( 'NONE', *, *, #26432, .T. ) ;
#9579=CIRCLE ( 'NONE', #18976, 1.000000000000000000 ) ;
#9593=CARTESIAN_POINT ( 'NONE',  ( -0.1538805260928999830, -78.08580753804999119, 9.702939253146000809 ) ) ;
#9600=( GEOMETRIC_REPRESENTATION_CONTEXT ( 3 ) GLOBAL_UNCERTAINTY_ASSIGNED_CONTEXT ( ( #47299 ) ) GLOBAL_UNIT_ASSIGNED_CONTEXT ( ( #5710, #24311, #37293 ) ) REPRESENTATION_CONTEXT ( 'NONE', 'WORKASPACE' ) );
#9613=CARTESIAN_POINT ( 'NONE',  ( 11.03313550157999856, -78.37214908313399064, 0.1851758569619000039 ) ) ;
#9619=AXIS2_PLACEMENT_3D ( 'NONE', #33801, #23789, #41804 ) ;
#9620=EDGE_CURVE ( 'NONE', #40940, #45319, #44008, .T. ) ;
#9625=CARTESIAN_POINT ( 'NONE',  ( -2.975062338844999932, -77.84659905823998827, -10.76170074862000092 ) ) ;
#9628=CARTESIAN_POINT ( 'NONE',  ( 8.774584709929998283, -79.29716346014799910, 3.021992008916999595 ) ) ;
#9640=CARTESIAN_POINT ( 'NONE',  ( -10.78159125964999987, -79.35724697177198550, 1.856099740267000087 ) ) ;
#9651=ORIENTED_EDGE ( 'NONE', *, *, #787, .F. ) ;
#9662=CARTESIAN_POINT ( 'NONE',  ( -1.723907883222934201, -78.71014354949818426, -9.087954477670448838 ) ) ;
#9663=DIRECTION ( 'NONE',  ( 0.000000000000000000, 1.000000000000000000, 0.000000000000000000 ) ) ;
#9682=CARTESIAN_POINT ( 'NONE',  ( 7.714905556308770507, -79.55033101189913225, -5.543136766205470245 ) ) ;
#9684=CARTESIAN_POINT ( 'NONE',  ( 8.637786863126128978, -77.25138813405403937, 6.437705951042563157 ) ) ;
#9696=CARTESIAN_POINT ( 'NONE',  ( 8.931146968900000260, -78.54653426492899371, -3.885139576175999920 ) ) ;
#9709=CARTESIAN_POINT ( 'NONE',  ( 6.855510751285000204, -78.10715244345298913, -8.732042287340998854 ) ) ;
#9717=CARTESIAN_POINT ( 'NONE',  ( -9.358268528169000788, -79.41356642288599232, -2.797054701638000296 ) ) ;
#9723=ORIENTED_EDGE ( 'NONE', *, *, #35872, .T. ) ;
#9729=CARTESIAN_POINT ( 'NONE',  ( 7.912189497417754680, -79.89383890195257720, 4.794239927622985675 ) ) ;
#9742=CARTESIAN_POINT ( 'NONE',  ( -10.87436498444000144, -80.04903360897698406, 1.083693866698000052 ) ) ;
#9753=CARTESIAN_POINT ( 'NONE',  ( 4.977714881822485893, -76.94999999999998863, -8.125826846032065731 ) ) ;
#9756=CARTESIAN_POINT ( 'NONE',  ( 1.475792658273999969, -77.34418023959399591, -9.517102871385000995 ) ) ;
#9764=CARTESIAN_POINT ( 'NONE',  ( -4.399243655502999673, -79.89827306409299013, 10.05537673064999815 ) ) ;
#9765=CARTESIAN_POINT ( 'NONE',  ( -9.611650271896836628, -79.14166666666666572, -5.539808784079885307 ) ) ;
#9770=ORIENTED_EDGE ( 'NONE', *, *, #55900, .T. ) ;
#9777=CARTESIAN_POINT ( 'NONE',  ( -0.5228656313312000092, -78.92817062466399136, -11.03650783440000005 ) ) ;
#9783=CARTESIAN_POINT ( 'NONE',  ( 0.000000000000000000, -76.30000000005068728, -9.649999999948999374 ) ) ;
#9784=CARTESIAN_POINT ( 'NONE',  ( 9.632278712654541053, -79.23988867217208565, 5.261846222106294491 ) ) ;
#9805=ORIENTED_EDGE ( 'NONE', *, *, #27746, .T. ) ;
#9806=CARTESIAN_POINT ( 'NONE',  ( -0.02231494135697667525, -77.47534742525941454, 9.249882832515465836 ) ) ;
#9807=CARTESIAN_POINT ( 'NONE',  ( 2.604371601988999974, -77.57410247015199900, -10.72853197743999942 ) ) ;
#9808=CARTESIAN_POINT ( 'NONE',  ( 1.000000000000000000, -81.19999999999998863, 7.000000000000000000 ) ) ;
#9814=CARTESIAN_POINT ( 'NONE',  ( 10.82226978776999893, -79.19088091476099578, 1.601965348215999896 ) ) ;
#9819=ORIENTED_EDGE ( 'NONE', *, *, #10383, .F. ) ;
#9831=CARTESIAN_POINT ( 'NONE',  ( 8.191903123214999027, -77.87017682799398699, 4.637231687908999866 ) ) ;
#9838=DIRECTION ( 'NONE',  ( 0.7071067811865474617, 0.7071067811865474617, 2.341637280430153019E-09 ) ) ;
#9843=CARTESIAN_POINT ( 'NONE',  ( 0.9090372547675998893, -78.67794717677197980, 10.93790052299999971 ) ) ;
#9859=CARTESIAN_POINT ( 'NONE',  ( 0.000000000000000000, -74.64999999999999147, 0.000000000000000000 ) ) ;
#9877=CARTESIAN_POINT ( 'NONE',  ( 3.589839488473549611, -78.25675447763170212, -8.524986016596304950 ) ) ;
#9879=ORIENTED_EDGE ( 'NONE', *, *, #14479, .F. ) ;
#9885=CARTESIAN_POINT ( 'NONE',  ( -9.022250383429000209, -78.79985853368698656, -3.573472734901999903 ) ) ;
#9898=EDGE_CURVE ( 'NONE', #12885, #47367, #52677, .T. ) ;
#9902=CARTESIAN_POINT ( 'NONE',  ( 10.41647365791567381, -77.20000000000001705, -2.825691430128591808 ) ) ;
#9904=ORIENTED_EDGE ( 'NONE', *, *, #44488, .T. ) ;
#9906=DIRECTION ( 'NONE',  ( 0.000000000000000000, -1.000000000000000000, 2.129426118997999821E-13 ) ) ;
#9917=CARTESIAN_POINT ( 'NONE',  ( 1.937326043969999745, -77.16792237372438024, 10.88551626581000065 ) ) ;
#9920=CARTESIAN_POINT ( 'NONE',  ( 4.603815134758999505, -77.68647980950599674, -8.210729597153999748 ) ) ;
#9934=DIRECTION ( 'NONE',  ( 1.000000000000000000, 0.000000000000000000, 0.000000000000000000 ) ) ;
#9938=ORIENTED_EDGE ( 'NONE', *, *, #12812, .F. ) ;
#9946=ORIENTED_EDGE ( 'NONE', *, *, #30472, .F. ) ;
#9947=DIRECTION ( 'NONE',  ( 1.000000000000000000, 0.000000000000000000, 0.000000000000000000 ) ) ;
#9950=CARTESIAN_POINT ( 'NONE',  ( 8.898800776725989792, -78.56725350033094912, -3.871068654289783861 ) ) ;
#9959=CARTESIAN_POINT ( 'NONE',  ( -1.799037492230971980, -78.70949564512361007, -9.073313084848985355 ) ) ;
#9962=CARTESIAN_POINT ( 'NONE',  ( -5.636745332574527367, -80.18232361003532560, -9.445903029628405889 ) ) ;
#9974=CARTESIAN_POINT ( 'NONE',  ( 4.659053635387349956, -79.76712042365360844, -8.083800990292457911 ) ) ;
#9977=CARTESIAN_POINT ( 'NONE',  ( 0.000000000000000000, -78.49999999999998579, -2.600000000000000089 ) ) ;
#9980=CARTESIAN_POINT ( 'NONE',  ( -8.189132907799949734, -77.39413886308913959, 6.999642771075209602 ) ) ;
#9983=CARTESIAN_POINT ( 'NONE',  ( 10.85730540529999999, -79.11169407763458139, 1.607151491820999922 ) ) ;
#9989=CIRCLE ( 'NONE', #577, 2.600000000000000089 ) ;
#9991=CARTESIAN_POINT ( 'NONE',  ( 9.011045739978872149, -78.33204682128099705, -2.089134863993796998 ) ) ;
#9997=CARTESIAN_POINT ( 'NONE',  ( -0.2794722982914999987, -79.14806235426497949, 9.887242051013000577 ) ) ;
#10000=AXIS2_PLACEMENT_3D ( 'NONE', #12136, #7704, #54261 ) ;
#10005=ORIENTED_EDGE ( 'NONE', *, *, #42111, .T. ) ;
#10009=ORIENTED_EDGE ( 'NONE', *, *, #20888, .T. ) ;
#10011=CARTESIAN_POINT ( 'NONE',  ( 10.84815226135000010, -78.23216936534500121, -1.481085459616000133 ) ) ;
#10017=CARTESIAN_POINT ( 'NONE',  ( -2.116314338179000387, -79.99807427152899209, -9.535298106756000536 ) ) ;
#10026=CARTESIAN_POINT ( 'NONE',  ( 7.368185037057407349, -79.90209409743945912, 5.615580762807375947 ) ) ;
#10045=VECTOR ( 'NONE', #30272, 1000.000000000000000 ) ;
#10048=CARTESIAN_POINT ( 'NONE',  ( -2.891062785949999991, -76.92985585977308460, -9.145460139217000517 ) ) ;
#10049=DIRECTION ( 'NONE',  ( -1.000000000000000000, 0.000000000000000000, 0.000000000000000000 ) ) ;
#10053=CARTESIAN_POINT ( 'NONE',  ( -5.638451105654999296, -78.28216660084999035, -7.807757622656001040 ) ) ;
#10059=EDGE_CURVE ( 'NONE', #20388, #52990, #37538, .T. ) ;
#10062=CARTESIAN_POINT ( 'NONE',  ( -9.871730464199000465, -79.95445777275799060, 4.797141237513000256 ) ) ;
#10072=CARTESIAN_POINT ( 'NONE',  ( 10.70395128840999988, -78.11714908313399519, -0.4932637219220999958 ) ) ;
#10080=CARTESIAN_POINT ( 'NONE',  ( -9.009247259181927703, -79.97916666666664298, 2.421167930323307793 ) ) ;
#10082=CARTESIAN_POINT ( 'NONE',  ( 0.2613628514566687655, -79.57699692416433379, -10.97267097489929810 ) ) ;
#10099=ORIENTED_EDGE ( 'NONE', *, *, #30027, .F. ) ;
#10100=CARTESIAN_POINT ( 'NONE',  ( 9.249668415229836071, -77.35072839144281431, 0.08481753625212125336 ) ) ;
#10101=CARTESIAN_POINT ( 'NONE',  ( 9.507661145905998978, -77.57741896181198626, -5.611464101879999333 ) ) ;
#10108=CARTESIAN_POINT ( 'NONE',  ( -8.603527126503999867, -78.37620263911298935, 6.757746467621000619 ) ) ;
#10114=EDGE_CURVE ( 'NONE', #37542, #38384, #22491, .T. ) ;
#10121=CARTESIAN_POINT ( 'NONE',  ( 10.61050599188999932, -78.32876026662599145, -2.901234667509999809 ) ) ;
#10125=CARTESIAN_POINT ( 'NONE',  ( -8.883074525067000238, -78.55234872708999205, 3.114832498031999908 ) ) ;
#10133=AXIS2_PLACEMENT_3D ( 'NONE', #11816, #47846, #21240 ) ;
#10134=CARTESIAN_POINT ( 'NONE',  ( -4.999999999872000167, -80.49999999987198862, 4.857408280386999624E-10 ) ) ;
#10136=CARTESIAN_POINT ( 'NONE',  ( -6.920341278396000106, -79.38025603508899053, -8.518972542050999408 ) ) ;
#10156=DIRECTION ( 'NONE',  ( 0.000000000000000000, 0.000000000000000000, 1.000000000000000000 ) ) ;
#10158=DIRECTION ( 'NONE',  ( 0.000000000000000000, 1.000000000000000000, 0.000000000000000000 ) ) ;
#10170=CARTESIAN_POINT ( 'NONE',  ( 5.142492926713607027, -78.27207518130937558, -7.688654696769305019 ) ) ;
#10179=CARTESIAN_POINT ( 'NONE',  ( -9.282419925074000489, -77.23309266417999197, -2.829762163499999872 ) ) ;
#10184=DIRECTION ( 'NONE',  ( 0.000000000000000000, 1.000000000000000000, 0.000000000000000000 ) ) ;
#10201=CARTESIAN_POINT ( 'NONE',  ( 3.042616888044999968, -79.17893513191498300, 9.264577239222999694 ) ) ;
#10204=FACE_OUTER_BOUND ( 'NONE', #55768, .T. ) ;
#10206=CARTESIAN_POINT ( 'NONE',  ( 9.419185743363001961, -77.38288739614199585, -6.195553150604999892 ) ) ;
#10209=CARTESIAN_POINT ( 'NONE',  ( 1.222863591967999985, -77.88544661340898756, 9.333584474513999751 ) ) ;
#10238=CARTESIAN_POINT ( 'NONE',  ( 4.545340142815106788, -77.68611479733223746, 8.574013691167166940 ) ) ;
#10240=CARTESIAN_POINT ( 'NONE',  ( 0.000000000000000000, -74.64999999999999147, 0.000000000000000000 ) ) ;
#10246=CARTESIAN_POINT ( 'NONE',  ( 7.205376029061446808, -78.79611051935776800, -5.800537444989805280 ) ) ;
#10250=CARTESIAN_POINT ( 'NONE',  ( -7.396665944778026969, -80.16677562652540701, -8.142152547388292305 ) ) ;
#10271=CARTESIAN_POINT ( 'NONE',  ( 9.304500756975000897, -79.05550936896946723, -5.821536072646999571 ) ) ;
#10276=CARTESIAN_POINT ( 'NONE',  ( 8.780887922207014640, -78.32464479236936938, -2.908481940203349048 ) ) ;
#10281=CARTESIAN_POINT ( 'NONE',  ( 9.589208240076997569, -79.15046275916299123, 0.8944121949827000817 ) ) ;
#10298=CARTESIAN_POINT ( 'NONE',  ( 9.270530027976999321, -77.29059517626798481, 6.305874881421999589 ) ) ;
#10301=VERTEX_POINT ( 'NONE', #3211 ) ;
#10306=CARTESIAN_POINT ( 'NONE',  ( 8.985706068735000329, -79.60840237243299100, -3.828549499589000149 ) ) ;
#10323=AXIS2_PLACEMENT_3D ( 'NONE', #47579, #52556, #25389 ) ;
#10340=CARTESIAN_POINT ( 'NONE',  ( -9.070848764158998989, -77.18311187452979993, 2.805586010018000120 ) ) ;
#10348=CARTESIAN_POINT ( 'NONE',  ( -2.169167664939000151, -78.38128593012899614, 10.75912301088999889 ) ) ;
#10350=CARTESIAN_POINT ( 'NONE',  ( 8.664202219160999974, -79.35643979701998774, -4.294932555920000006 ) ) ;
#10354=CARTESIAN_POINT ( 'NONE',  ( -6.612779597103238594, -77.43740819862406966, 6.629663389723390310 ) ) ;
#10356=EDGE_CURVE ( 'NONE', #36426, #21041, #16785, .T. ) ;
#10365=CARTESIAN_POINT ( 'NONE',  ( 11.00000000000000000, -79.44999999999998863, 0.000000000000000000 ) ) ;
#10367=DIRECTION ( 'NONE',  ( 0.000000000000000000, -0.7071067811866525998, -0.7071067811864425456 ) ) ;
#10383=EDGE_CURVE ( 'NONE', #20614, #17190, #25351, .T. ) ;
#10387=CARTESIAN_POINT ( 'NONE',  ( 9.192586965176360536, -77.35899963357374531, 1.030861253847850101 ) ) ;
#10396=CARTESIAN_POINT ( 'NONE',  ( 6.696351723200000272, -79.10660385176299769, -8.651398149159000184 ) ) ;
#10402=CARTESIAN_POINT ( 'NONE',  ( -10.79944190718824082, -77.20000000000001705, 1.961979764079434752 ) ) ;
#10411=CARTESIAN_POINT ( 'NONE',  ( 6.053520011479999852, -77.89860065712299786, 7.208750930507999755 ) ) ;
#10421=CARTESIAN_POINT ( 'NONE',  ( 9.028681611143001717, -78.07339771656899075, -5.970393136294000591 ) ) ;
#10426=B_SPLINE_SURFACE_WITH_KNOTS ( 'NONE', 3, 3, ( 
 ( #51081, #46365, #32449, #42502, #6770, #55493, #5889, #56082, #15628, #1489, #32741, #50494, #10629, #33624, #6185, #51667, #24779, #10048, #28029 ),
 ( #23898, #46074, #5596, #23608, #19479, #28613, #41622, #33334, #15341, #19193, #51369, #42214, #6477, #37185, #24197, #19774, #37771, #55792, #46951 ),
 ( #38921, #39502, #52795, #25061, #35049, #7918, #3493, #3215, #7632, #57223, #12067, #12350, #30048, #20637, #2920, #21496, #26210, #3775, #12638 ),
 ( #56939, #38639, #39783, #56656, #52227, #51947, #48663, #16212, #48380, #34480, #30338, #53084, #21779, #25919, #8208, #57506, #7345, #21203, #15920 ) ),
 .UNSPECIFIED., .F., .F., .F.,
 ( 4, 4 ),
 ( 4, 1, 1, 1, 1, 1, 1, 1, 1, 1, 1, 1, 1, 1, 1, 1, 4 ),
 ( -0.1387574078320000237, 1.138757407831999968 ),
 ( -0.004592865874913999551, 0.01033394821856000075, 0.02526076231202999817, 0.04018757640548999838, 0.05511439049895999753, 0.07004120459242998975, 0.08496801868589999585, 0.09989483277937000194, 0.1148216468727999984, 0.1297484609662999944, 0.1446752750597999904, 0.1596020891533000141, 0.1745289032467000068, 0.1894557173402000028, 0.2043825314336999988, 0.2193093455270999914, 0.2342361596205999874 ),
 .UNSPECIFIED. ) ;
#10433=CARTESIAN_POINT ( 'NONE',  ( 0.000000000000000000, -76.39999999999999147, 0.000000000000000000 ) ) ;
#10439=EDGE_LOOP ( 'NONE', ( #2610, #51209, #51195, #42924, #5084, #33593, #57466, #46339 ) ) ;
#10442=FILL_AREA_STYLE_COLOUR ( '', #27482 ) ;
#10445=EDGE_LOOP ( 'NONE', ( #18448, #28048, #36579, #38073 ) ) ;
#10446=VERTEX_POINT ( 'NONE', #37400 ) ;
#10457=CARTESIAN_POINT ( 'NONE',  ( 6.818911827320396135, -78.29096144711863303, -6.251674546281022593 ) ) ;
#10462=CARTESIAN_POINT ( 'NONE',  ( -7.652281944047452100, -77.55252551045413156, 5.196868011323922509 ) ) ;
#10467=CARTESIAN_POINT ( 'NONE',  ( -1.182190922889000184, -78.88513002107399075, -9.631881180458998770 ) ) ;
#10483=CARTESIAN_POINT ( 'NONE',  ( 2.935661446561999899, -79.99999999999998579, -9.035036904803998681 ) ) ;
#10495=EDGE_CURVE ( 'NONE', #2535, #12885, #28541, .T. ) ;
#10499=CARTESIAN_POINT ( 'NONE',  ( 4.403823373056999557, -77.14888256794749566, 9.969607752326000494 ) ) ;
#10504=CARTESIAN_POINT ( 'NONE',  ( -1.900968108529000000, -77.62963215124798921, -9.219409434742001253 ) ) ;
#10509=FACE_BOUND ( 'NONE', #10993, .T. ) ;
#10518=ORIENTED_EDGE ( 'NONE', *, *, #7016, .F. ) ;
#10532=ORIENTED_EDGE ( 'NONE', *, *, #55315, .T. ) ;
#10533=CARTESIAN_POINT ( 'NONE',  ( -2.421342480286628795, -79.20438042701073300, -9.010110489339714590 ) ) ;
#10534=CARTESIAN_POINT ( 'NONE',  ( 9.259200219731782866, -78.62410115858894244, 2.905346636976683605 ) ) ;
#10538=CARTESIAN_POINT ( 'NONE',  ( -3.536681740116999872, -78.15468623100123580, 9.036735673663999435 ) ) ;
#10542=CARTESIAN_POINT ( 'NONE',  ( -7.608820801282668356, -78.64829813045270157, -5.263042126654066344 ) ) ;
#10577=CARTESIAN_POINT ( 'NONE',  ( -7.400482488103000023, -78.83780063874398536, 6.163283938603000500 ) ) ;
#10587=CARTESIAN_POINT ( 'NONE',  ( -9.247932426686000795, -77.50168256874098915, -0.1955654147372000162 ) ) ;
#10592=CARTESIAN_POINT ( 'NONE',  ( 8.081843650394000989, -77.30829253183799210, -8.086130236420000728 ) ) ;
#10599=CARTESIAN_POINT ( 'NONE',  ( 6.728605944993000243, -79.57592971417498973, -7.080011783993000130 ) ) ;
#10629=CARTESIAN_POINT ( 'NONE',  ( 9.133953537529999167, -77.05169957229118438, -3.286716366334999861 ) ) ;
#10636=CARTESIAN_POINT ( 'NONE',  ( 5.883202309618000392, -77.88423299304498926, -7.625033806424000637 ) ) ;
#10638=CARTESIAN_POINT ( 'NONE',  ( -1.229229940090210249, -77.06588541667790082, 9.384114583052001635 ) ) ;
#10647=CARTESIAN_POINT ( 'NONE',  ( 9.503328962285682024, -79.49493491590959593, -0.6046619501317949119 ) ) ;
#10649=CARTESIAN_POINT ( 'NONE',  ( 3.915498778898000687, -79.33642597743899216, 10.25343288338999947 ) ) ;
#10651=CARTESIAN_POINT ( 'NONE',  ( -10.44613170738330332, -80.07483812962188097, 3.446999337742282510 ) ) ;
#10652=CARTESIAN_POINT ( 'NONE',  ( 9.248423471988997946, -79.91665467088898822, 2.825168219357999888 ) ) ;
#10670=CARTESIAN_POINT ( 'NONE',  ( 6.718136267461014555, -79.12751925484205628, -8.679542842522213419 ) ) ;
#10688=CARTESIAN_POINT ( 'NONE',  ( 7.479723288845285367, -77.40016007753332872, 5.441954638049121940 ) ) ;
#10689=CARTESIAN_POINT ( 'NONE',  ( -9.177034484502000211, -77.44354714383098326, 6.137278520473000043 ) ) ;
#10691=CARTESIAN_POINT ( 'NONE',  ( 9.131029190779001325, -77.61296824509499004, -3.285576857342999979 ) ) ;
#10698=CARTESIAN_POINT ( 'NONE',  ( 8.926269970182000080, -78.69290956889000199, -6.511497375149000177 ) ) ;
#10699=ADVANCED_FACE ( 'NONE', ( #35277 ), #30853, .F. ) ;
#10704=CARTESIAN_POINT ( 'NONE',  ( -10.22338514145507737, -77.19999999999998863, 3.927200133048044606 ) ) ;
#10712=CARTESIAN_POINT ( 'NONE',  ( 2.781615572646999990, -77.72805768234898949, -8.992986673707997980 ) ) ;
#10723=CARTESIAN_POINT ( 'NONE',  ( -2.928603948516999900, -78.70603953110398265, 10.57767911662999971 ) ) ;
#10741=EDGE_LOOP ( 'NONE', ( #27598, #8469, #7602, #23723, #32272, #46769, #8690, #3327, #42343 ) ) ;
#10745=ORIENTED_EDGE ( 'NONE', *, *, #50924, .T. ) ;
#10758=CARTESIAN_POINT ( 'NONE',  ( 5.918406792461694543, -78.28036926306923249, -7.108720655904040342 ) ) ;
#10760=ORIENTED_EDGE ( 'NONE', *, *, #24981, .F. ) ;
#10762=CARTESIAN_POINT ( 'NONE',  ( -9.137085346172289846, -77.58769485083752215, 1.440358904308211674 ) ) ;
#10766=CARTESIAN_POINT ( 'NONE',  ( -9.346518596363001308, -77.74817685591499128, 2.610229778083999808 ) ) ;
#10769=CARTESIAN_POINT ( 'NONE',  ( 0.000000000000000000, -80.74999999986198418, 0.000000000000000000 ) ) ;
#10771=VECTOR ( 'NONE', #25446, 1000.000000000000000 ) ;
#10781=CARTESIAN_POINT ( 'NONE',  ( -4.657764537801160287, -79.51694645399435046, 8.081867300299901302 ) ) ;
#10786=EDGE_CURVE ( 'NONE', #52834, #36325, #8941, .T. ) ;
#10790=CARTESIAN_POINT ( 'NONE',  ( 5.228979477480000249, -79.62813585431899810, -7.971711000620000043 ) ) ;
#10792=CARTESIAN_POINT ( 'NONE',  ( -9.703099203832849184, -79.34568276157449418, 0.5050087370209813686 ) ) ;
#10796=CARTESIAN_POINT ( 'NONE',  ( 10.36233872082999774, -77.89696215211898789, -4.441556149583999691 ) ) ;
#10797=EDGE_CURVE ( 'NONE', #18403, #30305, #27220, .T. ) ;
#10810=VERTEX_POINT ( 'NONE', #46230 ) ;
#10821=EDGE_LOOP ( 'NONE', ( #5208, #35022, #10518, #28958 ) ) ;
#10822=ORIENTED_EDGE ( 'NONE', *, *, #5924, .T. ) ;
#10837=CARTESIAN_POINT ( 'NONE',  ( 9.499178638196321245, -79.00092112126561972, 0.1004274591880019996 ) ) ;
#10839=CARTESIAN_POINT ( 'NONE',  ( -0.09237677837556851346, -79.72557714387301075, 9.715793344066241843 ) ) ;
#10842=CARTESIAN_POINT ( 'NONE',  ( -6.203490556899441621, -78.66660757515437297, -6.861839749120386855 ) ) ;
#10847=CARTESIAN_POINT ( 'NONE',  ( -5.338532579233360664, -80.18476939357704225, -9.618388971371432561 ) ) ;
#10856=CARTESIAN_POINT ( 'NONE',  ( 3.931521788677165397, -79.99999999999997158, 8.490588278901316954 ) ) ;
#10866=CARTESIAN_POINT ( 'NONE',  ( 2.464155593302254754, -77.80709632922713581, 10.48634603565272627 ) ) ;
#10868=CARTESIAN_POINT ( 'NONE',  ( 7.318097147681000614, -79.53307939262458603, -8.179820946710000484 ) ) ;
#10873=CARTESIAN_POINT ( 'NONE',  ( 8.720468637437409853, -78.32301164407923011, -3.084721045281239249 ) ) ;
#10877=CARTESIAN_POINT ( 'NONE',  ( -5.638451105654999296, -78.46829086006698617, -7.807757622656001040 ) ) ;
#10886=CARTESIAN_POINT ( 'NONE',  ( -7.069392057028999865, -79.23718652232298609, 8.491265488204000178 ) ) ;
#10887=CARTESIAN_POINT ( 'NONE',  ( -8.975709286823001065, -80.12499131680598907, 7.273687588511000612 ) ) ;
#10890=CARTESIAN_POINT ( 'NONE',  ( 3.641219478425000045, -77.27160782317299947, -10.83718297704999856 ) ) ;
#10895=EDGE_LOOP ( 'NONE', ( #20438, #1094, #5789, #22578, #17697 ) ) ;
#10898=CARTESIAN_POINT ( 'NONE',  ( -5.809791519574999619, -79.55585413501300707, 7.851562197947999699 ) ) ;
#10899=VERTEX_POINT ( 'NONE', #43522 ) ;
#10906=CARTESIAN_POINT ( 'NONE',  ( 9.549999999999998934, -80.99999999999998579, 0.000000000000000000 ) ) ;
#10908=CARTESIAN_POINT ( 'NONE',  ( -4.099999999699000419, -75.20000000030088927, 8.298667500436000154E-10 ) ) ;
#10910=CARTESIAN_POINT ( 'NONE',  ( 2.968094753861000079, -77.12165489554539022, 9.474519209979000323 ) ) ;
#10931=CARTESIAN_POINT ( 'NONE',  ( -2.191084135724000070, -77.66387044253798422, 9.489933931099999498 ) ) ;
#10933=CARTESIAN_POINT ( 'NONE',  ( -11.00000000000000000, -77.69999999999998863, 0.000000000000000000 ) ) ;
#10943=CARTESIAN_POINT ( 'NONE',  ( -10.91764451743335762, -80.09049157782284567, 1.351593570394689081 ) ) ;
#10944=CARTESIAN_POINT ( 'NONE',  ( 9.669905736194998269, -79.39378745527798742, 0.08814083877134999689 ) ) ;
#10960=CARTESIAN_POINT ( 'NONE',  ( 10.80348683896752959, -79.46729337777097157, 2.390241153868424284 ) ) ;
#10982=CARTESIAN_POINT ( 'NONE',  ( 8.238405875913969112, -77.38767930335906442, 4.205914151111458388 ) ) ;
#10989=CARTESIAN_POINT ( 'NONE',  ( -9.878709405926999310, -79.03001782088199434, -4.948635581693999974 ) ) ;
#10993=EDGE_LOOP ( 'NONE', ( #12308, #23727, #28422 ) ) ;
#10994=CARTESIAN_POINT ( 'NONE',  ( -10.16722439191025629, -77.19999999999998863, 4.064972966511320784 ) ) ;
#11002=CARTESIAN_POINT ( 'NONE',  ( 9.085337660295000006, -78.41725766396999120, 2.850792140868000146 ) ) ;
#11015=CARTESIAN_POINT ( 'NONE',  ( 10.94409238582999855, -78.56557775944099831, 0.8311789410725000105 ) ) ;
#11029=CARTESIAN_POINT ( 'NONE',  ( -7.707335466132000157, -78.74423443443198778, -8.217415310065000256 ) ) ;
#11036=EDGE_CURVE ( 'NONE', #50169, #40498, #48255, .T. ) ;
#11042=CARTESIAN_POINT ( 'NONE',  ( 0.000000000000000000, -76.30000000005068728, 0.000000000000000000 ) ) ;
#11047=CARTESIAN_POINT ( 'NONE',  ( 8.974834626914359959, -79.97252914747060970, -3.225705101019638033 ) ) ;
#11054=CARTESIAN_POINT ( 'NONE',  ( 3.541417221457102915, -78.25630717469576325, -8.545189235367685043 ) ) ;
#11058=CARTESIAN_POINT ( 'NONE',  ( -8.823116529173212541, -77.57575035185114132, 2.777645208995981996 ) ) ;
#11059=FACE_OUTER_BOUND ( 'NONE', #52762, .T. ) ;
#11062=CARTESIAN_POINT ( 'NONE',  ( 6.240531904507999883, -78.08926280546299381, 7.431451467605000083 ) ) ;
#11065=VECTOR ( 'NONE', #32378, 1000.000000000000000 ) ;
#11087=CARTESIAN_POINT ( 'NONE',  ( -5.134431902050000218, -79.97337732914698449, -8.161852231781001166 ) ) ;
#11093=CARTESIAN_POINT ( 'NONE',  ( 2.932810412914000242, -77.51739520116099413, -10.54767017414000208 ) ) ;
#11097=CARTESIAN_POINT ( 'NONE',  ( 7.993200843029001135, -78.22653256295699009, -4.971914600080000746 ) ) ;
#11114=ORIENTED_EDGE ( 'NONE', *, *, #53159, .F. ) ;
#11121=ORIENTED_EDGE ( 'NONE', *, *, #51244, .F. ) ;
#11131=CARTESIAN_POINT ( 'NONE',  ( 8.444976262095000408, -78.04099091448563286, 4.780490068936999570 ) ) ;
#11138=CARTESIAN_POINT ( 'NONE',  ( -2.993561518543238709, -78.69892983886539639, -8.753304730231880271 ) ) ;
#11142=CARTESIAN_POINT ( 'NONE',  ( -10.89273321435514497, -80.11128739981552371, -1.531847966823179918 ) ) ;
#11157=CARTESIAN_POINT ( 'NONE',  ( -2.444356268457450909, -77.55728255341558963, -10.55741984921857046 ) ) ;
#11159=CONICAL_SURFACE ( 'NONE', #40373, 10.59999999997999787, 0.7853981633972997312 ) ;
#11160=CARTESIAN_POINT ( 'NONE',  ( 6.612939829087000732, -79.67354116428806776, 8.759739992124000452 ) ) ;
#11165=CARTESIAN_POINT ( 'NONE',  ( 9.152874836537630898, -78.33854092996706697, -1.339099148577004739 ) ) ;
#11169=CARTESIAN_POINT ( 'NONE',  ( 8.475813183550998886, -78.12017682799398699, 4.797946079729999092 ) ) ;
#11182=CARTESIAN_POINT ( 'NONE',  ( 11.32642973867000080, -77.38166194916898633, 1.553704360265000028 ) ) ;
#11189=CARTESIAN_POINT ( 'NONE',  ( -7.479908383216000267, -79.56589192459449578, -6.281056869080000382 ) ) ;
#11198=CARTESIAN_POINT ( 'NONE',  ( 0.000000000000000000, -80.99999999999998579, 7.000000000000000000 ) ) ;
#11200=CARTESIAN_POINT ( 'NONE',  ( 7.135985293347999914, -76.86160783604827884, -6.061232200253999558 ) ) ;
#11201=EDGE_CURVE ( 'NONE', #17327, #5962, #44231, .T. ) ;
#11203=CARTESIAN_POINT ( 'NONE',  ( -2.879226727952072018, -79.70416666666665151, -10.71369944335147295 ) ) ;
#11205=CARTESIAN_POINT ( 'NONE',  ( 6.582919013437252609, -77.16874999997368434, -6.583307234616106562 ) ) ;
#11219=CARTESIAN_POINT ( 'NONE',  ( -8.102939992022999860, -78.31761851250499262, -5.403892966383000207 ) ) ;
#11224=DIRECTION ( 'NONE',  ( 0.000000000000000000, -1.000000000000000000, 0.000000000000000000 ) ) ;
#11230=CARTESIAN_POINT ( 'NONE',  ( -9.888820909766963041, -80.06422814540057686, 4.845029618406575089 ) ) ;
#11231=CARTESIAN_POINT ( 'NONE',  ( 7.549855238205000596, -78.88173981539898705, 5.864427966874999676 ) ) ;
#11246=DIRECTION ( 'NONE',  ( 1.000000000000000000, 0.000000000000000000, 0.000000000000000000 ) ) ;
#11248=DIRECTION ( 'NONE',  ( 0.000000000000000000, -1.000000000000000000, 0.000000000000000000 ) ) ;
#11267=CARTESIAN_POINT ( 'NONE',  ( 7.356220924712871145, -77.29817559292861517, -5.612009723571459219 ) ) ;
#11268=CARTESIAN_POINT ( 'NONE',  ( 10.07768261906999996, -78.20698015179898732, -4.508174471003999706 ) ) ;
#11278=CARTESIAN_POINT ( 'NONE',  ( -9.501885680564001291, -79.53568019887099183, -5.638445012646999821 ) ) ;
#11290=CARTESIAN_POINT ( 'NONE',  ( 8.731705537153999330, -78.36041000571199788, -3.798380529179000042 ) ) ;
#11293=CARTESIAN_POINT ( 'NONE',  ( 0.000000000000000000, -81.90000000002299885, 0.000000000000000000 ) ) ;
#11301=CARTESIAN_POINT ( 'NONE',  ( 10.94409238582999855, -78.62588068511199424, 0.8311789410725000105 ) ) ;
#11306=CARTESIAN_POINT ( 'NONE',  ( -10.69999999999999929, -77.19999999999998863, 0.000000000000000000 ) ) ;
#11311=EDGE_CURVE ( 'NONE', #48925, #37657, #42363, .T. ) ;
#11312=CARTESIAN_POINT ( 'NONE',  ( -5.068180973607000261, -78.33054015155998684, -9.940077528656999561 ) ) ;
#11328=EDGE_CURVE ( 'NONE', #17190, #43667, #35098, .T. ) ;
#11330=CARTESIAN_POINT ( 'NONE',  ( 2.074043784921811628, -79.89245142283287748, -9.331470595881391716 ) ) ;
#11337=CARTESIAN_POINT ( 'NONE',  ( -1.799561319299137985, -78.20949348124068479, -9.073216031666641257 ) ) ;
#11340=EDGE_LOOP ( 'NONE', ( #43171, #39987 ) ) ;
#11344=DIRECTION ( 'NONE',  ( 0.000000000000000000, 0.000000000000000000, -1.000000000000000000 ) ) ;
#11347=CARTESIAN_POINT ( 'NONE',  ( 8.240135455977000589, -78.03587041461697993, -5.125512367919999868 ) ) ;
#11351=DIRECTION ( 'NONE',  ( 0.000000000000000000, -1.000000000000000000, 0.000000000000000000 ) ) ;
#11363=AXIS2_PLACEMENT_3D ( 'NONE', #4551, #32554, #50602 ) ;
#11366=CARTESIAN_POINT ( 'NONE',  ( -8.752258451002999706, -79.98164082875798897, -6.780921793939000075 ) ) ;
#11369=VERTEX_POINT ( 'NONE', #56981 ) ;
#11373=CARTESIAN_POINT ( 'NONE',  ( 3.815187358399000139, -80.11518015861798858, -8.581477306024998697 ) ) ;
#11379=EDGE_CURVE ( 'NONE', #11369, #3961, #39481, .T. ) ;
#11382=CARTESIAN_POINT ( 'NONE',  ( 10.16239288306999988, -78.02471363368498203, -4.355854389664999715 ) ) ;
#11388=CARTESIAN_POINT ( 'NONE',  ( 1.210822168571061175, -78.36458333333334281, 9.250000000000001776 ) ) ;
#11394=CARTESIAN_POINT ( 'NONE',  ( 9.549999999999998934, -76.39999999999999147, 0.000000000000000000 ) ) ;
#11398=ORIENTED_EDGE ( 'NONE', *, *, #57125, .T. ) ;
#11417=CARTESIAN_POINT ( 'NONE',  ( 9.611650271896829523, -78.49166666666667425, 5.539808784079915505 ) ) ;
#11419=CARTESIAN_POINT ( 'NONE',  ( -4.412537506371384310, -78.68548379871316456, -8.131199301624301157 ) ) ;
#11423=CARTESIAN_POINT ( 'NONE',  ( -10.28968504916697313, -80.12913738177938683, -3.888065173257339247 ) ) ;
#11428=EDGE_CURVE ( 'NONE', #45010, #29062, #52873, .T. ) ;
#11440=AXIS2_PLACEMENT_3D ( 'NONE', #22698, #21602, #23568 ) ;
#11441=CARTESIAN_POINT ( 'NONE',  ( -8.316360841097289125, -78.00592770181216906, -6.948075690853510622 ) ) ;
#11445=VERTEX_POINT ( 'NONE', #23803 ) ;
#11452=CARTESIAN_POINT ( 'NONE',  ( 9.062046460520999602, -77.61557598619799592, -3.260755114102000363 ) ) ;
#11458=DIRECTION ( 'NONE',  ( 1.000000000000000000, 0.000000000000000000, 0.000000000000000000 ) ) ;
#11460=EDGE_CURVE ( 'NONE', #44860, #37493, #8125, .T. ) ;
#11464=CARTESIAN_POINT ( 'NONE',  ( 2.567527713034000403, -78.45060060100799149, -10.74642708485000142 ) ) ;
#11466=CARTESIAN_POINT ( 'NONE',  ( 5.729309059712077712, -77.67757408254945517, -7.360974123654262513 ) ) ;
#11467=CARTESIAN_POINT ( 'NONE',  ( -9.709765936195999814, -79.63777772118899634, 5.586663845304999931 ) ) ;
#11471=CARTESIAN_POINT ( 'NONE',  ( -10.46158978484000102, -78.08816509035798958, -4.329824488994000298 ) ) ;
#11474=ORIENTED_EDGE ( 'NONE', *, *, #22117, .T. ) ;
#11477=CARTESIAN_POINT ( 'NONE',  ( -9.387315177295000979, -80.22774216884852194, 2.697965643110000311 ) ) ;
#11489=CARTESIAN_POINT ( 'NONE',  ( 2.914566591598000134, -77.01848277179368552, 9.303650809983000869 ) ) ;
#11494=CARTESIAN_POINT ( 'NONE',  ( 9.249999999999998224, -77.76041666666667140, 1.210822168571084934 ) ) ;
#11502=ORIENTED_EDGE ( 'NONE', *, *, #27994, .F. ) ;
#11510=FACE_OUTER_BOUND ( 'NONE', #49584, .T. ) ;
#11512=CARTESIAN_POINT ( 'NONE',  ( 0.000000000000000000, -75.09999999979599750, 0.000000000000000000 ) ) ;
#11516=CARTESIAN_POINT ( 'NONE',  ( -7.052869246477441401, -79.30872110581411505, -6.415029687693263760 ) ) ;
#11520=CARTESIAN_POINT ( 'NONE',  ( -10.19950126981313687, -80.06978458045568914, 4.126879458600376971 ) ) ;
#11521=CARTESIAN_POINT ( 'NONE',  ( -5.286327514246000447, -80.06604530392098695, 7.677899541690999641 ) ) ;
#11522=DIRECTION ( 'NONE',  ( 1.000000000000000000, 0.000000000000000000, 0.000000000000000000 ) ) ;
#11523=CARTESIAN_POINT ( 'NONE',  ( -1.439896632895311335, -78.71458333333333712, -11.00000000000000178 ) ) ;
#11530=ADVANCED_FACE ( 'NONE', ( #21121 ), #17870, .F. ) ;
#11546=CARTESIAN_POINT ( 'NONE',  ( 9.253998064331378615, -79.07669581907259726, -2.773690070707886424 ) ) ;
#11556=CARTESIAN_POINT ( 'NONE',  ( 5.442070907333274477, -77.27518984243994282, -7.479617580235857766 ) ) ;
#11566=CARTESIAN_POINT ( 'NONE',  ( 9.295311691678000088, -79.78851138786500030, 5.972861453165999812 ) ) ;
#11571=CARTESIAN_POINT ( 'NONE',  ( -2.508516875516433320, -77.19999999999998863, 10.53783702169892678 ) ) ;
#11580=CARTESIAN_POINT ( 'NONE',  ( 0.8456326333846000409, -78.27513851832499370, -9.484475825334998333 ) ) ;
#11588=CARTESIAN_POINT ( 'NONE',  ( -7.396918292183192634, -78.94791666666665719, 5.684557159767932077 ) ) ;
#11594=CARTESIAN_POINT ( 'NONE',  ( 0.9090372547675998893, -78.73825010244298994, 10.93790052299999971 ) ) ;
#11598=CYLINDRICAL_SURFACE ( 'NONE', #35891, 9.250000000000000000 ) ;
#11602=CARTESIAN_POINT ( 'NONE',  ( 4.658475568430802127, -78.16666666666665719, -8.082524092276894834 ) ) ;
#11604=CARTESIAN_POINT ( 'NONE',  ( -6.574673376928999780, -78.60377266276799446, 9.148912741538998361 ) ) ;
#11625=B_SPLINE_SURFACE_WITH_KNOTS ( 'NONE', 3, 3, ( 
 ( #30231, #26094, #48274, #29935, #56829, #57402, #7231, #43839, #47988, #21097, #25235, #21381, #16960, #34942, #16676, #57110, #3386, #25521, #20525 ),
 ( #30521, #16099, #11957, #43255, #48552, #8098, #34657, #17238, #47412, #52685, #35225, #53256, #7524, #29364, #34079, #24946, #2523, #20805, #38523 ),
 ( #52115, #11675, #29650, #47701, #38812, #16385, #39963, #21951, #18423, #731, #49725, #8675, #8977, #444, #18711, #36705, #41140, #18130, #4843 ),
 ( #12805, #49125, #23132, #22839, #50015, #17836, #31088, #40852, #36413, #22249, #13385, #26377, #30804, #44396, #48837, #9268, #36125, #3948, #54441 ) ),
 .UNSPECIFIED., .F., .F., .F.,
 ( 4, 4 ),
 ( 4, 1, 1, 1, 1, 1, 1, 1, 1, 1, 1, 1, 1, 1, 1, 1, 4 ),
 ( -0.4045438850609999748, 1.404543885061000141 ),
 ( -0.004592865874913999551, 0.01033394821856000075, 0.02526076231202999817, 0.04018757640548999838, 0.05511439049895999753, 0.07004120459242998975, 0.08496801868589999585, 0.09989483277937000194, 0.1148216468727999984, 0.1297484609662999944, 0.1446752750597999904, 0.1596020891533000141, 0.1745289032467000068, 0.1894557173402000028, 0.2043825314336999988, 0.2193093455270999914, 0.2342361596205999874 ),
 .UNSPECIFIED. ) ;
#11628=CARTESIAN_POINT ( 'NONE',  ( -2.632720150768073974, -78.20209331882408321, -8.868811374433354544 ) ) ;
#11632=CARTESIAN_POINT ( 'NONE',  ( -4.216522652542374239, -77.51279216956007190, 8.232977916204301749 ) ) ;
#11636=CARTESIAN_POINT ( 'NONE',  ( -7.843978203195000276, -77.78005595245699055, 5.713380375430999969 ) ) ;
#11650=CARTESIAN_POINT ( 'NONE',  ( 2.398181734629726503, -79.45434264457517770, 8.953979686625713086 ) ) ;
#11651=CARTESIAN_POINT ( 'NONE',  ( 0.7222841580580000587, -80.29899131680598146, 11.04814689212999923 ) ) ;
#11661=CARTESIAN_POINT ( 'NONE',  ( 3.338062356706000156, -79.80347180386698369, 8.930159145143999666 ) ) ;
#11669=CARTESIAN_POINT ( 'NONE',  ( 6.514771768986000744, -77.48207916904298997, -8.933413800474999888 ) ) ;
#11675=CARTESIAN_POINT ( 'NONE',  ( -9.555818165766000405, -77.33116456062899147, -0.1257991660602000017 ) ) ;
#11677=CARTESIAN_POINT ( 'NONE',  ( -1.439896632895359962, -77.48541666666666572, 10.99999999999999645 ) ) ;
#11697=CARTESIAN_POINT ( 'NONE',  ( -9.009247259181922374, -79.52083333333332860, -2.421167930323344653 ) ) ;
#11705=CARTESIAN_POINT ( 'NONE',  ( -9.497876546326999403, -77.25168256874098915, -0.2008509664869000122 ) ) ;
#11709=CARTESIAN_POINT ( 'NONE',  ( -2.251478210889264364, -76.95593248568935962, -9.257098554661395085 ) ) ;
#11711=CARTESIAN_POINT ( 'NONE',  ( -3.481545117580455262, -78.69439501636868783, -8.569750538382592708 ) ) ;
#11713=CARTESIAN_POINT ( 'NONE',  ( -10.93151875640478643, -80.10922970060033776, -1.237410007773367404 ) ) ;
#11725=FACE_OUTER_BOUND ( 'NONE', #32792, .T. ) ;
#11737=CARTESIAN_POINT ( 'NONE',  ( 2.845884614340000063, -78.04193342313199366, -9.200769029100998253 ) ) ;
#11746=CARTESIAN_POINT ( 'NONE',  ( 10.24785796630000156, -78.14927573546698625, 3.830033060943999867 ) ) ;
#11748=CARTESIAN_POINT ( 'NONE',  ( -4.043962765326000408, -80.21098163303398110, 10.58371677765999941 ) ) ;
#11756=CARTESIAN_POINT ( 'NONE',  ( -0.5483576180056000116, -79.63083724111049833, -9.751923335751000010 ) ) ;
#11775=CARTESIAN_POINT ( 'NONE',  ( -9.009247259181927703, -77.97916666666667140, 2.421167930323307793 ) ) ;
#11785=CARTESIAN_POINT ( 'NONE',  ( 9.250000000000000000, -79.24999999999998579, 0.000000000000000000 ) ) ;
#11789=CARTESIAN_POINT ( 'NONE',  ( -5.702118101738999911, -78.34604234163299452, -7.895919506952999711 ) ) ;
#11798=CARTESIAN_POINT ( 'NONE',  ( 2.308268922230239273, -79.39449714348630494, -9.238196189940964587 ) ) ;
#11799=CARTESIAN_POINT ( 'NONE',  ( -4.419147127517656592, -79.99999999999998579, -8.303618670951507852 ) ) ;
#11802=CARTESIAN_POINT ( 'NONE',  ( -10.49130490104844604, -80.07586413098869116, 3.306199282034132825 ) ) ;
#11803=CARTESIAN_POINT ( 'NONE',  ( 9.065614955752000270, -78.93479598044999079, -2.589622044563999914 ) ) ;
#11805=CARTESIAN_POINT ( 'NONE',  ( 9.250000000000000000, -79.24999999999998579, 0.000000000000000000 ) ) ;
#11813=VERTEX_POINT ( 'NONE', #37023 ) ;
#11816=CARTESIAN_POINT ( 'NONE',  ( 0.000000000000000000, -74.64999999999999147, 0.000000000000000000 ) ) ;
#11818=CARTESIAN_POINT ( 'NONE',  ( 10.71573898357587851, -79.71745869582807131, 2.375027775440368139 ) ) ;
#11819=CYLINDRICAL_SURFACE ( 'NONE', #42243, 11.00000000000000000 ) ;
#11826=CARTESIAN_POINT ( 'NONE',  ( -7.456940411035866134, -78.79464413336293660, 6.210303333646408852 ) ) ;
#11839=CARTESIAN_POINT ( 'NONE',  ( -3.642272407944000090, -79.71961638910200065, -10.66127506782999923 ) ) ;
#11840=CARTESIAN_POINT ( 'NONE',  ( 4.552121687394530269, -77.26596116455657182, -8.053328680974594533 ) ) ;
#11843=B_SPLINE_CURVE_WITH_KNOTS ( 'NONE', 3,
 ( #17160, #52894, #44036, #30147, #44316, #21872, #34291, #7729, #43754, #47912, #35436, #16883, #53465, #48197, #25443, #44613, #21016, #22166 ),
 .UNSPECIFIED., .F., .F.,
 ( 4, 2, 2, 2, 2, 2, 2, 2, 4 ),
 ( 0.000000000000000000, 0.1250000000000000000, 0.2500000000000000000, 0.3750000000000000000, 0.5000000000000000000, 0.6250000000000000000, 0.7500000000000000000, 0.8750000000000000000, 1.000000000000000000 ),
 .UNSPECIFIED. ) ;
#11853=CARTESIAN_POINT ( 'NONE',  ( -5.018808260229000062, -78.58054015155998684, -9.843244246394000641 ) ) ;
#11858=ORIENTED_EDGE ( 'NONE', *, *, #11036, .T. ) ;
#11859=CARTESIAN_POINT ( 'NONE',  ( -8.599335516584035943, -77.20000000000000284, 6.732869530217218568 ) ) ;
#11867=CARTESIAN_POINT ( 'NONE',  ( -9.487842642213001554, -77.64981427748799092, -0.8069809344748999358 ) ) ;
#11877=CARTESIAN_POINT ( 'NONE',  ( -7.604423127187000198, -79.80575956708399588, 7.914351627518998455 ) ) ;
#11884=ORIENTED_EDGE ( 'NONE', *, *, #37094, .F. ) ;
#11887=CARTESIAN_POINT ( 'NONE',  ( -6.760013919724102038, -78.12708333333334565, 8.796335266379953666 ) ) ;
#11889=CARTESIAN_POINT ( 'NONE',  ( 1.712298698931000063, -78.10580131689799543, 11.02540857285000087 ) ) ;
#11908=CARTESIAN_POINT ( 'NONE',  ( -3.364651265678953340, -78.19549771079697109, -8.616567145014089490 ) ) ;
#11909=CARTESIAN_POINT ( 'NONE',  ( 9.236725725698626377, -79.26122289752220240, 1.304468322093308652 ) ) ;
#11913=CARTESIAN_POINT ( 'NONE',  ( -6.861508235578342330, -77.54162168376055320, 6.204469612445603133 ) ) ;
#11916=CARTESIAN_POINT ( 'NONE',  ( -5.351292223237999579, -77.75163212332799390, 8.095330809056001442 ) ) ;
#11920=CARTESIAN_POINT ( 'NONE',  ( 8.693423296916000353, -80.00478354744298315, -7.148151291522000683 ) ) ;
#11931=CARTESIAN_POINT ( 'NONE',  ( 2.398305471015380608, -78.45419662550813200, 8.954209520413279222 ) ) ;
#11934=CARTESIAN_POINT ( 'NONE',  ( -4.084322113587999681, -80.33425248214398096, 10.29083287403000035 ) ) ;
#11938=AXIS2_PLACEMENT_3D ( 'NONE', #7699, #26275, #25983 ) ;
#11946=CARTESIAN_POINT ( 'NONE',  ( -1.840794636227000014, -80.06647572818799574, -9.354253787032998702 ) ) ;
#11952=CARTESIAN_POINT ( 'NONE',  ( 10.95453373411999998, -77.56775829503899899, 1.498774166161999988 ) ) ;
#11957=CARTESIAN_POINT ( 'NONE',  ( -9.467475792354999697, -77.25345539031198427, 1.978357023055999919 ) ) ;
#11958=CARTESIAN_POINT ( 'NONE',  ( -8.082524092276896610, -78.45833333333331439, 4.658475568430797686 ) ) ;
#11962=ADVANCED_FACE ( 'NONE', ( #11059 ), #49881, .T. ) ;
#11974=VERTEX_POINT ( 'NONE', #51502 ) ;
#11990=CARTESIAN_POINT ( 'NONE',  ( -7.000000000000000000, -81.19999999999998863, 0.000000000000000000 ) ) ;
#11998=CARTESIAN_POINT ( 'NONE',  ( 10.69999999999999929, -76.39999999999999147, 0.000000000000000000 ) ) ;
#12021=CARTESIAN_POINT ( 'NONE',  ( -1.535759092668000036, -78.84482872126899622, 9.397436897434999992 ) ) ;
#12033=CARTESIAN_POINT ( 'NONE',  ( 0.1286847231337999997, -79.24487755444098980, 10.93943584368999922 ) ) ;
#12035=CARTESIAN_POINT ( 'NONE',  ( -8.309722314488999118, -79.75160881430899451, 6.932476156777000575 ) ) ;
#12039=ORIENTED_EDGE ( 'NONE', *, *, #18169, .F. ) ;
#12042=CARTESIAN_POINT ( 'NONE',  ( -9.387315177295000979, -80.10788932539801976, 2.697965643110000311 ) ) ;
#12055=CARTESIAN_POINT ( 'NONE',  ( 11.00000000000000355, -79.83958333333332291, -1.439896632895299566 ) ) ;
#12063=DIRECTION ( 'NONE',  ( 0.000000000000000000, 0.000000000000000000, -1.000000000000000000 ) ) ;
#12067=CARTESIAN_POINT ( 'NONE',  ( 9.035852695838000770, -77.23166978779399017, 2.902309323059000246 ) ) ;
#12072=CARTESIAN_POINT ( 'NONE',  ( 5.949632932387999951, -77.94810873382799343, -7.711132450962999485 ) ) ;
#12078=ORIENTED_EDGE ( 'NONE', *, *, #58361, .F. ) ;
#12081=CARTESIAN_POINT ( 'NONE',  ( 7.875215672226593355, -79.45217620423241556, -5.395709537963816693 ) ) ;
#12085=CARTESIAN_POINT ( 'NONE',  ( 4.175433224444000224, -79.04683895522299508, 8.844688580446998571 ) ) ;
#12092=CONICAL_SURFACE ( 'NONE', #14905, 1.099999997148999986, 0.7853981633972997312 ) ;
#12098=CARTESIAN_POINT ( 'NONE',  ( 0.000000000000000000, -74.99999999999998579, 0.000000000000000000 ) ) ;
#12100=AXIS2_PLACEMENT_3D ( 'NONE', #17730, #3285, #57297 ) ;
#12108=ORIENTED_EDGE ( 'NONE', *, *, #50852, .F. ) ;
#12117=CARTESIAN_POINT ( 'NONE',  ( 0.9519614230518689268, -79.96731120637714696, 9.201533066724445931 ) ) ;
#12121=CARTESIAN_POINT ( 'NONE',  ( -5.117553686986000550, -78.70829163312599519, -10.03691081092000026 ) ) ;
#12122=CARTESIAN_POINT ( 'NONE',  ( 6.565127467646830972, -77.28787814322510030, -6.516269025712384533 ) ) ;
#12132=CARTESIAN_POINT ( 'NONE',  ( -7.138937464960999790, -79.48718652232298609, 8.574798629027000629 ) ) ;
#12136=CARTESIAN_POINT ( 'NONE',  ( 0.000000000000000000, -79.99999999999998579, 0.000000000000000000 ) ) ;
#12147=CARTESIAN_POINT ( 'NONE',  ( 8.085542028362999289, -77.84878108138998698, -5.029352477166999513 ) ) ;
#12149=ADVANCED_FACE ( 'NONE', ( #16347 ), #27638, .F. ) ;
#12154=CARTESIAN_POINT ( 'NONE',  ( -9.250000000000000000, -78.99999999999998579, 0.000000000000000000 ) ) ;
#12159=CARTESIAN_POINT ( 'NONE',  ( -1.297526016723000053, -78.48541891344798671, -10.89864408161000142 ) ) ;
#12167=CARTESIAN_POINT ( 'NONE',  ( 8.266242728491365099, -77.28744835287174908, 4.213564929189619335 ) ) ;
#12168=CARTESIAN_POINT ( 'NONE',  ( -1.439896632895359962, -78.08541666666666003, 10.99999999999999645 ) ) ;
#12170=CARTESIAN_POINT ( 'NONE',  ( 0.2682802194768000303, -79.30608152108499098, -11.26307951182000089 ) ) ;
#12177=EDGE_CURVE ( 'NONE', #38384, #30828, #37238, .T. ) ;
#12194=CARTESIAN_POINT ( 'NONE',  ( 9.249483092228999226, -79.25084128437099196, 0.09778817195952001218 ) ) ;
#12197=CARTESIAN_POINT ( 'NONE',  ( -6.557430175411668394, -77.53787113409947551, 6.523852457878298594 ) ) ;
#12198=CARTESIAN_POINT ( 'NONE',  ( 10.77519778174000109, -77.11087656805389656, -1.228540277667999892 ) ) ;
#12200=CARTESIAN_POINT ( 'NONE',  ( 9.051070938631999852, -77.60951297768299639, 3.499832029064999794 ) ) ;
#12204=CARTESIAN_POINT ( 'NONE',  ( -9.459258931978000717, -79.94904572086998940, 5.442530770145999952 ) ) ;
#12216=CARTESIAN_POINT ( 'NONE',  ( -0.2842604123649000170, -80.11603890021898167, -11.17811493562000003 ) ) ;
#12225=CARTESIAN_POINT ( 'NONE',  ( 5.169261753999999875, -79.69201159510198806, -7.880669826094999664 ) ) ;
#12227=CARTESIAN_POINT ( 'NONE',  ( -1.724324800276255454, -77.21249999999999147, -10.89830687840934864 ) ) ;
#12235=CARTESIAN_POINT ( 'NONE',  ( 4.790019567428999814, -77.96759421635398724, -9.965127559477000574 ) ) ;
#12241=CARTESIAN_POINT ( 'NONE',  ( -9.250000000000000000, -78.49999999999998579, 0.000000000000000000 ) ) ;
#12242=CARTESIAN_POINT ( 'NONE',  ( -11.00000000000000888, -77.58958333333332291, 1.439896632895276252 ) ) ;
#12264=ORIENTED_EDGE ( 'NONE', *, *, #3920, .T. ) ;
#12267=CYLINDRICAL_SURFACE ( 'NONE', #5768, 10.69999999999999929 ) ;
#12294=CARTESIAN_POINT ( 'NONE',  ( -10.71369944335147117, -79.72083333333331723, -2.879226727952084453 ) ) ;
#12304=CARTESIAN_POINT ( 'NONE',  ( -0.5506691749702000704, -78.01350959400299701, -9.615090921292999582 ) ) ;
#12308=ORIENTED_EDGE ( 'NONE', *, *, #2312, .T. ) ;
#12314=CARTESIAN_POINT ( 'NONE',  ( -10.93134324956000114, -78.37401457012799710, -0.4399444258272000030 ) ) ;
#12318=CARTESIAN_POINT ( 'NONE',  ( -8.227975111406001574, -79.81548455509199869, 6.864277664119000200 ) ) ;
#12337=CARTESIAN_POINT ( 'NONE',  ( 9.099688436573039496, -78.83571894269113045, -1.661325781669990453 ) ) ;
#12350=CARTESIAN_POINT ( 'NONE',  ( 9.489101650983998937, -77.20556042082598935, -0.1642684238307999811 ) ) ;
#12363=CARTESIAN_POINT ( 'NONE',  ( -8.340505669901505215, -79.20899701435310192, 4.714710602094070779 ) ) ;
#12368=CARTESIAN_POINT ( 'NONE',  ( 10.99999999999999645, -78.86041666666666572, 1.439896632895345974 ) ) ;
#12370=CARTESIAN_POINT ( 'NONE',  ( 9.470739325998000169, -78.94724519986900191, -1.171383596386999848 ) ) ;
#12373=ORIENTED_EDGE ( 'NONE', *, *, #23830, .F. ) ;
#12374=CARTESIAN_POINT ( 'NONE',  ( 7.000000000000000000, -81.10000000285099020, 0.000000000000000000 ) ) ;
#12396=CARTESIAN_POINT ( 'NONE',  ( -6.760013919724102038, -77.62708333333333144, 8.796335266379953666 ) ) ;
#12408=CARTESIAN_POINT ( 'NONE',  ( 11.14483649738000004, -79.38250813710999410, 1.649713251514000056 ) ) ;
#12409=CARTESIAN_POINT ( 'NONE',  ( 7.840108872306949195, -77.30560672394517496, -4.911361524887249530 ) ) ;
#12415=CYLINDRICAL_SURFACE ( 'NONE', #53022, 9.250000000000000000 ) ;
#12421=CARTESIAN_POINT ( 'NONE',  ( -3.607132791900000246, -79.65574064831898227, -10.55841809546000043 ) ) ;
#12428=DIRECTION ( 'NONE',  ( 1.000000000000000000, 0.000000000000000000, 0.000000000000000000 ) ) ;
#12443=CARTESIAN_POINT ( 'NONE',  ( 3.303001513109999898, -79.01917364576898706, -10.46681410869999951 ) ) ;
#12448=VERTEX_POINT ( 'NONE', #10906 ) ;
#12450=CARTESIAN_POINT ( 'NONE',  ( -0.01192727606575066587, -77.37492492956100421, 9.363670505352606810 ) ) ;
#12451=CARTESIAN_POINT ( 'NONE',  ( -11.00000000000000000, -77.59999999999999432, 0.000000000000000000 ) ) ;
#12452=CARTESIAN_POINT ( 'NONE',  ( 3.229284361504000334, -79.59469609652998656, 10.68004289648999894 ) ) ;
#12461=EDGE_LOOP ( 'NONE', ( #3122, #8607, #10005, #21969, #47 ) ) ;
#12465=CARTESIAN_POINT ( 'NONE',  ( -9.551084006840532936, -79.74233320338822750, 0.9337316140615163906 ) ) ;
#12471=EDGE_CURVE ( 'NONE', #30828, #45319, #39486, .T. ) ;
#12472=CARTESIAN_POINT ( 'NONE',  ( 0.06516443285433551336, -78.22564617984212987, -9.249726598108379605 ) ) ;
#12477=CARTESIAN_POINT ( 'NONE',  ( -6.545454099276200033, -77.53772617611215878, 6.535861892516707350 ) ) ;
#12478=CARTESIAN_POINT ( 'NONE',  ( 10.42639159904000046, -77.10027333183208498, -2.617796444239999687 ) ) ;
#12480=CARTESIAN_POINT ( 'NONE',  ( -1.182190922889000184, -78.94543294674498668, -9.631881180458998770 ) ) ;
#12484=CARTESIAN_POINT ( 'NONE',  ( -9.497876546326999403, -77.35168256874098347, -0.2008509664869000122 ) ) ;
#12485=CARTESIAN_POINT ( 'NONE',  ( -9.459258931978000717, -79.88874279519899346, 5.442530770145999952 ) ) ;
#12498=CARTESIAN_POINT ( 'NONE',  ( 9.007844276740291534, -79.37087089868364842, 2.420897759216547040 ) ) ;
#12499=CARTESIAN_POINT ( 'NONE',  ( -8.397876581538000096, -79.87585733274299571, 6.655340051815000102 ) ) ;
#12509=CARTESIAN_POINT ( 'NONE',  ( -3.827647950032363244, -78.04671362439400184, -10.14077206697919387 ) ) ;
#12518=CARTESIAN_POINT ( 'NONE',  ( 9.498848458907630743, -79.03416273108655332, 0.1004247326035953569 ) ) ;
#12523=FACE_OUTER_BOUND ( 'NONE', #22399, .T. ) ;
#12546=DIRECTION ( 'NONE',  ( 2.706894537570999990E-12, 1.000000000000000000, 1.232851854724000084E-11 ) ) ;
#12562=CARTESIAN_POINT ( 'NONE',  ( -8.724187533938204453, -78.62698228320140004, -3.074223295207495266 ) ) ;
#12574=EDGE_CURVE ( 'NONE', #28211, #25253, #40503, .T. ) ;
#12579=CARTESIAN_POINT ( 'NONE',  ( 8.212410987726999068, -78.00373067278798089, -6.936771999183999782 ) ) ;
#12587=CARTESIAN_POINT ( 'NONE',  ( 1.846868607710999921, -78.81640489213999956, 9.341276817324001058 ) ) ;
#12594=CARTESIAN_POINT ( 'NONE',  ( 1.439896632895302009, -78.83541666666664582, -11.00000000000000000 ) ) ;
#12598=CARTESIAN_POINT ( 'NONE',  ( 10.94008345411999983, -78.12118338113400284, 0.05084573220516999670 ) ) ;
#12601=CARTESIAN_POINT ( 'NONE',  ( 11.28909814340999951, -79.98006123089598418, -1.860932571041999939 ) ) ;
#12603=B_SPLINE_CURVE_WITH_KNOTS ( 'NONE', 3,
 ( #8318, #22480, #17767, #40490, #31612, #22771, #40781, #45519, #18355, #44332, #36345, #48773, #39895, #31024, #50821, #10960, #32776, #10365 ),
 .UNSPECIFIED., .F., .F.,
 ( 4, 2, 2, 2, 2, 2, 2, 2, 4 ),
 ( 0.000000000000000000, 0.1249999999999999445, 0.2500000000000000000, 0.3750000000000000555, 0.5000000000000001110, 0.6250000000000000000, 0.7500000000000000000, 0.8749999999999998890, 1.000000000000000000 ),
 .UNSPECIFIED. ) ;
#12609=CARTESIAN_POINT ( 'NONE',  ( 3.366547962069000199, -79.90301558626953238, -9.168809063548000182 ) ) ;
#12610=ORIENTED_EDGE ( 'NONE', *, *, #19106, .T. ) ;
#12611=CARTESIAN_POINT ( 'NONE',  ( -9.250000000000000000, -79.09999999999999432, 1.813240672189999963E-14 ) ) ;
#12622=CARTESIAN_POINT ( 'NONE',  ( 8.564407298655666523, -78.81931219690746104, -3.494578516088384657 ) ) ;
#12624=DIRECTION ( 'NONE',  ( 0.000000000000000000, 0.7071067811866525998, -0.7071067811864425456 ) ) ;
#12628=LINE ( 'NONE', #30331, #8480 ) ;
#12638=CARTESIAN_POINT ( 'NONE',  ( -3.759408710945999488, -77.04890421901679076, -8.530078903752000841 ) ) ;
#12644=DIRECTION ( 'NONE',  ( 1.000000000000000000, 0.000000000000000000, 0.000000000000000000 ) ) ;
#12650=CARTESIAN_POINT ( 'NONE',  ( 5.649609181776704681, -79.42525939925479861, -7.715451315860589965 ) ) ;
#12654=CARTESIAN_POINT ( 'NONE',  ( -8.050862028188001673, -79.15888192999699413, 5.553975462107000105 ) ) ;
#12666=CYLINDRICAL_SURFACE ( 'NONE', #50538, 9.549999999999998934 ) ;
#12673=CARTESIAN_POINT ( 'NONE',  ( -5.726462542197000793, -79.84499576192899895, -7.912542777261000637 ) ) ;
#12681=CARTESIAN_POINT ( 'NONE',  ( -4.475319841928504516, -78.93676327900720935, -8.610768833002914846 ) ) ;
#12687=CARTESIAN_POINT ( 'NONE',  ( 3.538064976920356042, -79.94385801930759783, 8.546548758931297840 ) ) ;
#12688=CARTESIAN_POINT ( 'NONE',  ( 10.93619165073445210, -80.21437323052235513, 1.947132623917049887 ) ) ;
#12690=CARTESIAN_POINT ( 'NONE',  ( -4.391024480082000636, -79.21395401111398371, -10.37534762698999913 ) ) ;
#12692=CARTESIAN_POINT ( 'NONE',  ( -2.463318457235554426, -77.20365170611822236, -8.921952837938405878 ) ) ;
#12700=CARTESIAN_POINT ( 'NONE',  ( 7.917622607290999426, -78.86915472700400187, 7.861478989701000231 ) ) ;
#12722=VECTOR ( 'NONE', #27010, 1000.000000000000114 ) ;
#12726=CARTESIAN_POINT ( 'NONE',  ( 4.038786804788999873, -79.58513894942799993, -10.20549938643999965 ) ) ;
#12735=CARTESIAN_POINT ( 'NONE',  ( -10.83342013959000028, -78.72383311221699387, 2.669945268378000058 ) ) ;
#12756=CARTESIAN_POINT ( 'NONE',  ( -6.041084908348863358, -78.16847799058953683, -7.008332470365363775 ) ) ;
#12760=CARTESIAN_POINT ( 'NONE',  ( -7.162195376558232240, -77.54552129972844909, 5.853735638857269663 ) ) ;
#12761=CARTESIAN_POINT ( 'NONE',  ( -10.47078769031000078, -77.83521312279499682, -3.499536356729999742 ) ) ;
#12764=CARTESIAN_POINT ( 'NONE',  ( -1.959694873104000257, -77.43897000290898802, -9.504225410855001499 ) ) ;
#12768=CARTESIAN_POINT ( 'NONE',  ( -10.55592303174000079, -80.01864766310099242, -3.904632140253000205 ) ) ;
#12772=EDGE_CURVE ( 'NONE', #32566, #41582, #35167, .T. ) ;
#12777=DIRECTION ( 'NONE',  ( 3.944178317128000824E-11, 1.000000000000000000, -1.496715540702999877E-09 ) ) ;
#12781=CARTESIAN_POINT ( 'NONE',  ( -11.10900444195999981, -80.10274572043100250, 2.566683358663000014 ) ) ;
#12787=CARTESIAN_POINT ( 'NONE',  ( 0.000000000000000000, -76.19999999999998863, 0.000000000000000000 ) ) ;
#12805=CARTESIAN_POINT ( 'NONE',  ( -9.429275737370000243, -77.40017060862199116, -1.157047565421999824 ) ) ;
#12812=EDGE_CURVE ( 'NONE', #13297, #16896, #33874, .T. ) ;
#12828=ORIENTED_EDGE ( 'NONE', *, *, #14062, .T. ) ;
#12829=CARTESIAN_POINT ( 'NONE',  ( 4.099999999699000419, -75.20000000030088927, -8.298664203784000017E-10 ) ) ;
#12844=CARTESIAN_POINT ( 'NONE',  ( -8.867285139540818761, -78.62306678270786620, -2.634614563402982501 ) ) ;
#12864=B_SPLINE_CURVE_WITH_KNOTS ( 'NONE', 3,
 ( #57134, #18074, #22785, #39125, #21119, #7545, #13627, #30254, #25258, #53797, #48294, #43862, #48011, #4495, #22493, #11697, #43562, #34681 ),
 .UNSPECIFIED., .F., .F.,
 ( 4, 2, 2, 2, 2, 2, 2, 2, 4 ),
 ( 0.000000000000000000, 0.1250000000000000278, 0.2500000000000000555, 0.3750000000000001665, 0.5000000000000001110, 0.6250000000000001110, 0.7500000000000002220, 0.8750000000000001110, 1.000000000000000000 ),
 .UNSPECIFIED. ) ;
#12867=CARTESIAN_POINT ( 'NONE',  ( -5.062255795481000575, -77.53733258133598838, -8.064983548927001422 ) ) ;
#12872=CIRCLE ( 'NONE', #28893, 1.199999999999999734 ) ;
#12879=EDGE_CURVE ( 'NONE', #23736, #35917, #17938, .T. ) ;
#12880=CARTESIAN_POINT ( 'NONE',  ( 9.601044633201999190, -79.16060049144299171, 5.244783912358999878 ) ) ;
#12882=CARTESIAN_POINT ( 'NONE',  ( 1.802966087674999995, -80.16922046769499843, 11.18561714559999842 ) ) ;
#12885=VERTEX_POINT ( 'NONE', #36228 ) ;
#12887=EDGE_CURVE ( 'NONE', #21042, #18942, #53697, .T. ) ;
#12890=EDGE_CURVE ( 'NONE', #27720, #29378, #3710, .T. ) ;
#12893=ORIENTED_EDGE ( 'NONE', *, *, #52449, .T. ) ;
#12902=CARTESIAN_POINT ( 'NONE',  ( 9.079299172193310952, -78.83476146753204716, -1.768634379958562208 ) ) ;
#12909=CARTESIAN_POINT ( 'NONE',  ( 9.611650271896820641, -77.89166666666666572, 5.539808784079911952 ) ) ;
#12922=DIRECTION ( 'NONE',  ( 0.000000000000000000, -1.000000000000000000, 0.000000000000000000 ) ) ;
#12930=DIRECTION ( 'NONE',  ( -1.000000000000000000, 0.000000000000000000, 0.000000000000000000 ) ) ;
#12933=CARTESIAN_POINT ( 'NONE',  ( 9.634996601833998753, -79.94318275341397850, -1.682215218792999956 ) ) ;
#12945=CARTESIAN_POINT ( 'NONE',  ( 10.99860714806000139, -77.19003472681939115, 1.508735257010000108 ) ) ;
#12949=AXIS2_PLACEMENT_3D ( 'NONE', #10769, #11351, #52082 ) ;
#12951=CARTESIAN_POINT ( 'NONE',  ( 8.985706068735000329, -79.48779652109199390, -3.828549499589000149 ) ) ;
#12967=CARTESIAN_POINT ( 'NONE',  ( -2.858407197967999913, -79.99999999999998579, 8.797272775729998884 ) ) ;
#12971=CARTESIAN_POINT ( 'NONE',  ( -7.707335466132000157, -79.18586165678098610, -8.217415310065000256 ) ) ;
#12979=CARTESIAN_POINT ( 'NONE',  ( -10.57172952804012667, -80.44999999999998863, -2.251292830071324857 ) ) ;
#12980=CARTESIAN_POINT ( 'NONE',  ( 3.357763675545999860, -79.20626297899599422, -10.64034880800999971 ) ) ;
#13006=CARTESIAN_POINT ( 'NONE',  ( 3.915498778898000687, -79.27612305176899099, 10.25343288338999947 ) ) ;
#13016=CARTESIAN_POINT ( 'NONE',  ( 1.439896632895333539, -77.73541666666666572, -10.99999999999999822 ) ) ;
#13017=EDGE_CURVE ( 'NONE', #52316, #17327, #29162, .T. ) ;
#13018=CARTESIAN_POINT ( 'NONE',  ( -10.97221500190000043, -79.25758784453798000, -2.025363574538999956 ) ) ;
#13033=CARTESIAN_POINT ( 'NONE',  ( -6.383854037583304830, -79.81686861624592666, -7.133078034627309272 ) ) ;
#13039=CARTESIAN_POINT ( 'NONE',  ( -3.536609267268810974, -78.19392279636586807, -8.547114838364091582 ) ) ;
#13044=CARTESIAN_POINT ( 'NONE',  ( 0.4664785593013082154, -77.47109208897903443, 9.249934602145987839 ) ) ;
#13045=CARTESIAN_POINT ( 'NONE',  ( -1.996894868142000012, -77.25932187515898875, 10.85801781015000067 ) ) ;
#13047=CARTESIAN_POINT ( 'NONE',  ( 1.487026788147999934, -77.46739383203798468, -9.589549613196998834 ) ) ;
#13052=CARTESIAN_POINT ( 'NONE',  ( -1.870137171474999915, -79.98156414243598533, -11.09839649295000008 ) ) ;
#13066=CARTESIAN_POINT ( 'NONE',  ( 5.496473448154000074, -80.39148163303399031, 9.863667302640999779 ) ) ;
#13077=CARTESIAN_POINT ( 'NONE',  ( -6.382469709265000013, -79.95501551942399487, 6.934717328048000340 ) ) ;
#13079=CARTESIAN_POINT ( 'NONE',  ( 11.00000000000000178, -77.34374999999998579, -0.8639379797371515846 ) ) ;
#13099=CARTESIAN_POINT ( 'NONE',  ( 0.000000000000000000, -80.49999999999998579, 0.000000000000000000 ) ) ;
#13116=CARTESIAN_POINT ( 'NONE',  ( -8.283402485400999993, -77.90747789361365960, -7.298588567666998372 ) ) ;
#13123=CARTESIAN_POINT ( 'NONE',  ( -8.073459667400001649, -78.25635051282399957, -5.384232384047000330 ) ) ;
#13130=CARTESIAN_POINT ( 'NONE',  ( -8.823800648792902379, -78.62434323315024187, -2.778829492415963553 ) ) ;
#13139=CARTESIAN_POINT ( 'NONE',  ( 9.250000000000000000, -78.74999999999998579, 0.000000000000000000 ) ) ;
#13144=DIRECTION ( 'NONE',  ( -1.000000000000000000, 0.000000000000000000, 0.000000000000000000 ) ) ;
#13145=CARTESIAN_POINT ( 'NONE',  ( -5.539808784079887083, -79.28333333333333144, -9.611650271896841957 ) ) ;
#13151=VERTEX_POINT ( 'NONE', #20821 ) ;
#13156=CARTESIAN_POINT ( 'NONE',  ( -9.171168281578999881, -77.93526618914198423, 2.561259179188999813 ) ) ;
#13165=ORIENTED_EDGE ( 'NONE', *, *, #45440, .T. ) ;
#13167=CARTESIAN_POINT ( 'NONE',  ( -6.898009915208000109, -79.44152403476999780, -8.491482529321999095 ) ) ;
#13170=ORIENTED_EDGE ( 'NONE', *, *, #125, .T. ) ;
#13181=CARTESIAN_POINT ( 'NONE',  ( -9.250000000000000000, -79.59999999999999432, 0.000000000000000000 ) ) ;
#13182=ORIENTED_EDGE ( 'NONE', *, *, #1611, .T. ) ;
#13185=CARTESIAN_POINT ( 'NONE',  ( 7.395663543987498478, -79.29799491392495270, -5.683475073351669238 ) ) ;
#13194=CARTESIAN_POINT ( 'NONE',  ( 11.00000000000000000, -79.84999999999999432, 0.000000000000000000 ) ) ;
#13200=CARTESIAN_POINT ( 'NONE',  ( 6.760013919724039866, -77.92291666666667993, 8.796335266379998075 ) ) ;
#13203=FACE_BOUND ( 'NONE', #53792, .T. ) ;
#13209=CARTESIAN_POINT ( 'NONE',  ( -9.250000000000000000, -78.59999999999999432, 0.000000000000000000 ) ) ;
#13228=CARTESIAN_POINT ( 'NONE',  ( -4.299999999999999822, -74.99999999999998579, 0.000000000000000000 ) ) ;
#13243=CARTESIAN_POINT ( 'NONE',  ( 0.000000000000000000, -74.64999999999999147, 0.000000000000000000 ) ) ;
#13249=CARTESIAN_POINT ( 'NONE',  ( 8.193575559979001000, -79.06565196373898630, 5.316613930189999948 ) ) ;
#13259=CARTESIAN_POINT ( 'NONE',  ( -7.844108077142347035, -77.79981011384823830, 5.713474972744468694 ) ) ;
#13267=CARTESIAN_POINT ( 'NONE',  ( 8.240432763520827208, -79.88799569061337991, 4.201471099154182376 ) ) ;
#13276=CARTESIAN_POINT ( 'NONE',  ( 11.03731426084000056, -79.31863239632698992, 1.633797283747999929 ) ) ;
#13292=CARTESIAN_POINT ( 'NONE',  ( 8.959721679174998954, -77.36557598619799592, -3.223936051704999972 ) ) ;
#13297=VERTEX_POINT ( 'NONE', #49447 ) ;
#13303=CARTESIAN_POINT ( 'NONE',  ( -6.920341278396000106, -79.50086188642998763, -8.518972542050999408 ) ) ;
#13313=CARTESIAN_POINT ( 'NONE',  ( 4.105747930350998942, -79.39804961620099277, -10.37470161445000016 ) ) ;
#13316=EDGE_CURVE ( 'NONE', #18942, #48890, #1, .T. ) ;
#13319=DIRECTION ( 'NONE',  ( 0.000000000000000000, -0.7071067811866525998, -0.7071067811864425456 ) ) ;
#13322=ORIENTED_EDGE ( 'NONE', *, *, #17478, .F. ) ;
#13325=DIRECTION ( 'NONE',  ( -1.000000000000000000, 0.000000000000000000, 0.000000000000000000 ) ) ;
#13326=VERTEX_POINT ( 'NONE', #26980 ) ;
#13328=ORIENTED_EDGE ( 'NONE', *, *, #15451, .T. ) ;
#13333=CARTESIAN_POINT ( 'NONE',  ( -4.898542333728430620, -78.18064372240367277, -7.846565971572500686 ) ) ;
#13338=CARTESIAN_POINT ( 'NONE',  ( 1.272989083314503000, -77.46403964825013588, 9.162259919681792653 ) ) ;
#13340=CARTESIAN_POINT ( 'NONE',  ( 10.74764839381999870, -78.11818400912298443, -0.2248421733643000131 ) ) ;
#13343=CARTESIAN_POINT ( 'NONE',  ( 7.658860137760000519, -78.69307375199699095, 5.959242465009999989 ) ) ;
#13352=EDGE_LOOP ( 'NONE', ( #28667, #43197, #9879, #1898 ) ) ;
#13359=DIRECTION ( 'NONE',  ( 1.000000000000000000, 0.000000000000000000, 0.000000000000000000 ) ) ;
#13365=CARTESIAN_POINT ( 'NONE',  ( 11.00000000000000000, -79.94999999999998863, 0.000000000000000000 ) ) ;
#13372=B_SPLINE_CURVE_WITH_KNOTS ( 'NONE', 3,
 ( #29356, #47403, #56822, #21373, #38803, #48268, #30515, #20798, #34360, #2514, #26087, #48544, #56245, #20231, #29928, #16669, #47977, #7224 ),
 .UNSPECIFIED., .F., .F.,
 ( 4, 2, 2, 2, 2, 2, 2, 2, 4 ),
 ( 0.000000000000000000, 0.1250000000000000000, 0.2500000000000000000, 0.3750000000000000000, 0.5000000000000000000, 0.6250000000000000000, 0.7500000000000000000, 0.8750000000000000000, 1.000000000000000000 ),
 .UNSPECIFIED. ) ;
#13374=DIRECTION ( 'NONE',  ( 0.000000000000000000, 0.000000000000000000, -1.000000000000000000 ) ) ;
#13375=CARTESIAN_POINT ( 'NONE',  ( -3.399186938124999724, -77.19999999999998863, -10.46162167925000119 ) ) ;
#13385=CARTESIAN_POINT ( 'NONE',  ( 9.208615812369000508, -77.16518630590849170, 2.957800710608999850 ) ) ;
#13402=FILL_AREA_STYLE ('',( #39409 ) ) ;
#13406=AXIS2_PLACEMENT_3D ( 'NONE', #47417, #42971, #1664 ) ;
#13413=LINE ( 'NONE', #8405, #46978 ) ;
#13419=CARTESIAN_POINT ( 'NONE',  ( 5.091895231007000255, -78.54058880411299981, 8.260951054388000259 ) ) ;
#13433=CARTESIAN_POINT ( 'NONE',  ( 0.000000000000000000, -74.64999999999999147, 0.000000000000000000 ) ) ;
#13440=CARTESIAN_POINT ( 'NONE',  ( 9.611650271896843734, -79.40833333333331723, -5.539808784079876425 ) ) ;
#13444=EDGE_CURVE ( 'NONE', #28960, #29374, #2796, .T. ) ;
#13449=B_SPLINE_CURVE_WITH_KNOTS ( 'NONE', 3,
 ( #28249, #18837, #46304, #23834, #49553, #45126, #4677, #22676, #40687, #19710, #2580, #43023, #56308, #43308, #33562, #29707, #37708, #24130 ),
 .UNSPECIFIED., .F., .F.,
 ( 4, 2, 2, 2, 2, 2, 2, 2, 4 ),
 ( 0.000000000000000000, 0.1250000000000000000, 0.2500000000000000000, 0.3750000000000000000, 0.5000000000000000000, 0.6250000000000000000, 0.7500000000000000000, 0.8750000000000000000, 1.000000000000000000 ),
 .UNSPECIFIED. ) ;
#13453=CARTESIAN_POINT ( 'NONE',  ( -8.130434485062000505, -77.24008885281497783, -7.810376049085999917 ) ) ;
#13456=CARTESIAN_POINT ( 'NONE',  ( 7.653824198668000456, -79.22136658247099206, -5.479973919995999587 ) ) ;
#13464=ADVANCED_FACE ( 'NONE', ( #15161 ), #33157, .F. ) ;
#13465=ORIENTED_EDGE ( 'NONE', *, *, #18652, .T. ) ;
#13471=CIRCLE ( 'NONE', #38923, 1.000000000000000000 ) ;
#13479=CARTESIAN_POINT ( 'NONE',  ( -5.809791519574999619, -79.67570697846352346, 7.851562197947999699 ) ) ;
#13480=B_SPLINE_SURFACE_WITH_KNOTS ( 'NONE', 3, 3, ( 
 ( #37169, #6460, #33889, #46933, #37457, #33607, #51930, #24473, #42487, #38329, #51649 ),
 ( #28295, #46641, #19173, #15904, #1763, #11489, #51351, #14723, #51064, #32720, #11200 ),
 ( #24178, #56352, #24765, #2057, #1471, #19757, #29177, #15023, #29462, #37754, #41897 ),
 ( #47224, #15323, #5578, #20058, #23589, #10910, #6755, #41603, #1183, #55181, #50772 ) ),
 .UNSPECIFIED., .F., .F., .F.,
 ( 4, 4 ),
 ( 4, 1, 1, 1, 1, 1, 1, 1, 4 ),
 ( 0.1070361703151999910, 1.138757407831999968 ),
 ( -0.003449459057608000173, 0.01897202481685000136, 0.04139350869129999888, 0.06381499256575000334, 0.08623647644019999392, 0.1086579603147000000, 0.1310794441891000028, 0.1535009280635999951, 0.1759224119379999840 ),
 .UNSPECIFIED. ) ;
#13494=CARTESIAN_POINT ( 'NONE',  ( 3.246408215754346127, -78.75374379457647933, -8.682844942750486794 ) ) ;
#13496=CARTESIAN_POINT ( 'NONE',  ( 8.796335266379966100, -78.40208333333335133, 6.760013919724084275 ) ) ;
#13502=CARTESIAN_POINT ( 'NONE',  ( -1.842497806997728027, -79.98834702216801418, 10.91026042240053862 ) ) ;
#13503=CARTESIAN_POINT ( 'NONE',  ( -0.3558927676304953214, -79.99999999999994316, 9.287066994265805064 ) ) ;
#13510=DIRECTION ( 'NONE',  ( 0.000000000000000000, -1.000000000000000000, 0.000000000000000000 ) ) ;
#13511=ADVANCED_FACE ( 'NONE', ( #50905 ), #41452, .T. ) ;
#13526=CARTESIAN_POINT ( 'NONE',  ( 7.686826547751000938, -78.63180575231598368, 5.981002702827999506 ) ) ;
#13543=CARTESIAN_POINT ( 'NONE',  ( 7.847929611857001220, -77.11666530948868115, -7.852092130568000705 ) ) ;
#13545=CARTESIAN_POINT ( 'NONE',  ( -7.000000000000000000, -81.19999999999998863, -1.000000000000000000 ) ) ;
#13550=CARTESIAN_POINT ( 'NONE',  ( -4.465297566879000257, -79.74293539630998850, 8.686876450551999085 ) ) ;
#13561=AXIS2_PLACEMENT_3D ( 'NONE', #29211, #2940, #11522 ) ;
#13562=CARTESIAN_POINT ( 'NONE',  ( 2.260091721765999928, -78.89370578835476522, -9.437303113984999214 ) ) ;
#13564=CARTESIAN_POINT ( 'NONE',  ( 6.989933869880151640, -79.90691905236667480, 6.058301176545876743 ) ) ;
#13565=CARTESIAN_POINT ( 'NONE',  ( -9.497876546326999403, -77.25168256874098915, -0.2008509664869000122 ) ) ;
#13567=CARTESIAN_POINT ( 'NONE',  ( -9.497876546326999403, -77.35168256874098347, -0.2008509664869000122 ) ) ;
#13570=CARTESIAN_POINT ( 'NONE',  ( 0.000000000000000000, -80.99999999999998579, -8.199999999999970868 ) ) ;
#13596=CARTESIAN_POINT ( 'NONE',  ( -5.755176823513999729, -78.34907535878998885, 9.345691860246999383 ) ) ;
#13611=CARTESIAN_POINT ( 'NONE',  ( 0.1312417595986999919, -79.11712607287400090, 11.15680847095000061 ) ) ;
#13627=CARTESIAN_POINT ( 'NONE',  ( 4.658475568430830549, -79.66666666666665719, -8.082524092276877070 ) ) ;
#13630=CARTESIAN_POINT ( 'NONE',  ( -4.672105271192539711, -78.18294966887039266, -7.983815220272783009 ) ) ;
#13635=EDGE_LOOP ( 'NONE', ( #55760, #51233, #57731, #50765 ) ) ;
#13637=CARTESIAN_POINT ( 'NONE',  ( -0.006254617009199966819, -77.47520766586539764, 9.249905062637703068 ) ) ;
#13638=CARTESIAN_POINT ( 'NONE',  ( 10.90987126150000108, -77.25268889183898580, 1.690571823134000118 ) ) ;
#13641=CARTESIAN_POINT ( 'NONE',  ( -1.565122400816999937, -78.77834523938398092, 9.577113408380000692 ) ) ;
#13646=CARTESIAN_POINT ( 'NONE',  ( -4.969435546850999863, -78.51666441077600211, -9.746410964130999943 ) ) ;
#13657=DIRECTION ( 'NONE',  ( 0.000000000000000000, 0.000000000000000000, -1.000000000000000000 ) ) ;
#13659=CARTESIAN_POINT ( 'NONE',  ( 10.99801204134999999, -80.34957387780099225, -3.007190593213000085 ) ) ;
#13690=FACE_OUTER_BOUND ( 'NONE', #40355, .T. ) ;
#13691=ADVANCED_FACE ( 'NONE', ( #45879 ), #49317, .F. ) ;
#13704=CARTESIAN_POINT ( 'NONE',  ( -9.254388464354001087, -79.80752053325198858, 5.469807505829999528 ) ) ;
#13715=CARTESIAN_POINT ( 'NONE',  ( -1.565122400816999937, -78.59743646237099313, 9.577113408380000692 ) ) ;
#13737=CARTESIAN_POINT ( 'NONE',  ( -7.809619239761000031, -79.88027893010598746, -5.839499659979000334 ) ) ;
#13747=CARTESIAN_POINT ( 'NONE',  ( 9.333674174720000494, -78.19108065130299678, -1.884914489352999878 ) ) ;
#13775=CARTESIAN_POINT ( 'NONE',  ( 5.642655093990001092, -79.27719169461070692, -7.355059082576608454 ) ) ;
#13782=CARTESIAN_POINT ( 'NONE',  ( 6.922474547212758900, -78.79240049070052976, -6.137042015094014147 ) ) ;
#13785=CARTESIAN_POINT ( 'NONE',  ( -5.684882048478777428, -77.67303331842424541, -7.397090001915298529 ) ) ;
#13806=CYLINDRICAL_SURFACE ( 'NONE', #19425, 11.00000000000000000 ) ;
#13807=LINE ( 'NONE', #45719, #40188 ) ;
#13811=ORIENTED_EDGE ( 'NONE', *, *, #50627, .T. ) ;
#13822=CARTESIAN_POINT ( 'NONE',  ( -9.480927541711999140, -78.34756746102598868, -2.229732866345000009 ) ) ;
#13827=CARTESIAN_POINT ( 'NONE',  ( 10.71369944335147473, -78.82916666666667993, -2.879226727952063580 ) ) ;
#13837=CARTESIAN_POINT ( 'NONE',  ( -10.35967608510999938, -78.02428934957498541, -4.287644625136000087 ) ) ;
#13840=VERTEX_POINT ( 'NONE', #9569 ) ;
#13842=CARTESIAN_POINT ( 'NONE',  ( -9.358268528169000788, -79.29296057154398625, -2.797054701638000296 ) ) ;
#13843=ORIENTED_EDGE ( 'NONE', *, *, #47920, .F. ) ;
#13849=ADVANCED_FACE ( 'NONE', ( #13690 ), #41476, .T. ) ;
#13857=CARTESIAN_POINT ( 'NONE',  ( 4.545264886168000729, -77.58620964842175738, 8.573871732259998879 ) ) ;
#13858=CARTESIAN_POINT ( 'NONE',  ( 6.330346032565856262, -79.91530064090616747, 6.754712701908596628 ) ) ;
#13862=CARTESIAN_POINT ( 'NONE',  ( 2.858906827459719580, -77.25017575896374922, -8.796993064675801222 ) ) ;
#13874=DIRECTION ( 'NONE',  ( 0.000000000000000000, 0.000000000000000000, -1.000000000000000000 ) ) ;
#13884=CARTESIAN_POINT ( 'NONE',  ( -9.596198845516999754, -77.71369001827098089, -0.8161970854479000392 ) ) ;
#13892=CARTESIAN_POINT ( 'NONE',  ( -7.508490145779999736, -78.99519950844198490, -8.005410190140000992 ) ) ;
#13898=AXIS2_PLACEMENT_3D ( 'NONE', #14645, #50398, #9947 ) ;
#13905=CARTESIAN_POINT ( 'NONE',  ( 3.941639820121999094, -79.15290945932498801, 10.32188786877999931 ) ) ;
#13917=FACE_OUTER_BOUND ( 'NONE', #5637, .T. ) ;
#13924=CARTESIAN_POINT ( 'NONE',  ( -6.457621509944139859, -78.16366907265800990, -6.622725915400998531 ) ) ;
#13930=CARTESIAN_POINT ( 'NONE',  ( 2.155228666668488557, -77.45640456078321279, 8.995333024866518201 ) ) ;
#13931=CARTESIAN_POINT ( 'NONE',  ( -4.789974786805000662, -77.95913546579699016, -9.946872946892002076 ) ) ;
#13932=CARTESIAN_POINT ( 'NONE',  ( -9.247932426686000795, -77.50168256874098915, -0.1955654147372000162 ) ) ;
#13933=CARTESIAN_POINT ( 'NONE',  ( -8.680270256945998852, -77.29685085726399052, 3.860428508128000313 ) ) ;
#13939=CARTESIAN_POINT ( 'NONE',  ( 10.28297802758999957, -78.15146380445199270, -3.734674224488999883 ) ) ;
#13952=CARTESIAN_POINT ( 'NONE',  ( 3.151000900302999952, -77.92702448625199452, 8.870309342620000592 ) ) ;
#13959=CARTESIAN_POINT ( 'NONE',  ( -9.083128615135207085, -77.12447916667788661, 2.440148005863599145 ) ) ;
#13963=CARTESIAN_POINT ( 'NONE',  ( -1.439896632895311113, -79.81458333333331723, -11.00000000000000355 ) ) ;
#13989=ORIENTED_EDGE ( 'NONE', *, *, #46593, .F. ) ;
#14008=CARTESIAN_POINT ( 'NONE',  ( 9.045658679128999680, -78.98589546046697762, 3.115350657311999782 ) ) ;
#14029=CARTESIAN_POINT ( 'NONE',  ( 2.322774810132999690, -78.26209495713698061, -11.19403484768000112 ) ) ;
#14031=CYLINDRICAL_SURFACE ( 'NONE', #38736, 2.600000000000000089 ) ;
#14041=CARTESIAN_POINT ( 'NONE',  ( -10.88539795434999924, -77.76091993224399346, -2.484616007705999774 ) ) ;
#14042=EDGE_CURVE ( 'NONE', #24542, #1524, #1890, .T. ) ;
#14045=CARTESIAN_POINT ( 'NONE',  ( 8.631984821280999753, -78.73816148727799202, -3.755001005681000148 ) ) ;
#14062=EDGE_CURVE ( 'NONE', #26404, #28211, #2838, .T. ) ;
#14082=CARTESIAN_POINT ( 'NONE',  ( -1.552995512644810727, -78.71162349006438319, -9.118897746246291902 ) ) ;
#14086=CARTESIAN_POINT ( 'NONE',  ( -8.083004225747728810, -77.64177325540374852, -4.658611240203036630 ) ) ;
#14093=CARTESIAN_POINT ( 'NONE',  ( 9.392881678679827928, -79.99999999999998579, 1.479774839917263440 ) ) ;
#14101=CARTESIAN_POINT ( 'NONE',  ( 10.36873448126860886, -78.14542693329265433, -2.835127193485178054 ) ) ;
#14116=FACE_OUTER_BOUND ( 'NONE', #23920, .T. ) ;
#14119=CARTESIAN_POINT ( 'NONE',  ( 9.577678893670999116, -79.01112094065199187, -1.184610362647000148 ) ) ;
#14121=ORIENTED_EDGE ( 'NONE', *, *, #500, .F. ) ;
#14128=CARTESIAN_POINT ( 'NONE',  ( -1.544822269226999945, -77.17104737372439160, -11.21622675622000109 ) ) ;
#14132=CARTESIAN_POINT ( 'NONE',  ( -0.6514213267380000172, -79.77076566372298316, 9.745581310452999801 ) ) ;
#14138=ORIENTED_EDGE ( 'NONE', *, *, #26362, .F. ) ;
#14145=CARTESIAN_POINT ( 'NONE',  ( 6.811742960620783549, -79.90924285524151571, 6.259193223187502042 ) ) ;
#14147=ORIENTED_EDGE ( 'NONE', *, *, #44181, .F. ) ;
#14148=CARTESIAN_POINT ( 'NONE',  ( -8.324924863653999196, -77.20749743507077767, 4.923709561474999497 ) ) ;
#14151=VECTOR ( 'NONE', #13319, 1000.000000000000000 ) ;
#14170=CARTESIAN_POINT ( 'NONE',  ( -8.705161348370999974, -77.74211384739999176, -4.119875709756000148 ) ) ;
#14179=CARTESIAN_POINT ( 'NONE',  ( -10.65673661723999999, -78.97122537111499696, 2.626400817186000047 ) ) ;
#14191=AXIS2_PLACEMENT_3D ( 'NONE', #55214, #5049, #41062 ) ;
#14198=CARTESIAN_POINT ( 'NONE',  ( -4.985602094412718621, -78.53757981385534492, -9.778117948741643417 ) ) ;
#14200=ORIENTED_EDGE ( 'NONE', *, *, #44844, .T. ) ;
#14207=EDGE_CURVE ( 'NONE', #18212, #13840, #12603, .T. ) ;
#14215=CARTESIAN_POINT ( 'NONE',  ( -9.250000000000000000, -77.49999999999998579, -1.203901273580999948E-14 ) ) ;
#14218=CARTESIAN_POINT ( 'NONE',  ( 2.146749720031601250, -77.45647823904469931, 8.997362320892142051 ) ) ;
#14219=CARTESIAN_POINT ( 'NONE',  ( -1.996894868142000012, -77.31962480082998468, 10.85801781015000067 ) ) ;
#14221=CARTESIAN_POINT ( 'NONE',  ( -5.159044788988000008, -77.47084909945098730, -8.219183903844999861 ) ) ;
#14225=CARTESIAN_POINT ( 'NONE',  ( 0.000000000000000000, -81.89999999962999766, 0.000000000000000000 ) ) ;
#14226=CARTESIAN_POINT ( 'NONE',  ( -9.408410525920000822, -79.47180445808699290, -5.582976599613999724 ) ) ;
#14241=CARTESIAN_POINT ( 'NONE',  ( -8.751877897654001259, -78.60919638534799958, -3.466385404677000182 ) ) ;
#14250=CARTESIAN_POINT ( 'NONE',  ( -9.871730464199000465, -79.77354899574598335, 4.797141237513000256 ) ) ;
#14252=EDGE_CURVE ( 'NONE', #30580, #7174, #4128, .T. ) ;
#14263=DIRECTION ( 'NONE',  ( 0.000000000000000000, -1.000000000000000000, 0.000000000000000000 ) ) ;
#14279=DIRECTION ( 'NONE',  ( -1.000000000000000000, 0.000000000000000000, 0.000000000000000000 ) ) ;
#14281=CONICAL_SURFACE ( 'NONE', #23684, 1.099999997149000430, 0.7853981633972997312 ) ;
#14286=CARTESIAN_POINT ( 'NONE',  ( 2.287265073136303783, -78.24504505375756480, -8.963578713372259088 ) ) ;
#14295=CARTESIAN_POINT ( 'NONE',  ( 6.983565664416999219, -78.39846965846798810, -6.737990796766999857 ) ) ;
#14317=CARTESIAN_POINT ( 'NONE',  ( 8.467134758521000393, -79.12048981539898307, 4.837118142732999893 ) ) ;
#14322=CARTESIAN_POINT ( 'NONE',  ( -11.00000000000000000, -78.69999999999998863, 0.000000000000000000 ) ) ;
#14326=CARTESIAN_POINT ( 'NONE',  ( -5.756396345943000092, -77.16116605027188768, 9.567080340993001641 ) ) ;
#14343=CARTESIAN_POINT ( 'NONE',  ( 0.000000000000000000, -81.99999999999998579, 0.000000000000000000 ) ) ;
#14347=VERTEX_POINT ( 'NONE', #48135 ) ;
#14356=CARTESIAN_POINT ( 'NONE',  ( -8.082019532840464038, -79.14197076906785355, -4.658078629671525306 ) ) ;
#14357=CARTESIAN_POINT ( 'NONE',  ( -0.5548702034695790486, -77.97035308862197667, -9.688443984839716805 ) ) ;
#14366=CARTESIAN_POINT ( 'NONE',  ( 8.412275655993779466, -78.81594285012758405, -3.858088829829057431 ) ) ;
#14370=CARTESIAN_POINT ( 'NONE',  ( -9.210028442906166291, -80.14621276956458473, -6.014467946005654042 ) ) ;
#14397=CARTESIAN_POINT ( 'NONE',  ( 9.168564808419466416, -78.33948019894700110, -1.229073866473058718 ) ) ;
#14403=CARTESIAN_POINT ( 'NONE',  ( 9.711109801449000045, -79.03601937949099465, 1.878356537329999965 ) ) ;
#14404=DIRECTION ( 'NONE',  ( 1.000000000000000000, 0.000000000000000000, 0.000000000000000000 ) ) ;
#14408=CARTESIAN_POINT ( 'NONE',  ( 9.499693205731109202, -80.00008708754018016, -1.997583897032410100E-06 ) ) ;
#14415=CARTESIAN_POINT ( 'NONE',  ( 10.74143315901999962, -78.16829362456198282, -1.466515226187000032 ) ) ;
#14417=EDGE_LOOP ( 'NONE', ( #56960, #18388, #44000, #51757 ) ) ;
#14419=AXIS2_PLACEMENT_3D ( 'NONE', #53368, #13510, #44228 ) ;
#14424=CARTESIAN_POINT ( 'NONE',  ( 9.647254834573999460, -80.12796490456099718, -1.526580663425000095 ) ) ;
#14448=CARTESIAN_POINT ( 'NONE',  ( -10.74684349920000059, -80.03966949086598959, 2.363312785431999963 ) ) ;
#14463=CARTESIAN_POINT ( 'NONE',  ( 9.062046460520999602, -77.42945172698098588, -3.260755114102000363 ) ) ;
#14473=CARTESIAN_POINT ( 'NONE',  ( 1.439896632895302675, -79.23541666666665151, -11.00000000000000355 ) ) ;
#14474=CARTESIAN_POINT ( 'NONE',  ( 0.000000000000000000, -81.19999999999998863, -8.000000000000000000 ) ) ;
#14479=EDGE_CURVE ( 'NONE', #6792, #33386, #23866, .T. ) ;
#14489=CARTESIAN_POINT ( 'NONE',  ( 5.684557159767942736, -79.82291666666664298, 7.396918292183182864 ) ) ;
#14490=CARTESIAN_POINT ( 'NONE',  ( 1.684399200443891909, -78.31284097919404985, 10.84576505037703953 ) ) ;
#14501=AXIS2_PLACEMENT_3D ( 'NONE', #49421, #26089, #8971 ) ;
#14509=CARTESIAN_POINT ( 'NONE',  ( 10.36935812844000004, -78.07876026662599145, -2.835297515976000327 ) ) ;
#14511=CARTESIAN_POINT ( 'NONE',  ( 9.247895922801244950, -77.35175846627117835, 0.2043318676645352883 ) ) ;
#14512=CARTESIAN_POINT ( 'NONE',  ( 9.391860901740999523, -77.22419567483399305, 5.803232400709999794 ) ) ;
#14514=CARTESIAN_POINT ( 'NONE',  ( -9.139898499914998808, -77.36662839264398883, 2.826942883852999966 ) ) ;
#14519=CARTESIAN_POINT ( 'NONE',  ( 3.292343003156000147, -79.07851149742998587, -10.43303857396000112 ) ) ;
#14536=DIRECTION ( 'NONE',  ( 0.000000000000000000, -1.000000000000000000, 0.000000000000000000 ) ) ;
#14539=VECTOR ( 'NONE', #4487, 1000.000000000000000 ) ;
#14543=CARTESIAN_POINT ( 'NONE',  ( -0.6514878906251000412, -79.68927193274799947, 10.95625855609000077 ) ) ;
#14544=B_SPLINE_CURVE_WITH_KNOTS ( 'NONE', 3,
 ( #52791, #9087, #35338, #27073, #26484, #48375, #26206, #7913, #8788, #34765, #21775, #13502, #58383, #17645, #35045, #53363, #26779, #48659 ),
 .UNSPECIFIED., .F., .F.,
 ( 4, 2, 2, 2, 2, 2, 2, 2, 4 ),
 ( 0.000000000000000000, 0.1250000000000000278, 0.2500000000000000555, 0.3750000000000001110, 0.5000000000000001110, 0.6250000000000001110, 0.7500000000000002220, 0.8750000000000002220, 1.000000000000000000 ),
 .UNSPECIFIED. ) ;
#14564=DIRECTION ( 'NONE',  ( 1.000000000000000000, 0.000000000000000000, 0.000000000000000000 ) ) ;
#14567=FACE_OUTER_BOUND ( 'NONE', #8657, .T. ) ;
#14579=CARTESIAN_POINT ( 'NONE',  ( 5.968579026041624047, -78.28091924325941875, -7.066778786571805249 ) ) ;
#14584=CARTESIAN_POINT ( 'NONE',  ( -8.777663923591063622, -77.57446822344188320, 2.920505049390259344 ) ) ;
#14589=CARTESIAN_POINT ( 'NONE',  ( 7.658860137760000519, -78.57246790065498487, 5.959242465009999989 ) ) ;
#14611=AXIS2_PLACEMENT_3D ( 'NONE', #6645, #15504, #50367 ) ;
#14613=CARTESIAN_POINT ( 'NONE',  ( -1.494867482892000110, -79.44193905623698981, -9.636143388403000998 ) ) ;
#14618=AXIS2_PLACEMENT_3D ( 'NONE', #4265, #41152, #45006 ) ;
#14620=CARTESIAN_POINT ( 'NONE',  ( 11.02299141721000098, -77.92552186078398790, -0.5079658554739000520 ) ) ;
#14623=CARTESIAN_POINT ( 'NONE',  ( 2.781615572646999990, -78.16968490469898256, -8.992986673707997980 ) ) ;
#14625=CARTESIAN_POINT ( 'NONE',  ( -3.399186938124999724, -80.19999999999998863, -10.46162167925000119 ) ) ;
#14645=CARTESIAN_POINT ( 'NONE',  ( 0.000000000000000000, -81.99999999999998579, 7.000000000000000000 ) ) ;
#14649=CARTESIAN_POINT ( 'NONE',  ( -9.446590193405137725, -78.36828669642795830, -2.221657378611725964 ) ) ;
#14656=CARTESIAN_POINT ( 'NONE',  ( 8.129070811701460286, -78.81050004387087426, -4.417681596447804893 ) ) ;
#14660=CARTESIAN_POINT ( 'NONE',  ( -10.20656157772921446, -80.13085429318095976, -4.103012457657285950 ) ) ;
#14670=LINE ( 'NONE', #35941, #33587 ) ;
#14676=CARTESIAN_POINT ( 'NONE',  ( 10.75026368982902625, -77.20550397114976704, 0.6886793354171069081 ) ) ;
#14678=DIRECTION ( 'NONE',  ( 1.000000000000000000, 0.000000000000000000, 0.000000000000000000 ) ) ;
#14679=CARTESIAN_POINT ( 'NONE',  ( -10.65673661723999999, -78.83077053430758951, 2.626400817186000047 ) ) ;
#14689=CARTESIAN_POINT ( 'NONE',  ( -9.088317367618000020, -78.86622446787298202, 3.186800494491000002 ) ) ;
#14690=DIRECTION ( 'NONE',  ( -1.000000000000000000, 0.000000000000000000, 0.000000000000000000 ) ) ;
#14694=CIRCLE ( 'NONE', #56312, 4.100000000000000533 ) ;
#14703=DIRECTION ( 'NONE',  ( 0.7071067811864980568, 0.7071067811865969777, -8.992977225616968835E-09 ) ) ;
#14706=CARTESIAN_POINT ( 'NONE',  ( 11.10788134493000179, -77.25391046760299218, 1.523724958095000082 ) ) ;
#14711=CARTESIAN_POINT ( 'NONE',  ( -2.217000330786000450, -79.28367578985398723, 9.512392227823999846 ) ) ;
#14723=CARTESIAN_POINT ( 'NONE',  ( 9.365691051289999791, -76.94004530392098218, 2.708750943512000298 ) ) ;
#14735=AXIS2_PLACEMENT_3D ( 'NONE', #31297, #46089, #54642 ) ;
#14736=CARTESIAN_POINT ( 'NONE',  ( 0.000000000000000000, -76.19999999999998863, 0.000000000000000000 ) ) ;
#14742=FACE_OUTER_BOUND ( 'NONE', #25037, .T. ) ;
#14747=CARTESIAN_POINT ( 'NONE',  ( 6.193386186315999353, -78.02635213868897779, 7.375308638433999420 ) ) ;
#14751=ORIENTED_EDGE ( 'NONE', *, *, #15451, .F. ) ;
#14758=CARTESIAN_POINT ( 'NONE',  ( -4.277738290159001089, -79.08359478844498369, -10.10766895494000117 ) ) ;
#14759=B_SPLINE_CURVE_WITH_KNOTS ( 'NONE', 3,
 ( #44385, #43826, #21940, #39950, #57966, #39385, #57390, #54430, #18120, #36115 ),
 .UNSPECIFIED., .F., .F.,
 ( 4, 2, 2, 2, 4 ),
 ( 0.000000000000000000, 0.2500000000000000555, 0.5000000000000001110, 0.7500000000000000000, 1.000000000000000000 ),
 .UNSPECIFIED. ) ;
#14778=CARTESIAN_POINT ( 'NONE',  ( 3.915560572087711577, -79.29607338083805246, 10.25359469989230732 ) ) ;
#14795=ORIENTED_EDGE ( 'NONE', *, *, #14042, .F. ) ;
#14799=CARTESIAN_POINT ( 'NONE',  ( 7.016739011427143957, -77.40660838192772530, 6.033546689316169775 ) ) ;
#14808=CARTESIAN_POINT ( 'NONE',  ( 10.90877671396000004, -78.68521853677198408, 0.8284967960653000230 ) ) ;
#14821=CARTESIAN_POINT ( 'NONE',  ( -4.341134711875000107, -78.66604404360498393, -8.352589043283000336 ) ) ;
#14833=CARTESIAN_POINT ( 'NONE',  ( 9.694840914897000062, -79.52071780675198909, -5.145296513660000848 ) ) ;
#14844=CARTESIAN_POINT ( 'NONE',  ( 11.26616169758000119, -77.92955615878399556, 0.05236123134324999900 ) ) ;
#14849=CARTESIAN_POINT ( 'NONE',  ( 9.250000000000000000, -79.74999999999998579, 1.907449677260999760E-14 ) ) ;
#14853=ORIENTED_EDGE ( 'NONE', *, *, #20617, .T. ) ;
#14861=ORIENTED_EDGE ( 'NONE', *, *, #46354, .T. ) ;
#14867=CARTESIAN_POINT ( 'NONE',  ( 1.828541268174307399, -78.24096508442137576, -9.067390816575571222 ) ) ;
#14870=EDGE_LOOP ( 'NONE', ( #2823, #50238, #2868, #20315, #52917, #47495, #44338, #55280, #26821, #45832, #4990 ) ) ;
#14874=CARTESIAN_POINT ( 'NONE',  ( 10.18773063539611812, -78.17416963246105865, -3.499611392789568676 ) ) ;
#14877=CARTESIAN_POINT ( 'NONE',  ( -2.572125540837000290, -78.37350109675199406, -9.357076443458000270 ) ) ;
#14884=FACE_OUTER_BOUND ( 'NONE', #23005, .T. ) ;
#14893=CARTESIAN_POINT ( 'NONE',  ( 7.094389250268374525, -80.00000000000000000, -6.397685483451420296 ) ) ;
#14905=AXIS2_PLACEMENT_3D ( 'NONE', #58261, #40840, #13374 ) ;
#14908=CARTESIAN_POINT ( 'NONE',  ( 10.88908634000999953, -77.47532284559098059, -2.468401097160000113 ) ) ;
#14912=CARTESIAN_POINT ( 'NONE',  ( -3.430696936678000242, -78.42549936685999512, 8.765929102848000198 ) ) ;
#14947=CARTESIAN_POINT ( 'NONE',  ( 4.746041175454999816, -77.41566667364776322, -8.464384343845999581 ) ) ;
#14949=CARTESIAN_POINT ( 'NONE',  ( 8.393801617969296913, -79.55998208041128805, -4.599114686830800380 ) ) ;
#14950=EDGE_CURVE ( 'NONE', #56949, #10301, #32774, .T. ) ;
#14952=CARTESIAN_POINT ( 'NONE',  ( -7.828848276711099174, -78.64487340676903671, -4.926425388625121471 ) ) ;
#14956=CARTESIAN_POINT ( 'NONE',  ( -4.797609507281214825, -80.18923283849920836, -9.904543496687123749 ) ) ;
#14968=CARTESIAN_POINT ( 'NONE',  ( -5.683881862889148984, -79.67335042278446622, -7.396142196161008542 ) ) ;
#14974=CARTESIAN_POINT ( 'NONE',  ( 5.620651130188175415, -77.28197757598998408, 9.267943761422831273 ) ) ;
#14980=CARTESIAN_POINT ( 'NONE',  ( 7.546403568604966416, -78.30109726589176944, -5.349046595936441939 ) ) ;
#14985=CARTESIAN_POINT ( 'NONE',  ( -2.191084135724000070, -77.72224322018799114, 9.489933931099999498 ) ) ;
#14998=CARTESIAN_POINT ( 'NONE',  ( -4.543693065121372499, -77.58445504582732610, -8.146396484383414460 ) ) ;
#15000=ORIENTED_EDGE ( 'NONE', *, *, #30539, .T. ) ;
#15006=VECTOR ( 'NONE', #38114, 1000.000000000000114 ) ;
#15011=CARTESIAN_POINT ( 'NONE',  ( 9.202039358297998461, -80.16043756281898425, 2.360608321670000453 ) ) ;
#15023=CARTESIAN_POINT ( 'NONE',  ( 9.451694958653000356, -76.99163136579679190, 2.733625046654999835 ) ) ;
#15028=FACE_OUTER_BOUND ( 'NONE', #43954, .T. ) ;
#15043=CARTESIAN_POINT ( 'NONE',  ( -9.434983556464704435, -77.21406646732883416, -0.1995201537112713253 ) ) ;
#15048=CARTESIAN_POINT ( 'NONE',  ( 0.8552902072924000176, -78.33901425910798366, -9.592793577801000282 ) ) ;
#15050=CARTESIAN_POINT ( 'NONE',  ( 9.468749999988999022, -76.98125000001098783, 2.084568677130999610E-09 ) ) ;
#15057=CARTESIAN_POINT ( 'NONE',  ( 9.632126701410999914, -79.28024126877399169, 5.261763182588000021 ) ) ;
#15058=CARTESIAN_POINT ( 'NONE',  ( -10.93918996500858043, -80.09187350056868127, 1.167787996473995671 ) ) ;
#15059=CARTESIAN_POINT ( 'NONE',  ( 5.578188741145999607, -79.40460703100998785, 7.763689502541000209 ) ) ;
#15062=EDGE_LOOP ( 'NONE', ( #19054, #38112, #47488 ) ) ;
#15074=CARTESIAN_POINT ( 'NONE',  ( 8.867210690492070668, -78.64994923118607062, -6.468415063504793672 ) ) ;
#15095=CARTESIAN_POINT ( 'NONE',  ( 7.337322956731747503, -77.40219940825448930, 5.633178353381969927 ) ) ;
#15102=CARTESIAN_POINT ( 'NONE',  ( -10.86532694299999946, -79.50758784453798000, -2.005633084294999868 ) ) ;
#15109=CARTESIAN_POINT ( 'NONE',  ( -10.59387557900170940, -77.20000000000000284, 2.870323072861859615 ) ) ;
#15129=CARTESIAN_POINT ( 'NONE',  ( -10.44304457033000055, -78.34495714178498815, 3.377400876517000050 ) ) ;
#15130=FACE_OUTER_BOUND ( 'NONE', #13635, .T. ) ;
#15137=AXIS2_PLACEMENT_3D ( 'NONE', #1088, #24075, #18207 ) ;
#15161=FACE_OUTER_BOUND ( 'NONE', #44178, .T. ) ;
#15165=CARTESIAN_POINT ( 'NONE',  ( 3.632230827930608807, -78.25714950312151075, -8.507066908565283470 ) ) ;
#15169=ORIENTED_EDGE ( 'NONE', *, *, #24516, .F. ) ;
#15176=CARTESIAN_POINT ( 'NONE',  ( 7.405962610586999340, -77.46393856462499627, -6.270759699041999369 ) ) ;
#15177=CARTESIAN_POINT ( 'NONE',  ( 0.000000000000000000, -75.19999999999998863, 0.000000000000000000 ) ) ;
#15180=B_SPLINE_SURFACE_WITH_KNOTS ( 'NONE', 3, 3, ( 
 ( #4011, #44761, #22016, #58038, #17598, #4310, #22311, #40327, #53919, #13453, #23481, #45944, #19067, #28483, #10206, #23197, #33199, #41788, #50080, #19356, #46825, #18773, #6056, #41492, #54502, #37349, #55364, #51246, #46534, #24066, #1078, #37055, #10796, #28778, #14620 ),
 ( #55071, #32612, #41202, #6352, #14326, #15207, #32906, #50661, #42084, #1653, #19643, #32323, #27897, #28185, #24368, #14908, #5764, #36476, #37642, #55658, #46239, #23772, #42379, #18483, #792, #14041, #32035, #1359, #9625, #50949, #27613, #36764, #45653, #5194, #54783 ),
 ( #50368, #10499, #9917, #5476, #19942, #52398, #34652, #29074, #47981, #39095, #6938, #2806, #20800, #11669, #34362, #37931, #11952, #47119, #52680, #57103, #38806, #56825, #16671, #16380, #56247, #29930, #6646, #38518, #48269, #7519, #12235, #7226, #11382, #33786, #51537 ),
 ( #30224, #55956, #21092, #7805, #15505, #25806, #43249, #3097, #25516, #1948, #33500, #20520, #11093, #24656, #42666, #2235, #43533, #20233, #38227, #15797, #51828, #47696, #29358, #42961, #47406, #24941, #2517, #56533, #16093, #34074, #52110, #29643, #25229, #57397, #10072 ) ),
 .UNSPECIFIED., .F., .F., .F.,
 ( 4, 4 ),
 ( 4, 1, 1, 1, 1, 1, 1, 1, 1, 1, 1, 1, 1, 1, 1, 1, 1, 1, 1, 1, 1, 1, 1, 1, 1, 1, 1, 1, 1, 1, 1, 1, 4 ),
 ( -0.1387574078320999993, 1.138757407831999968 ),
 ( 0.4815154597993999697, 0.4980358005410999711, 0.5145561412828000281, 0.5310764820244999740, 0.5475968227662000309, 0.5641171635078000568, 0.5806375042495000027, 0.5971578449912000597, 0.6136781857329000056, 0.6301985264746000626, 0.6467188672163000085, 0.6632392079580000654, 0.6797595486996000913, 0.6962798894413000372, 0.7128002301829999832, 0.7293205709246999291, 0.7458409116664000971, 0.7623612524081000430, 0.7788815931497999889, 0.7954019338913999038, 0.8119222746331000717, 0.8284426153748000177, 0.8449629561165000746, 0.8614832968581999095, 0.8780036375998999665, 0.8945239783415001034, 0.9110443190832000493, 0.9275646598248999952, 0.9440850005665999412, 0.9606053413082999981, 0.9771256820500000551, 0.9936460227917000010, 1.010166363533000045 ),
 .UNSPECIFIED. ) ;
#15198=CARTESIAN_POINT ( 'NONE',  ( -9.250000000000000000, -78.99999999999998579, 0.000000000000000000 ) ) ;
#15201=CARTESIAN_POINT ( 'NONE',  ( -6.529936244858999927, -79.82726403785699176, 7.094943507923000325 ) ) ;
#15207=CARTESIAN_POINT ( 'NONE',  ( -8.749953746289000023, -77.18972575893728560, 6.935671482060999260 ) ) ;
#15211=CARTESIAN_POINT ( 'NONE',  ( 9.412698430168999764, -77.77175129689300093, 0.1109178415546999974 ) ) ;
#15229=ORIENTED_EDGE ( 'NONE', *, *, #32581, .F. ) ;
#15230=ORIENTED_EDGE ( 'NONE', *, *, #46254, .F. ) ;
#15234=ORIENTED_EDGE ( 'NONE', *, *, #11201, .F. ) ;
#15241=CARTESIAN_POINT ( 'NONE',  ( -5.685171361304339754, -79.17317559803932170, -7.397381645113899395 ) ) ;
#15245=CARTESIAN_POINT ( 'NONE',  ( 1.882180247600000245, -78.60946749706478442, 9.519879562373999349 ) ) ;
#15252=CARTESIAN_POINT ( 'NONE',  ( -4.009976957963860222, -78.68938149694008644, -8.341196569951419448 ) ) ;
#15257=CARTESIAN_POINT ( 'NONE',  ( -7.623780002575291093, -80.16446064207195832, -7.929242475467390250 ) ) ;
#15266=CARTESIAN_POINT ( 'NONE',  ( 1.199999995295999877, -81.00000000470399186, -6.999999972240000368 ) ) ;
#15267=CARTESIAN_POINT ( 'NONE',  ( -8.954424297038181990, -79.62125597785718867, -2.398079499860812369 ) ) ;
#15272=CARTESIAN_POINT ( 'NONE',  ( -3.664701384210835577, -77.85298049213145077, 10.19847459208089724 ) ) ;
#15274=B_SPLINE_CURVE_WITH_KNOTS ( 'NONE', 3,
 ( #19443, #47493, #6145, #20601, #19734, #11466, #55752, #37435, #56041, #55155, #24155, #14998, #28275, #24451, #29438, #32994, #51040, #10587 ),
 .UNSPECIFIED., .F., .F.,
 ( 4, 2, 2, 2, 2, 2, 2, 2, 4 ),
 ( 0.000000000000000000, 0.1250000000000000000, 0.2500000000000000000, 0.3750000000000000000, 0.5000000000000000000, 0.6250000000000000000, 0.7500000000000000000, 0.8750000000000000000, 1.000000000000000000 ),
 .UNSPECIFIED. ) ;
#15275=CARTESIAN_POINT ( 'NONE',  ( 7.218984044805001332, -79.16787878630005082, 8.267423174273998754 ) ) ;
#15280=CARTESIAN_POINT ( 'NONE',  ( 9.250000000000000000, -78.34999999999999432, 0.000000000000000000 ) ) ;
#15284=CARTESIAN_POINT ( 'NONE',  ( 5.053427186728000287, -78.72410532222798452, 8.198541555267000902 ) ) ;
#15287=CARTESIAN_POINT ( 'NONE',  ( 5.519612068167639052, -80.24166666702031137, -9.574916337700171809 ) ) ;
#15296=CARTESIAN_POINT ( 'NONE',  ( -7.558619072263999428, -78.87198591599799613, -8.058856703501000140 ) ) ;
#15298=CARTESIAN_POINT ( 'NONE',  ( 4.046534287111000161, -79.83266315943599523, -10.82105705926999839 ) ) ;
#15301=CARTESIAN_POINT ( 'NONE',  ( 9.338174682402000215, -77.82187845315299057, -6.595492338295000145 ) ) ;
#15310=CARTESIAN_POINT ( 'NONE',  ( 9.226480760116999136, -79.12131249856399506, -2.263195259622999611 ) ) ;
#15323=CARTESIAN_POINT ( 'NONE',  ( -9.641544011188999619, -77.26545691997898757, 0.6359099666973999643 ) ) ;
#15341=CARTESIAN_POINT ( 'NONE',  ( 5.450064804415999831, -77.22001278094698762, 7.901637168149001411 ) ) ;
#15347=CARTESIAN_POINT ( 'NONE',  ( 3.260206397764000119, -78.11865170860198759, 9.177731198418999981 ) ) ;
#15350=CARTESIAN_POINT ( 'NONE',  ( 0.000000000000000000, -77.04999999999999716, 0.000000000000000000 ) ) ;
#15358=CARTESIAN_POINT ( 'NONE',  ( -3.548303639235999896, -79.58925716643398118, -10.38621961377000069 ) ) ;
#15360=CARTESIAN_POINT ( 'NONE',  ( -4.085185354070000940, -80.05359608450199005, 8.504900574379000489 ) ) ;
#15377=CARTESIAN_POINT ( 'NONE',  ( -7.022618521819972592, -79.38035044383605054, 8.435084348146190791 ) ) ;
#15394=VERTEX_POINT ( 'NONE', #25898 ) ;
#15395=CARTESIAN_POINT ( 'NONE',  ( 7.430943141216144632, -77.40086315431187813, 5.508475347222059781 ) ) ;
#15396=CARTESIAN_POINT ( 'NONE',  ( 6.574300740938999077, -77.66621510448898391, -8.869200617850999890 ) ) ;
#15398=UNCERTAINTY_MEASURE_WITH_UNIT (LENGTH_MEASURE( 1.000000000000000082E-05 ), #35539, 'distance_accuracy_value', 'NONE');
#15405=CARTESIAN_POINT ( 'NONE',  ( 10.81514082164000001, -79.22666430121098813, -2.260668630147000258 ) ) ;
#15411=CARTESIAN_POINT ( 'NONE',  ( -10.17815165094191165, -77.19999999999998863, 4.038522141417139721 ) ) ;
#15419=CARTESIAN_POINT ( 'NONE',  ( -4.724527880064000485, -78.55937680961498870, 8.267358256580001452 ) ) ;
#15430=CARTESIAN_POINT ( 'NONE',  ( -10.65673661723999999, -78.79031659410199495, 2.626400817186000047 ) ) ;
#15444=LINE ( 'NONE', #33438, #39562 ) ;
#15451=EDGE_CURVE ( 'NONE', #27560, #29877, #49640, .T. ) ;
#15458=ORIENTED_EDGE ( 'NONE', *, *, #22500, .F. ) ;
#15459=ORIENTED_EDGE ( 'NONE', *, *, #31708, .F. ) ;
#15468=CARTESIAN_POINT ( 'NONE',  ( 5.148067466022420824, -78.27213350022245208, -7.684922334373290198 ) ) ;
#15470=ORIENTED_EDGE ( 'NONE', *, *, #54006, .F. ) ;
#15475=DIRECTION ( 'NONE',  ( -0.7071067811865474617, 0.7071067811865474617, -2.341635337278152801E-09 ) ) ;
#15476=CARTESIAN_POINT ( 'NONE',  ( -8.073459667400001649, -78.31665343849398653, -5.384232384047000330 ) ) ;
#15486=CARTESIAN_POINT ( 'NONE',  ( -7.283709231223095770, -80.36666666667369441, -8.098811904880690804 ) ) ;
#15495=CARTESIAN_POINT ( 'NONE',  ( 6.760013919724077169, -78.37708333333331723, -8.796335266379971429 ) ) ;
#15499=CARTESIAN_POINT ( 'NONE',  ( 9.210329749041999747, -79.12592023966598731, -2.015277344078000077 ) ) ;
#15504=DIRECTION ( 'NONE',  ( 0.000000000000000000, -1.000000000000000000, 0.000000000000000000 ) ) ;
#15505=CARTESIAN_POINT ( 'NONE',  ( -5.644242139785000667, -77.28891753183799551, 9.380681032049000834 ) ) ;
#15535=ORIENTED_EDGE ( 'NONE', *, *, #58090, .T. ) ;
#15540=CARTESIAN_POINT ( 'NONE',  ( 5.927986824875999261, -77.92729559796964622, -7.683077610609999830 ) ) ;
#15546=CARTESIAN_POINT ( 'NONE',  ( -7.233763587253225325, -78.65360029633727379, -5.764933821213369392 ) ) ;
#15552=CARTESIAN_POINT ( 'NONE',  ( -5.669906390347031255, -80.18205586309346700, -9.426039327529041500 ) ) ;
#15563=AXIS2_PLACEMENT_3D ( 'NONE', #20368, #20084, #24211 ) ;
#15567=CARTESIAN_POINT ( 'NONE',  ( 9.332554555131792995, -78.15887491149307209, -5.380831548737815773 ) ) ;
#15569=CARTESIAN_POINT ( 'NONE',  ( -6.920341278396000106, -79.42070997529405929, -8.518972542050999408 ) ) ;
#15575=CARTESIAN_POINT ( 'NONE',  ( 9.086775583825666303, -78.33514619779819554, -1.734270726548393871 ) ) ;
#15579=CARTESIAN_POINT ( 'NONE',  ( 6.263319273733999992, -78.14860065712299786, 7.458587492396000052 ) ) ;
#15588=CARTESIAN_POINT ( 'NONE',  ( 6.762881825298999949, -78.98435533332899183, -8.737352176957999816 ) ) ;
#15595=CARTESIAN_POINT ( 'NONE',  ( -6.211037838955999923, -77.19823840584228947, -9.120711488545000023 ) ) ;
#15602=CARTESIAN_POINT ( 'NONE',  ( 6.728605944993000243, -79.81563540107202925, -7.080011783993000130 ) ) ;
#15606=ORIENTED_EDGE ( 'NONE', *, *, #49457, .T. ) ;
#15614=CARTESIAN_POINT ( 'NONE',  ( -8.796335266379978535, -79.65208333333333712, -6.760013919724068288 ) ) ;
#15628=CARTESIAN_POINT ( 'NONE',  ( 5.511604622365999795, -77.15613704016388397, 7.990859100417000427 ) ) ;
#15632=AXIS2_PLACEMENT_3D ( 'NONE', #45706, #32962, #23248 ) ;
#15634=CARTESIAN_POINT ( 'NONE',  ( -9.704555048820999730, -77.77756575905399927, -0.8254132364208000006 ) ) ;
#15636=CARTESIAN_POINT ( 'NONE',  ( -4.716969252534931378, -77.08541666667790082, 8.182319320987406996 ) ) ;
#15638=CARTESIAN_POINT ( 'NONE',  ( 0.000000000000000000, -74.64999999999999147, 0.000000000000000000 ) ) ;
#15645=CARTESIAN_POINT ( 'NONE',  ( -10.96988615177242110, -80.09454209194464624, 0.8125309799759529161 ) ) ;
#15646=CARTESIAN_POINT ( 'NONE',  ( -6.632355475618000540, -79.14317342320499904, -6.884978231758999812 ) ) ;
#15683=CARTESIAN_POINT ( 'NONE',  ( 7.410718339131154409, -77.40115380615291940, 5.535753629427827782 ) ) ;
#15684=CARTESIAN_POINT ( 'NONE',  ( 10.65102452230999930, -77.76164423048498975, 2.905137941168000282 ) ) ;
#15693=CARTESIAN_POINT ( 'NONE',  ( -10.53745838584999994, -79.91191800929898648, 2.317267403318000074 ) ) ;
#15707=CARTESIAN_POINT ( 'NONE',  ( -8.431119552239000114, -78.10459554355099954, 4.425675013809000191 ) ) ;
#15718=CARTESIAN_POINT ( 'NONE',  ( 7.218984044805000444, -79.18772777176498323, 8.267423174273998754 ) ) ;
#15723=CARTESIAN_POINT ( 'NONE',  ( 6.000000002940000243, -81.20000000293998710, -1.734976712879000142E-08 ) ) ;
#15726=DIRECTION ( 'NONE',  ( 0.000000000000000000, 1.000000000000000000, 0.000000000000000000 ) ) ;
#15727=CARTESIAN_POINT ( 'NONE',  ( -9.250000000000000000, -78.01041666666667140, -1.210822168571064728 ) ) ;
#15729=CARTESIAN_POINT ( 'NONE',  ( -0.6687410688010000381, -79.55891271007898524, 11.24641019779000040 ) ) ;
#15742=CARTESIAN_POINT ( 'NONE',  ( -7.000000000000000000, -81.99999999999998579, 0.000000000000000000 ) ) ;
#15745=CARTESIAN_POINT ( 'NONE',  ( 4.926127088035904045, -79.91815483164202760, -8.184945656613731302 ) ) ;
#15753=CARTESIAN_POINT ( 'NONE',  ( -1.664588014272184502, -78.21069673449349580, -9.099086625984378784 ) ) ;
#15757=CARTESIAN_POINT ( 'NONE',  ( -8.852603344437753208, -77.57660330915794589, 2.682567943804467614 ) ) ;
#15760=CARTESIAN_POINT ( 'NONE',  ( -6.473047519705999342, -78.20295812197798568, 7.229824698717000508 ) ) ;
#15777=CARTESIAN_POINT ( 'NONE',  ( -9.010394027838918518, -79.57955026341325322, 2.421758550787145303 ) ) ;
#15778=CARTESIAN_POINT ( 'NONE',  ( -4.999715220074000044, -80.01690199409698323, -9.878567298617999981 ) ) ;
#15780=ADVANCED_FACE ( 'NONE', ( #48688 ), #43969, .F. ) ;
#15785=CARTESIAN_POINT ( 'NONE',  ( -9.250000000000000000, -78.49999999999998579, 0.000000000000000000 ) ) ;
#15790=CARTESIAN_POINT ( 'NONE',  ( 9.563799579366000003, -79.07178538496899023, -0.8978884989661999327 ) ) ;
#15792=CARTESIAN_POINT ( 'NONE',  ( 9.494736565810956819, -79.10440807414381936, 0.5477041750795209607 ) ) ;
#15795=CARTESIAN_POINT ( 'NONE',  ( -2.600000000000000089, -78.49999999999998579, 0.000000000000000000 ) ) ;
#15797=CARTESIAN_POINT ( 'NONE',  ( 3.837643902511000071, -77.71731316181897853, 10.25315621143999856 ) ) ;
#15804=CARTESIAN_POINT ( 'NONE',  ( 6.760013919724039866, -77.42291666666667993, 8.796335266379998075 ) ) ;
#15813=ORIENTED_EDGE ( 'NONE', *, *, #24591, .T. ) ;
#15827=EDGE_LOOP ( 'NONE', ( #51197, #1680 ) ) ;
#15838=CARTESIAN_POINT ( 'NONE',  ( 10.71369944335147117, -78.47083333333331723, 2.879226727952105769 ) ) ;
#15840=CARTESIAN_POINT ( 'NONE',  ( -6.523492958078782600, -78.66275140589766579, -6.557889900168049735 ) ) ;
#15860=CARTESIAN_POINT ( 'NONE',  ( 9.469096744587201187, -77.74081920503226684, 5.269811678343041095 ) ) ;
#15863=CARTESIAN_POINT ( 'NONE',  ( 10.74341457190999982, -79.08360172330206694, -2.245675826504000216 ) ) ;
#15865=EDGE_LOOP ( 'NONE', ( #48780, #46911, #12828 ) ) ;
#15870=CARTESIAN_POINT ( 'NONE',  ( 1.265244864176999995, -77.69381939105899448, 9.657062241701000360 ) ) ;
#15881=CARTESIAN_POINT ( 'NONE',  ( 0.9151062594318000176, -78.67533943566898813, 11.01092521911999889 ) ) ;
#15884=FACE_OUTER_BOUND ( 'NONE', #3916, .T. ) ;
#15887=CARTESIAN_POINT ( 'NONE',  ( 11.29729853867000067, -77.85856316181899217, -1.753017772781999772 ) ) ;
#15889=EDGE_LOOP ( 'NONE', ( #55967, #1211, #44309, #32344, #9425, #24086, #18581 ) ) ;
#15892=CARTESIAN_POINT ( 'NONE',  ( -2.116314338179000387, -80.23777995843001065, -9.535298106756000536 ) ) ;
#15896=VERTEX_POINT ( 'NONE', #43685 ) ;
#15904=CARTESIAN_POINT ( 'NONE',  ( -6.146221368751000114, -77.09692023966638885, 7.568187592052000312 ) ) ;
#15914=DIRECTION ( 'NONE',  ( 0.000000000000000000, 0.000000000000000000, -1.000000000000000000 ) ) ;
#15920=CARTESIAN_POINT ( 'NONE',  ( -3.716474266315000108, -77.11277995979999389, -8.432660871143999870 ) ) ;
#15925=CARTESIAN_POINT ( 'NONE',  ( -8.711966356949998769, -77.23751300560297750, 3.874524904258000557 ) ) ;
#15928=CARTESIAN_POINT ( 'NONE',  ( -9.319010416924347950, -77.13098958334455801, 1.219003397386794862 ) ) ;
#15933=CARTESIAN_POINT ( 'NONE',  ( -9.488660192930483461, -79.25397600642003226, -0.4744913388225507900 ) ) ;
#15936=CARTESIAN_POINT ( 'NONE',  ( -10.30068234846894626, -80.07172511735936382, 3.869806167791196572 ) ) ;
#15937=CARTESIAN_POINT ( 'NONE',  ( -3.001687856302999613, -79.54317808830998615, 9.192644655792999941 ) ) ;
#15939=CARTESIAN_POINT ( 'NONE',  ( -6.760013919724058518, -78.67291666666667993, -8.796335266379987416 ) ) ;
#15959=VERTEX_POINT ( 'NONE', #14408 ) ;
#15961=CARTESIAN_POINT ( 'NONE',  ( -9.702392362153268834, -78.85149179162094413, -0.1934172642948918386 ) ) ;
#15973=CARTESIAN_POINT ( 'NONE',  ( 7.486916784802780889, -77.30012800153166097, -5.432092700114928618 ) ) ;
#15983=CARTESIAN_POINT ( 'NONE',  ( -9.312499999988999022, -77.13750000001088836, -2.050180145195999796E-09 ) ) ;
#15984=CARTESIAN_POINT ( 'NONE',  ( -9.152236916771000708, -78.94574075788399625, 6.189866966782000546 ) ) ;
#15992=CARTESIAN_POINT ( 'NONE',  ( -0.2501781407124171741, -77.20000000000001705, 10.80171731040410243 ) ) ;
#16001=CARTESIAN_POINT ( 'NONE',  ( 8.393017115181999444, -78.92888658829198789, 4.056188317180000169 ) ) ;
#16012=CARTESIAN_POINT ( 'NONE',  ( -7.508490145779999736, -78.93489658277098897, -8.005410190140000992 ) ) ;
#16018=ORIENTED_EDGE ( 'NONE', *, *, #47840, .F. ) ;
#16019=CYLINDRICAL_SURFACE ( 'NONE', #56914, 1.000000000000000000 ) ;
#16023=CARTESIAN_POINT ( 'NONE',  ( -9.688835989853998854, -79.22180445808699290, -5.749381838710999837 ) ) ;
#16026=DIRECTION ( 'NONE',  ( 0.000000000000000000, -1.000000000000000000, 0.000000000000000000 ) ) ;
#16031=AXIS2_PLACEMENT_3D ( 'NONE', #44055, #16327, #7170 ) ;
#16047=CARTESIAN_POINT ( 'NONE',  ( -1.966495496757295847, -78.20800177901919881, -9.040030525289719066 ) ) ;
#16048=CARTESIAN_POINT ( 'NONE',  ( 4.601194894417628412, -79.33389418958066130, 8.114662363814824531 ) ) ;
#16052=CARTESIAN_POINT ( 'NONE',  ( -6.677150611632656663, -77.53932992427476734, 6.401716840538735021 ) ) ;
#16055=CARTESIAN_POINT ( 'NONE',  ( 9.259046916275000427, -78.60434699719698415, 2.905298533503999803 ) ) ;
#16067=CARTESIAN_POINT ( 'NONE',  ( -10.69999999999999929, -77.19999999999998863, 0.000000000000000000 ) ) ;
#16075=CARTESIAN_POINT ( 'NONE',  ( 8.396295933391000332, -80.12268549011298546, -7.217020962015999963 ) ) ;
#16084=CARTESIAN_POINT ( 'NONE',  ( -5.076456076831999731, -80.03725306992998867, -8.069692061488998647 ) ) ;
#16093=CARTESIAN_POINT ( 'NONE',  ( -2.917097991912000143, -77.97435053980699138, -10.55202616546000094 ) ) ;
#16099=CARTESIAN_POINT ( 'NONE',  ( -9.555818165766000405, -77.27086163495798132, -0.1257991660602000017 ) ) ;
#16111=EDGE_LOOP ( 'NONE', ( #53501, #35913, #29719, #9805, #47510 ) ) ;
#16127=B_SPLINE_CURVE_WITH_KNOTS ( 'NONE', 3,
 ( #31611, #22478, #10080, #45222, #32775, #49652, #9199, #951, #40489, #50820, #36344, #54371, #14489, #22770, #50526, #18935, #27771, #5632 ),
 .UNSPECIFIED., .F., .F.,
 ( 4, 2, 2, 2, 2, 2, 2, 2, 4 ),
 ( 0.000000000000000000, 0.1250000000000000555, 0.2500000000000001110, 0.3750000000000001665, 0.5000000000000001110, 0.6250000000000001110, 0.7500000000000002220, 0.8750000000000001110, 1.000000000000000000 ),
 .UNSPECIFIED. ) ;
#16130=CARTESIAN_POINT ( 'NONE',  ( -9.674786689060324463, -79.84246777690499641, 0.8964806179170247136 ) ) ;
#16133=CARTESIAN_POINT ( 'NONE',  ( -5.884541003006559912, -78.67027905328879456, -7.138263159130112889 ) ) ;
#16137=CARTESIAN_POINT ( 'NONE',  ( -10.34820832961891490, -80.12787718711169305, -3.730169475059172957 ) ) ;
#16148=CARTESIAN_POINT ( 'NONE',  ( -5.500000000000000000, -80.99999999999998579, 0.000000000000000000 ) ) ;
#16150=CARTESIAN_POINT ( 'NONE',  ( 9.249483092228999226, -79.25084128437099196, 0.09778817195952001218 ) ) ;
#16153=CARTESIAN_POINT ( 'NONE',  ( -10.75519713130186261, -77.95494529858517296, -0.6025658906798456727 ) ) ;
#16160=DIRECTION ( 'NONE',  ( 0.7071067811865474617, -0.7071067811865474617, -3.205711300058212616E-10 ) ) ;
#16164=CARTESIAN_POINT ( 'NONE',  ( 3.223804565277000211, -78.24090022703498448, 9.075257246486000184 ) ) ;
#16169=DIRECTION ( 'NONE',  ( 0.000000000000000000, 0.000000000000000000, -1.000000000000000000 ) ) ;
#16173=CARTESIAN_POINT ( 'NONE',  ( 10.78711022396000097, -79.57429477431499265, 2.390846439793999689 ) ) ;
#16178=CARTESIAN_POINT ( 'NONE',  ( 10.22337536533999902, -78.27158863368499908, -4.865471675980000299 ) ) ;
#16185=CARTESIAN_POINT ( 'NONE',  ( -2.217000330786000450, -79.40352863330448940, 9.512392227823999846 ) ) ;
#16204=CARTESIAN_POINT ( 'NONE',  ( 9.250000000000000000, -77.74999999999998579, 0.000000000000000000 ) ) ;
#16212=CARTESIAN_POINT ( 'NONE',  ( 2.554064167922000195, -77.37387362948199154, 9.027803880580000495 ) ) ;
#16225=CARTESIAN_POINT ( 'NONE',  ( 8.195846875379992014, -79.04247058337611520, 4.844231267137363517 ) ) ;
#16226=CARTESIAN_POINT ( 'NONE',  ( 2.935661446561999899, -79.99999999999998579, -9.035036904803998681 ) ) ;
#16228=CIRCLE ( 'NONE', #20981, 9.549999999999998934 ) ;
#16230=CARTESIAN_POINT ( 'NONE',  ( -6.785595605124000507, -79.27092490477099318, -7.044055193142999549 ) ) ;
#16233=ORIENTED_EDGE ( 'NONE', *, *, #5924, .F. ) ;
#16241=VERTEX_POINT ( 'NONE', #55671 ) ;
#16246=AXIS2_PLACEMENT_3D ( 'NONE', #2600, #20597, #11458 ) ;
#16249=DIRECTION ( 'NONE',  ( -1.000000000000000000, 0.000000000000000000, 0.000000000000000000 ) ) ;
#16258=CARTESIAN_POINT ( 'NONE',  ( -10.71369944335148361, -77.67916666666667425, 2.879226727952040044 ) ) ;
#16265=CARTESIAN_POINT ( 'NONE',  ( 3.537828989635279697, -79.94386011961954353, 8.546646707163249701 ) ) ;
#16269=CARTESIAN_POINT ( 'NONE',  ( 9.550909342165001092, -79.32632342844499362, -5.975706243058000133 ) ) ;
#16270=CARTESIAN_POINT ( 'NONE',  ( 7.485279715301945913, -77.30010352984844246, -5.434349560424259096 ) ) ;
#16281=CARTESIAN_POINT ( 'NONE',  ( -6.966543547089000477, -79.56377255320299469, -8.575847751312000611 ) ) ;
#16293=DIRECTION ( 'NONE',  ( 0.000000000000000000, 0.7071067811866525998, -0.7071067811864425456 ) ) ;
#16305=CARTESIAN_POINT ( 'NONE',  ( -8.082524092276901939, -78.95833333333332860, 4.658475568430788805 ) ) ;
#16308=CARTESIAN_POINT ( 'NONE',  ( -9.871730464199000465, -79.83385192141699349, 4.797141237513000256 ) ) ;
#16309=CARTESIAN_POINT ( 'NONE',  ( 0.000000000000000000, -74.64999999999999147, 0.000000000000000000 ) ) ;
#16317=CARTESIAN_POINT ( 'NONE',  ( 0.000000000000000000, -75.19999999999998863, -4.100000000000000533 ) ) ;
#16318=CARTESIAN_POINT ( 'NONE',  ( 2.592785862636999727, -78.38672486022498731, -10.85214546196000107 ) ) ;
#16327=DIRECTION ( 'NONE',  ( 0.000000000000000000, -1.000000000000000000, 0.000000000000000000 ) ) ;
#16346=CARTESIAN_POINT ( 'NONE',  ( -3.357666854334504514, -77.50471486696052636, 8.619924559119072072 ) ) ;
#16347=FACE_OUTER_BOUND ( 'NONE', #804, .T. ) ;
#16348=CARTESIAN_POINT ( 'NONE',  ( 10.61050599188999932, -78.32876026662599145, -2.901234667509999809 ) ) ;
#16349=CARTESIAN_POINT ( 'NONE',  ( -2.572125540837000290, -78.43380402242298999, -9.357076443458000270 ) ) ;
#16353=CARTESIAN_POINT ( 'NONE',  ( 8.693423296916000353, -80.12538939878398025, -7.148151291522000683 ) ) ;
#16361=CARTESIAN_POINT ( 'NONE',  ( -7.397096502814789254, -78.54793235670427975, 5.684705351741184742 ) ) ;
#16363=CARTESIAN_POINT ( 'NONE',  ( 5.642647961229684483, -79.42304073986576896, 7.355092408208053989 ) ) ;
#16368=ORIENTED_EDGE ( 'NONE', *, *, #5835, .F. ) ;
#16373=CARTESIAN_POINT ( 'NONE',  ( -0.4810211636624999731, -79.27203353095599425, 9.630519408955999339 ) ) ;
#16378=CARTESIAN_POINT ( 'NONE',  ( 9.549999999999998934, -76.89999999999999147, 0.000000000000000000 ) ) ;
#16380=CARTESIAN_POINT ( 'NONE',  ( -9.737968063966999210, -77.76767625569698339, 5.236421613506999861 ) ) ;
#16385=CARTESIAN_POINT ( 'NONE',  ( -3.591972190522999764, -77.23543021507899198, 8.980252640667000463 ) ) ;
#16399=EDGE_LOOP ( 'NONE', ( #9946, #13165, #30601, #36834 ) ) ;
#16406=B_SPLINE_SURFACE_WITH_KNOTS ( 'NONE', 3, 3, ( 
 ( #26701, #14008, #49463, #3984, #45325, #27288, #763, #54472, #32005, #31420, #45029, #18741, #36734, #22581, #54750, #13715, #35559, #13419, #53585, #50047, #21986, #9009, #14295, #45621, #26409, #4876, #22280, #13123, #53888, #32289, #26994, #4283, #31118, #9593, #4581, #40297, #50335, #5162, #22872, #49158, #23162, #18453, #41170, #31710, #18165, #9299, #40595, #40882, #189, #8710, #36158, #44431, #39995, #58008, #17567, #44732, #54178, #58308, #17869, #49759, #474, #36443, #42635, #10179, #42349, #50918, #6320 ),
 ( #20201, #55625, #19033, #55332, #37026, #37901, #5446, #10467, #2202, #29043, #9885, #46795, #5735, #55040, #19325, #56212, #28453, #46208, #14589, #55925, #46501, #23742, #38193, #1916, #47084, #14877, #28157, #15476, #33467, #37317, #50629, #15760, #6025, #51504, #42048, #11062, #6613, #24624, #33755, #24337, #41756, #19910, #27865, #45912, #1331, #24035, #23451, #10766, #51214, #41463, #28744, #19610, #1049, #32580, #1620, #37610, #32874, #15176, #33169, #30185, #8054, #7770, #34040, #6902, #17195, #3060, #39633 ),
 ( #38482, #48507, #3622, #16922, #38771, #26049, #29325, #12480, #47666, #16632, #24911, #7192, #52932, #48234, #44075, #47372, #25194, #7482, #21628, #16055, #56788, #47951, #2483, #30481, #29611, #16349, #43212, #25480, #57641, #52077, #34329, #43500, #20487, #51794, #2771, #52364, #34901, #25773, #56500, #11347, #43797, #39352, #39057, #21056, #34618, #57072, #3344, #52645, #11636, #11916, #57359, #42928, #20770, #29894, #12200, #21340, #17489, #690, #35476, #13047, #12764, #9516, #53507, #9224, #17791, #31636, #13933 ),
 ( #22798, #26618, #22505, #27503, #31046, #31928, #49678, #53807, #40806, #4797, #36370, #49081, #44655, #40216, #45543, #13641, #4504, #35778, #13343, #22205, #31339, #40516, #23085, #399, #39918, #18377, #54396, #18087, #5089, #49382, #49973, #8633, #44354, #53216, #41098, #4208, #35184, #48793, #8339, #36079, #58227, #8930, #26336, #54099, #26918, #27209, #44949, #45248, #3908, #21909, #37242, #32219, #1544, #19247, #50843, #54963, #10691, #28670, #18672, #50551, #28083, #14221, #55547, #41680, #46723, #14514, #50260 ) ),
 .UNSPECIFIED., .F., .F., .F.,
 ( 4, 4 ),
 ( 4, 1, 1, 1, 1, 1, 1, 1, 1, 1, 1, 1, 1, 1, 1, 1, 1, 1, 1, 1, 1, 1, 1, 1, 1, 1, 1, 1, 1, 1, 1, 1, 1, 1, 1, 1, 1, 1, 1, 1, 1, 1, 1, 1, 1, 1, 1, 1, 1, 1, 1, 1, 1, 1, 1, 1, 1, 1, 1, 1, 1, 1, 1, 1, 4 ),
 ( -0.4045438850609999748, 1.404543885061000141 ),
 ( -0.02000000000000000042, -0.003749999999999999861, 0.01250000000000000069, 0.02875000000000000125, 0.04499999999999999833, 0.06124999999999999889, 0.07749999999999999944, 0.09375000000000000000, 0.1100000000000000006, 0.1262500000000000011, 0.1424999999999999878, 0.1587500000000000022, 0.1749999999999999889, 0.1912500000000000033, 0.2074999999999999900, 0.2237500000000000044, 0.2399999999999999911, 0.2562499999999999778, 0.2725000000000000200, 0.2887500000000000067, 0.3049999999999999933, 0.3212499999999999800, 0.3375000000000000222, 0.3537500000000000089, 0.3699999999999999956, 0.3862499999999999822, 0.4025000000000000244, 0.4187500000000000111, 0.4349999999999999978, 0.4512499999999999845, 0.4675000000000000266, 0.4837500000000000133, 0.5000000000000000000, 0.5162499999999999867, 0.5324999999999999734, 0.5487499999999999600, 0.5649999999999999467, 0.5812500000000000444, 0.5975000000000000311, 0.6137500000000000178, 0.6300000000000000044, 0.6462499999999999911, 0.6624999999999999778, 0.6787499999999999645, 0.6949999999999999512, 0.7112500000000000488, 0.7275000000000000355, 0.7437500000000000222, 0.7600000000000000089, 0.7762499999999999956, 0.7924999999999999822, 0.8087499999999999689, 0.8249999999999999556, 0.8412500000000000533, 0.8575000000000000400, 0.8737500000000000266, 0.8900000000000000133, 0.9062500000000000000, 0.9224999999999999867, 0.9387499999999999734, 0.9549999999999999600, 0.9712499999999999467, 0.9875000000000000444, 1.003749999999999920, 1.020000000000000018 ),
 .UNSPECIFIED. ) ;
#16421=CARTESIAN_POINT ( 'NONE',  ( -9.350444020985786864, -77.33083626513527520, 2.280479404982021840 ) ) ;
#16448=B_SPLINE_CURVE_WITH_KNOTS ( 'NONE', 3,
 ( #35419, #53449, #21855, #56734 ),
 .UNSPECIFIED., .F., .F.,
 ( 4, 4 ),
 ( 0.000000000000000000, 1.000000000000000000 ),
 .UNSPECIFIED. ) ;
#16452=CARTESIAN_POINT ( 'NONE',  ( 9.440269692223999698, -78.12720491051898364, -1.906441214165000009 ) ) ;
#16458=CARTESIAN_POINT ( 'NONE',  ( 7.986185577601829344, -78.89281710089944966, 4.706103088835384973 ) ) ;
#16461=CARTESIAN_POINT ( 'NONE',  ( 10.94849663375999960, -79.54620241998199504, -1.486040076422999956 ) ) ;
#16463=CARTESIAN_POINT ( 'NONE',  ( -8.715923958271998728, -80.31661853915498739, 7.063164134645999681 ) ) ;
#16466=ADVANCED_FACE ( 'NONE', ( #997 ), #36975, .T. ) ;
#16472=CARTESIAN_POINT ( 'NONE',  ( -5.726462542197000793, -80.20530730017200938, -7.912542777261000637 ) ) ;
#16488=CARTESIAN_POINT ( 'NONE',  ( 9.250000000000000000, -78.84999999999999432, 1.340711541092999922E-14 ) ) ;
#16491=CARTESIAN_POINT ( 'NONE',  ( 9.009247259181915268, -77.77083333333335702, 2.421167930323361972 ) ) ;
#16494=DIRECTION ( 'NONE',  ( 0.000000000000000000, -1.000000000000000000, 0.000000000000000000 ) ) ;
#16503=CARTESIAN_POINT ( 'NONE',  ( -8.623695280723000067, -78.23234702511798844, 4.526762133323999571 ) ) ;
#16513=CARTESIAN_POINT ( 'NONE',  ( -7.586433418133593065, -79.30182515582218628, -5.779326228052479308 ) ) ;
#16514=CARTESIAN_POINT ( 'NONE',  ( -5.793906668835271390, -79.99999999999998579, -7.373316236663074008 ) ) ;
#16518=CARTESIAN_POINT ( 'NONE',  ( -9.294849547870001061, -79.68174914560898969, 3.044469259936000149 ) ) ;
#16520=CARTESIAN_POINT ( 'NONE',  ( 8.796335266379994522, -78.79791666666666572, -6.760013919724047859 ) ) ;
#16523=CONICAL_SURFACE ( 'NONE', #51431, 9.400000000000000355, 0.7853981633972997312 ) ;
#16535=CARTESIAN_POINT ( 'NONE',  ( 8.193575559979001000, -79.00534903806799036, 5.316613930189999948 ) ) ;
#16550=CARTESIAN_POINT ( 'NONE',  ( 4.445228475228653942, -79.93551855130198192, 8.119495521249815440 ) ) ;
#16554=CARTESIAN_POINT ( 'NONE',  ( 11.16390912141999792, -79.86007816076597976, -1.515278025736000123 ) ) ;
#16555=CARTESIAN_POINT ( 'NONE',  ( 6.898510738327106928, -77.29199995586373007, -6.163577416694886679 ) ) ;
#16562=CARTESIAN_POINT ( 'NONE',  ( -11.00000000000000000, -78.59999999999999432, 0.000000000000000000 ) ) ;
#16564=FACE_OUTER_BOUND ( 'NONE', #54235, .T. ) ;
#16565=CARTESIAN_POINT ( 'NONE',  ( 3.980415848809999879, -79.40290945932498801, 10.42342982551999953 ) ) ;
#16566=ADVANCED_FACE ( 'NONE', ( #34852 ), #11159, .T. ) ;
#16579=CARTESIAN_POINT ( 'NONE',  ( -7.316919381717999826, -78.58780063874398536, 6.093690752987000359 ) ) ;
#16591=CARTESIAN_POINT ( 'NONE',  ( -10.69701368780000017, -79.86194427574999111, 1.066019776055000090 ) ) ;
#16602=CARTESIAN_POINT ( 'NONE',  ( -11.10294551207000069, -79.16561974942199242, 1.911422329490000127 ) ) ;
#16610=CIRCLE ( 'NONE', #46812, 10.69999999999999929 ) ;
#16619=EDGE_CURVE ( 'NONE', #41582, #44945, #25289, .T. ) ;
#16620=ORIENTED_EDGE ( 'NONE', *, *, #34464, .F. ) ;
#16624=CARTESIAN_POINT ( 'NONE',  ( 0.1144858057291637116, -78.22606344178616666, -9.249342975308575632 ) ) ;
#16628=CARTESIAN_POINT ( 'NONE',  ( -2.333868897602956238, -77.49531809838757113, 8.954045959266851540 ) ) ;
#16629=CARTESIAN_POINT ( 'NONE',  ( -8.283402485401001769, -77.86702283146098580, -7.298588567667000149 ) ) ;
#16632=CARTESIAN_POINT ( 'NONE',  ( -7.203390125892000562, -78.88858528848699336, -6.502451851937000704 ) ) ;
#16637=CARTESIAN_POINT ( 'NONE',  ( -11.11771682179999843, -80.41771755615498307, 1.751409206030000165 ) ) ;
#16647=CARTESIAN_POINT ( 'NONE',  ( -9.009538955111615621, -78.57917760043629585, 2.421331503275422126 ) ) ;
#16667=CARTESIAN_POINT ( 'NONE',  ( 0.000000000000000000, -80.74999999986198418, -5.249999999862000166 ) ) ;
#16669=CARTESIAN_POINT ( 'NONE',  ( -10.71369944335147117, -77.22083333333334565, -2.879226727952084453 ) ) ;
#16671=CARTESIAN_POINT ( 'NONE',  ( -7.278304428485000699, -77.73911654703098861, 8.323125493531998487 ) ) ;
#16676=CARTESIAN_POINT ( 'NONE',  ( 5.212684961665999595, -76.87984006102360013, -8.147089634514999901 ) ) ;
#16703=CIRCLE ( 'NONE', #28949, 9.549999999999998934 ) ;
#16710=CARTESIAN_POINT ( 'NONE',  ( 5.491641493159680643, -77.17685792801958655, 7.961916067739349678 ) ) ;
#16712=CARTESIAN_POINT ( 'NONE',  ( -9.217496754025233940, -78.60672666432962785, -0.7743134236860684805 ) ) ;
#16715=CARTESIAN_POINT ( 'NONE',  ( -10.44884804545204382, -80.12557790367317523, -3.439072401377349486 ) ) ;
#16733=ORIENTED_EDGE ( 'NONE', *, *, #35921, .F. ) ;
#16739=CARTESIAN_POINT ( 'NONE',  ( -8.985695946343000173, -78.93010020865598619, 3.150816496261000133 ) ) ;
#16746=CARTESIAN_POINT ( 'NONE',  ( -2.879226727952095555, -78.80416666666667425, -10.71369944335146940 ) ) ;
#16750=ORIENTED_EDGE ( 'NONE', *, *, #4135, .T. ) ;
#16751=CARTESIAN_POINT ( 'NONE',  ( 8.999546809828999017, -78.07436279057898787, -5.951127176402999375 ) ) ;
#16753=CARTESIAN_POINT ( 'NONE',  ( -4.004180130848999930, -80.27485737381698527, 10.47959906926000073 ) ) ;
#16764=CARTESIAN_POINT ( 'NONE',  ( 5.496668217546000434, -80.42257811839652959, -8.073860231047000013 ) ) ;
#16776=CARTESIAN_POINT ( 'NONE',  ( 8.994028603496278862, -78.83108882679107410, -2.182395696014679309 ) ) ;
#16779=CARTESIAN_POINT ( 'NONE',  ( -8.082524092276901939, -77.95833333333330017, 4.658475568430788805 ) ) ;
#16782=CARTESIAN_POINT ( 'NONE',  ( 10.71369944335146762, -77.87083333333333712, 2.879226727952103548 ) ) ;
#16785=LINE ( 'NONE', #34186, #870 ) ;
#16802=CARTESIAN_POINT ( 'NONE',  ( -3.176479431003079057, -79.34794335332261994, -8.982299932693875277 ) ) ;
#16803=CARTESIAN_POINT ( 'NONE',  ( -7.966098808101403250, -80.00000000000000000, -4.899225432969430472 ) ) ;
#16806=CARTESIAN_POINT ( 'NONE',  ( -3.070249596178999951, -79.67092956987599450, 9.402614426748000298 ) ) ;
#16808=CARTESIAN_POINT ( 'NONE',  ( 8.082524092276891281, -79.20833333333335702, -4.658475568430806568 ) ) ;
#16810=CARTESIAN_POINT ( 'NONE',  ( 4.799999999999999822, -74.99999999999998579, 0.000000000000000000 ) ) ;
#16819=CARTESIAN_POINT ( 'NONE',  ( 10.58237688094999918, -77.70362064813399172, 3.355437010509000118 ) ) ;
#16820=DIRECTION ( 'NONE',  ( 1.000000000000000000, 0.000000000000000000, 0.000000000000000000 ) ) ;
#16826=CARTESIAN_POINT ( 'NONE',  ( -0.6514213267380000172, -79.58985688671099012, 9.745581310452999801 ) ) ;
#16833=CARTESIAN_POINT ( 'NONE',  ( 9.499157866768639380, -79.10080562451891240, 0.1004279358040388037 ) ) ;
#16834=CARTESIAN_POINT ( 'NONE',  ( 9.250000000000000000, -78.24999999999998579, -1.152201742116999973E-14 ) ) ;
#16842=CARTESIAN_POINT ( 'NONE',  ( 9.045200488146255324, -80.24963439586137781, 6.447942591652251032 ) ) ;
#16844=CARTESIAN_POINT ( 'NONE',  ( -8.859962374443000499, -78.56782986146299663, 6.959166695099000322 ) ) ;
#16845=CARTESIAN_POINT ( 'NONE',  ( 6.702743137996565181, -77.28954671824730838, -6.375165872689311897 ) ) ;
#16855=CARTESIAN_POINT ( 'NONE',  ( 6.184832724006000149, -78.72869295534098910, -9.286519468188998871 ) ) ;
#16861=CARTESIAN_POINT ( 'NONE',  ( -8.890092043222985296, -77.19999999999998863, 6.337337654403193632 ) ) ;
#16870=CARTESIAN_POINT ( 'NONE',  ( 7.267019124662000173, -77.33715215706898505, -6.153113788875000267 ) ) ;
#16882=CARTESIAN_POINT ( 'NONE',  ( 10.97550047727999889, -78.18052123279399268, 0.05101033830554000531 ) ) ;
#16883=CARTESIAN_POINT ( 'NONE',  ( -5.440921534716935071, -80.39791666666549474, 9.438387255472232340 ) ) ;
#16887=VERTEX_POINT ( 'NONE', #13932 ) ;
#16889=CARTESIAN_POINT ( 'NONE',  ( 9.164177083796486656, -77.26245504524652574, 1.449973650478227682 ) ) ;
#16890=CARTESIAN_POINT ( 'NONE',  ( 1.439896632895284911, -78.06458333333334565, 11.00000000000000355 ) ) ;
#16891=CARTESIAN_POINT ( 'NONE',  ( -11.14855507251999889, -78.24626308856198875, -0.4486863643567999826 ) ) ;
#16896=VERTEX_POINT ( 'NONE', #9808 ) ;
#16902=EDGE_LOOP ( 'NONE', ( #4188, #16733, #7687, #53531, #1818, #23390 ) ) ;
#16918=CARTESIAN_POINT ( 'NONE',  ( -4.267465266896234510, -77.51327689984762515, 8.206740657596899524 ) ) ;
#16919=CARTESIAN_POINT ( 'NONE',  ( -6.065106684382000068, -77.23082865815298703, 9.224892016835999797 ) ) ;
#16922=CARTESIAN_POINT ( 'NONE',  ( 9.367484565636001292, -79.05912826326098752, -2.533990228858999938 ) ) ;
#16924=CARTESIAN_POINT ( 'NONE',  ( -9.249310757543522499, -77.50112171249398330, -0.1303866578235779172 ) ) ;
#16926=CARTESIAN_POINT ( 'NONE',  ( 3.942135768300999654, -80.02332530777499642, -10.54187931140000067 ) ) ;
#16942=ORIENTED_EDGE ( 'NONE', *, *, #44317, .T. ) ;
#16960=CARTESIAN_POINT ( 'NONE',  ( 9.100722152916000951, -76.93205879495988597, -3.274758550341999808 ) ) ;
#16975=ORIENTED_EDGE ( 'NONE', *, *, #49961, .T. ) ;
#16984=CARTESIAN_POINT ( 'NONE',  ( 3.321932689531000182, -77.19999999999998863, 10.22385755016999909 ) ) ;
#16993=CARTESIAN_POINT ( 'NONE',  ( -9.309367086190000862, -77.13855160546319212, -0.1968645694141999969 ) ) ;
#17023=CARTESIAN_POINT ( 'NONE',  ( -1.944889849486000077, -77.50188066968198086, -9.432423272878001086 ) ) ;
#17033=CARTESIAN_POINT ( 'NONE',  ( -7.484260875330000395, -78.93586165678098610, -7.979577400219000083 ) ) ;
#17035=CARTESIAN_POINT ( 'NONE',  ( -7.298083752484999742, -79.81301656954198620, -8.811591453050999334 ) ) ;
#17042=CARTESIAN_POINT ( 'NONE',  ( 9.226480760116999136, -79.48087102891551581, -2.263195259622999611 ) ) ;
#17047=ORIENTED_EDGE ( 'NONE', *, *, #45440, .F. ) ;
#17056=CARTESIAN_POINT ( 'NONE',  ( 8.547140491457867029, -78.81892730245148471, -3.536545408174746274 ) ) ;
#17057=CARTESIAN_POINT ( 'NONE',  ( 0.000000000000000000, -81.90000000002299885, -10.59999999997999787 ) ) ;
#17071=EDGE_CURVE ( 'NONE', #4408, #37493, #57361, .T. ) ;
#17078=ORIENTED_EDGE ( 'NONE', *, *, #38805, .T. ) ;
#17082=CARTESIAN_POINT ( 'NONE',  ( -9.271561418023951617, -79.22981385905036689, 2.410639693388377580 ) ) ;
#17086=CARTESIAN_POINT ( 'NONE',  ( 5.707072418784999712, -79.53235851257699096, 7.943069029044000473 ) ) ;
#17089=VERTEX_POINT ( 'NONE', #44082 ) ;
#17090=DIRECTION ( 'NONE',  ( 0.000000000000000000, 1.000000000000000000, 0.000000000000000000 ) ) ;
#17103=CARTESIAN_POINT ( 'NONE',  ( 1.841371367509999857, -79.90994107844498728, -9.592189096167999196 ) ) ;
#17107=ADVANCED_FACE ( 'NONE', ( #8938 ), #7425, .F. ) ;
#17110=EDGE_CURVE ( 'NONE', #5115, #50169, #31181, .T. ) ;
#17120=CARTESIAN_POINT ( 'NONE',  ( 0.7916942038310399443, -79.96867701788805505, 9.217398666066213053 ) ) ;
#17121=LINE ( 'NONE', #54023, #51097 ) ;
#17124=CARTESIAN_POINT ( 'NONE',  ( 7.410162453131999172, -79.43869284577598933, 8.486367113423000319 ) ) ;
#17125=CARTESIAN_POINT ( 'NONE',  ( 4.220602197252363297, -77.26272508603567246, -8.230959913729840594 ) ) ;
#17136=CARTESIAN_POINT ( 'NONE',  ( 4.711402524194999941, -78.89724708133699949, 10.11406376844000121 ) ) ;
#17141=CARTESIAN_POINT ( 'NONE',  ( -9.096312194199068557, -77.19999999999997442, 6.047136293109013572 ) ) ;
#17143=CARTESIAN_POINT ( 'NONE',  ( 9.250000000000000000, -79.24999999999998579, 0.000000000000000000 ) ) ;
#17149=CARTESIAN_POINT ( 'NONE',  ( -7.148970245326999873, -78.76537169604299038, -6.453327391511999522 ) ) ;
#17159=CARTESIAN_POINT ( 'NONE',  ( -0.6514878906251000412, -79.80987778408999134, 10.95625855609000077 ) ) ;
#17160=CARTESIAN_POINT ( 'NONE',  ( 10.90625000000000000, -80.29374999999798490, -5.301077343649000152E-10 ) ) ;
#17169=CARTESIAN_POINT ( 'NONE',  ( 7.439427647571000612, -79.42614197053399039, -8.315438409070999626 ) ) ;
#17171=LINE ( 'NONE', #3596, #22797 ) ;
#17179=ORIENTED_EDGE ( 'NONE', *, *, #51244, .T. ) ;
#17182=CARTESIAN_POINT ( 'NONE',  ( 0.000000000000000000, -77.49999999999998579, 0.000000000000000000 ) ) ;
#17187=CARTESIAN_POINT ( 'NONE',  ( -6.486048890515720089, -78.16333030288288342, -6.594899609276845709 ) ) ;
#17190=VERTEX_POINT ( 'NONE', #41981 ) ;
#17192=CARTESIAN_POINT ( 'NONE',  ( -5.470294744961789135, -77.52538948961748133, 7.459090554855953847 ) ) ;
#17195=CARTESIAN_POINT ( 'NONE',  ( -9.685922776715001348, -77.26497176072199125, 0.5943755449006998814 ) ) ;
#17200=CARTESIAN_POINT ( 'NONE',  ( -8.744140569415000286, -80.37595639081598620, 7.086030162020000134 ) ) ;
#17201=VECTOR ( 'NONE', #34648, 1000.000000000000000 ) ;
#17217=CARTESIAN_POINT ( 'NONE',  ( -1.439896632895359962, -80.08541666668128300, 10.99999999999999645 ) ) ;
#17238=CARTESIAN_POINT ( 'NONE',  ( 2.632967082928999947, -77.12290855547149704, 9.306700570505000769 ) ) ;
#17246=CIRCLE ( 'NONE', #55915, 10.50000000000000000 ) ;
#17262=LINE ( 'NONE', #12829, #21234 ) ;
#17266=CARTESIAN_POINT ( 'NONE',  ( 0.000000000000000000, -75.10000000032299283, 0.000000000000000000 ) ) ;
#17275=VECTOR ( 'NONE', #15475, 1000.000000000000114 ) ;
#17300=ORIENTED_EDGE ( 'NONE', *, *, #29220, .F. ) ;
#17302=CARTESIAN_POINT ( 'NONE',  ( -9.469606800734000629, -79.65752053325199711, 5.597012331546999953 ) ) ;
#17306=CARTESIAN_POINT ( 'NONE',  ( 9.511010664898998712, -78.15562873964798030, 1.514558053418999961 ) ) ;
#17312=CARTESIAN_POINT ( 'NONE',  ( -6.760013919724074505, -78.77291666666668846, -8.796335266379974982 ) ) ;
#17316=CARTESIAN_POINT ( 'NONE',  ( 9.295311691678000088, -79.60238712864799027, 5.972861453165999812 ) ) ;
#17319=CARTESIAN_POINT ( 'NONE',  ( 7.094168877687000219, -80.19133504314000049, 8.690698855587999816 ) ) ;
#17326=CARTESIAN_POINT ( 'NONE',  ( -7.479908383216000267, -79.80559761149552855, -6.281056869080000382 ) ) ;
#17327=VERTEX_POINT ( 'NONE', #56147 ) ;
#17337=AXIS2_PLACEMENT_3D ( 'NONE', #33383, #51710, #20969 ) ;
#17340=DIRECTION ( 'NONE',  ( -1.000000000000000000, 0.000000000000000000, 0.000000000000000000 ) ) ;
#17345=CARTESIAN_POINT ( 'NONE',  ( -4.099999999699000419, -75.20000000030088927, 8.298667500436000154E-10 ) ) ;
#17347=DIRECTION ( 'NONE',  ( -1.000000000000000000, 0.000000000000000000, 0.000000000000000000 ) ) ;
#17358=CARTESIAN_POINT ( 'NONE',  ( 0.000000000000000000, -77.04999999999999716, 0.000000000000000000 ) ) ;
#17375=CARTESIAN_POINT ( 'NONE',  ( 3.221881332551000288, -80.05522572818799176, 9.234895928605999060 ) ) ;
#17393=CARTESIAN_POINT ( 'NONE',  ( -5.726462542197000793, -79.90529868759999488, -7.912542777261000637 ) ) ;
#17397=CARTESIAN_POINT ( 'NONE',  ( 0.000000000000000000, -74.64999999999999147, 0.000000000000000000 ) ) ;
#17401=CARTESIAN_POINT ( 'NONE',  ( 9.051220798599112882, -77.62926713907424414, 3.499889976320043061 ) ) ;
#17410=CARTESIAN_POINT ( 'NONE',  ( 3.532511455861872651, -79.94390816463113936, 8.548848039690394529 ) ) ;
#17412=ORIENTED_EDGE ( 'NONE', *, *, #11201, .T. ) ;
#17413=CARTESIAN_POINT ( 'NONE',  ( -10.93895610016999953, -79.10158459378298801, 2.695955081989000135 ) ) ;
#17420=CARTESIAN_POINT ( 'NONE',  ( 10.73159385090000129, -78.78487766400598957, -3.053603293876000269 ) ) ;
#17430=VECTOR ( 'NONE', #23879, 1000.000000000000000 ) ;
#17448=CARTESIAN_POINT ( 'NONE',  ( 7.218984044805000444, -79.24803069743599337, 8.267423174273998754 ) ) ;
#17452=CARTESIAN_POINT ( 'NONE',  ( -11.00000000000000000, -79.69999999999998863, 0.000000000000000000 ) ) ;
#17458=CARTESIAN_POINT ( 'NONE',  ( -0.6622892437428999912, -79.62278845086298418, 11.13790800686000004 ) ) ;
#17475=CARTESIAN_POINT ( 'NONE',  ( 9.376176103360082337, -79.51460875094232961, 1.742736205308521802 ) ) ;
#17476=ORIENTED_EDGE ( 'NONE', *, *, #57467, .T. ) ;
#17478=EDGE_CURVE ( 'NONE', #44945, #10899, #841, .T. ) ;
#17481=CARTESIAN_POINT ( 'NONE',  ( -3.533434062681735544, -78.19395196561279704, -8.548428288705636646 ) ) ;
#17486=CARTESIAN_POINT ( 'NONE',  ( 2.036425055830775488, -77.45743550615227946, 9.023012778983279247 ) ) ;
#17487=CARTESIAN_POINT ( 'NONE',  ( -9.050627908549000011, -77.35806749281498185, -6.322205650057999726 ) ) ;
#17489=CARTESIAN_POINT ( 'NONE',  ( 9.131029190779001325, -77.55266531942498887, -3.285576857342999979 ) ) ;
#17493=CARTESIAN_POINT ( 'NONE',  ( -1.635010352784000087, -80.54300105216999839, -10.62493487727000030 ) ) ;
#17518=CARTESIAN_POINT ( 'NONE',  ( 9.106330615755000579, -79.18979598044998625, -1.992521687893000104 ) ) ;
#17521=CARTESIAN_POINT ( 'NONE',  ( 0.000000000000000000, -81.99999999999998579, -10.50000000000000000 ) ) ;
#17528=CARTESIAN_POINT ( 'NONE',  ( 9.498848458907630743, -79.06748417780224258, 0.1004247326035953569 ) ) ;
#17536=DIRECTION ( 'NONE',  ( 0.000000000000000000, -1.000000000000000000, 0.000000000000000000 ) ) ;
#17539=ORIENTED_EDGE ( 'NONE', *, *, #14042, .T. ) ;
#17541=EDGE_CURVE ( 'NONE', #44945, #29444, #14670, .T. ) ;
#17552=EDGE_CURVE ( 'NONE', #55944, #21753, #53766, .T. ) ;
#17557=ORIENTED_EDGE ( 'NONE', *, *, #19466, .F. ) ;
#17558=CARTESIAN_POINT ( 'NONE',  ( -7.062685404271999090, -77.78023905895217638, 8.485436034813998774 ) ) ;
#17560=B_SPLINE_CURVE_WITH_KNOTS ( 'NONE', 3,
 ( #12451, #44620, #44043, #9190, #27175, #26309, #31306, #30446, #45213, #13016, #21598, #3593, #4761, #26017, #3880, #21879, #39603, #44913 ),
 .UNSPECIFIED., .F., .F.,
 ( 4, 2, 2, 2, 2, 2, 2, 2, 4 ),
 ( 0.000000000000000000, 0.1250000000000000000, 0.2500000000000000000, 0.3750000000000000000, 0.5000000000000000000, 0.6250000000000000000, 0.7500000000000000000, 0.8750000000000000000, 1.000000000000000000 ),
 .UNSPECIFIED. ) ;
#17565=VECTOR ( 'NONE', #44821, 1000.000000000000000 ) ;
#17567=CARTESIAN_POINT ( 'NONE',  ( 9.051070938631999852, -77.48890712634099032, 3.499832029064999794 ) ) ;
#17572=AXIS2_PLACEMENT_3D ( 'NONE', #9551, #18699, #45282 ) ;
#17578=CARTESIAN_POINT ( 'NONE',  ( -8.674899888355607658, -78.62823151048618797, -3.212842792980429518 ) ) ;
#17589=CARTESIAN_POINT ( 'NONE',  ( 9.250000000000000000, -78.84999999999999432, 1.340711541092999922E-14 ) ) ;
#17590=CARTESIAN_POINT ( 'NONE',  ( -10.71369944335147117, -79.22083333333333144, -2.879226727952084453 ) ) ;
#17598=CARTESIAN_POINT ( 'NONE',  ( -5.812473449021000604, -77.09729030948868456, 9.660279995464000180 ) ) ;
#17601=CARTESIAN_POINT ( 'NONE',  ( -3.833926501619000060, -78.04896150565798507, -8.716156481626001096 ) ) ;
#17606=ORIENTED_EDGE ( 'NONE', *, *, #38010, .T. ) ;
#17609=CARTESIAN_POINT ( 'NONE',  ( -2.460449926407452192, -78.99659071566932766, 8.997086085319750737 ) ) ;
#17614=CARTESIAN_POINT ( 'NONE',  ( -6.999846649096999940, -79.30106226310599027, 8.407732347380999727 ) ) ;
#17616=CARTESIAN_POINT ( 'NONE',  ( -3.516941471767000227, -80.40586707127998523, -10.40795029645000014 ) ) ;
#17617=CIRCLE ( 'NONE', #38345, 1.199999999999999956 ) ;
#17645=CARTESIAN_POINT ( 'NONE',  ( -5.239266479141337030, -80.01428708882451701, 9.745699944792930225 ) ) ;
#17655=CARTESIAN_POINT ( 'NONE',  ( 10.90625000000000000, -80.29374999999798490, -5.301077343649000152E-10 ) ) ;
#17673=CARTESIAN_POINT ( 'NONE',  ( 2.268344470944000157, -78.97289170186299145, -9.471763527590001175 ) ) ;
#17694=CARTESIAN_POINT ( 'NONE',  ( -7.545891804452000251, -79.71510512889798861, 6.201630566990999682 ) ) ;
#17697=ORIENTED_EDGE ( 'NONE', *, *, #7679, .F. ) ;
#17699=FACE_OUTER_BOUND ( 'NONE', #27112, .T. ) ;
#17706=CARTESIAN_POINT ( 'NONE',  ( 7.256259382531156099, -77.65769096820322659, 6.443642414277258368 ) ) ;
#17714=CARTESIAN_POINT ( 'NONE',  ( 7.021204365543900039, -79.90651252694955531, 6.021971066871157241 ) ) ;
#17717=VERTEX_POINT ( 'NONE', #18110 ) ;
#17718=CARTESIAN_POINT ( 'NONE',  ( -9.512698799462512511, -77.24565731317359507, 0.5183019084032332024 ) ) ;
#17730=CARTESIAN_POINT ( 'NONE',  ( 0.000000000000000000, -77.19999999999998863, 0.000000000000000000 ) ) ;
#17748=CARTESIAN_POINT ( 'NONE',  ( 9.028681611143001717, -78.19400356791099682, -5.970393136294000591 ) ) ;
#17760=CARTESIAN_POINT ( 'NONE',  ( -0.5280093414736000135, -78.86429488387997822, -11.14507989169999824 ) ) ;
#17767=CARTESIAN_POINT ( 'NONE',  ( -8.084233020759592492, -79.64022715548099995, 7.554717540679545706 ) ) ;
#17770=EDGE_LOOP ( 'NONE', ( #668, #37997, #41293, #26928 ) ) ;
#17774=CARTESIAN_POINT ( 'NONE',  ( -8.619769076539709474, -79.78588492011769517, -4.179965034922113354 ) ) ;
#17775=ORIENTED_EDGE ( 'NONE', *, *, #31865, .T. ) ;
#17787=CARTESIAN_POINT ( 'NONE',  ( 2.599724825704791797, -77.45250025653473358, 8.877253526477543843 ) ) ;
#17788=CARTESIAN_POINT ( 'NONE',  ( -3.203604947276999848, -77.76827721380398373, 10.56508708803000118 ) ) ;
#17791=CARTESIAN_POINT ( 'NONE',  ( -9.685922776715001348, -77.32527468639298718, 0.5943755449006998814 ) ) ;
#17821=CARTESIAN_POINT ( 'NONE',  ( 2.974672214138999848, -79.30668661348099135, 9.057689976529999853 ) ) ;
#17836=CARTESIAN_POINT ( 'NONE',  ( -3.591972190522999764, -77.29573314074899315, 8.980252640667000463 ) ) ;
#17845=CARTESIAN_POINT ( 'NONE',  ( 6.760013919724070064, -79.42291666666666572, 8.796335266379976758 ) ) ;
#17849=ORIENTED_EDGE ( 'NONE', *, *, #1288, .T. ) ;
#17851=ORIENTED_EDGE ( 'NONE', *, *, #1000, .F. ) ;
#17855=CARTESIAN_POINT ( 'NONE',  ( 11.10498291493000167, -80.08699962660007543, -1.830582403018000015 ) ) ;
#17861=CARTESIAN_POINT ( 'NONE',  ( 8.680753609988000719, -77.65300022429065052, 6.821192461343000168 ) ) ;
#17866=DIRECTION ( 'NONE',  ( -0.7071067811865474617, -0.7071067811865474617, -3.010159793144197746E-10 ) ) ;
#17869=CARTESIAN_POINT ( 'NONE',  ( 4.746041175454999816, -77.37521180982498947, -8.464384343845999581 ) ) ;
#17870=CONICAL_SURFACE ( 'NONE', #47096, 4.199999999676998996, 0.7853981633972997312 ) ;
#17872=FACE_BOUND ( 'NONE', #38187, .T. ) ;
#17882=AXIS2_PLACEMENT_3D ( 'NONE', #44217, #21766, #17340 ) ;
#17883=ADVANCED_FACE ( 'NONE', ( #57004 ), #23227, .F. ) ;
#17903=CARTESIAN_POINT ( 'NONE',  ( 9.521438313890000060, -77.70787555610998254, 0.1121992162086000028 ) ) ;
#17908=ORIENTED_EDGE ( 'NONE', *, *, #41685, .T. ) ;
#17936=CARTESIAN_POINT ( 'NONE',  ( 6.559075508479975447, -78.78789540257247381, -6.522196071853445076 ) ) ;
#17938=LINE ( 'NONE', #17057, #35768 ) ;
#17957=CARTESIAN_POINT ( 'NONE',  ( 0.000000000000000000, -77.49999999999998579, 0.000000000000000000 ) ) ;
#17971=CARTESIAN_POINT ( 'NONE',  ( 9.697485508432000856, -79.08658701837899230, 0.9045115177663000106 ) ) ;
#17978=CYLINDRICAL_SURFACE ( 'NONE', #25058, 9.549999999999998934 ) ;
#17986=CARTESIAN_POINT ( 'NONE',  ( -10.82992633042000108, -77.44682768747698276, -2.440973915835000341 ) ) ;
#17992=CARTESIAN_POINT ( 'NONE',  ( 3.269429986698999979, -79.67799007979499493, 9.203886808668999109 ) ) ;
#18006=CARTESIAN_POINT ( 'NONE',  ( 7.032896718443679696, -79.90636255966268209, 6.008298471892056902 ) ) ;
#18007=CARTESIAN_POINT ( 'NONE',  ( -0.2823905925365536862, -80.07332856916835340, -11.10458707158487890 ) ) ;
#18010=CARTESIAN_POINT ( 'NONE',  ( -0.4674429229059374746, -77.22105961193567225, -9.250557976676333283 ) ) ;
#18017=CARTESIAN_POINT ( 'NONE',  ( -4.472180980751999435, -79.96475654597900018, 10.22208999787000039 ) ) ;
#18037=CARTESIAN_POINT ( 'NONE',  ( 7.396918292183153554, -78.80208333333332860, 5.684557159767984480 ) ) ;
#18039=FACE_OUTER_BOUND ( 'NONE', #40590, .T. ) ;
#18044=CARTESIAN_POINT ( 'NONE',  ( 8.318585563179999198, -78.29700886712998908, 7.159970128962999780 ) ) ;
#18052=CARTESIAN_POINT ( 'NONE',  ( 8.267707368506879817, -77.21246842999600801, -4.210867517961808026 ) ) ;
#18057=CARTESIAN_POINT ( 'NONE',  ( -8.689005542484000699, -78.25395412067899770, 6.824886543446999632 ) ) ;
#18070=CARTESIAN_POINT ( 'NONE',  ( -3.363908607861598288, -79.65371335578565493, 8.914120539577261582 ) ) ;
#18074=CARTESIAN_POINT ( 'NONE',  ( 9.250000000000001776, -79.73958333333332860, -1.210822168571047186 ) ) ;
#18080=VERTEX_POINT ( 'NONE', #34700 ) ;
#18081=CARTESIAN_POINT ( 'NONE',  ( -1.703864646944121430, -77.48977711739701135, 9.091877587378041525 ) ) ;
#18083=CARTESIAN_POINT ( 'NONE',  ( 10.07768261906999996, -78.14667722612898615, -4.508174471003999706 ) ) ;
#18087=CARTESIAN_POINT ( 'NONE',  ( -8.073459667400001649, -78.43725928983597839, -5.384232384047000330 ) ) ;
#18092=CARTESIAN_POINT ( 'NONE',  ( -10.93134324956000114, -78.43238734777798982, -0.4399444258272000030 ) ) ;
#18094=CARTESIAN_POINT ( 'NONE',  ( 1.210822168571075386, -78.63541666666665719, -9.249999999999996447 ) ) ;
#18106=CARTESIAN_POINT ( 'NONE',  ( 9.194664024258999646, -80.35622046769498183, 6.554488853579999663 ) ) ;
#18110=CARTESIAN_POINT ( 'NONE',  ( -11.00000000000000000, -77.59999999999999432, 0.000000000000000000 ) ) ;
#18120=CARTESIAN_POINT ( 'NONE',  ( 10.75000000000000000, -77.20000000000000284, 1.135012739489781763 ) ) ;
#18130=CARTESIAN_POINT ( 'NONE',  ( -2.880544446985999762, -76.93082093378328068, -9.112186890989001142 ) ) ;
#18133=CARTESIAN_POINT ( 'NONE',  ( 10.62542268813949242, -78.08596328497016259, -1.896582608316532692 ) ) ;
#18138=CARTESIAN_POINT ( 'NONE',  ( -6.760013919724082498, -79.52708333333333712, 8.796335266379969653 ) ) ;
#18165=CARTESIAN_POINT ( 'NONE',  ( -6.766389538252999714, -77.77314541763098532, -6.956053621355001049 ) ) ;
#18169=EDGE_CURVE ( 'NONE', #47434, #58355, #20849, .T. ) ;
#18186=AXIS2_PLACEMENT_3D ( 'NONE', #30982, #41038, #13874 ) ;
#18187=CARTESIAN_POINT ( 'NONE',  ( 8.796335266379992746, -79.39791666666667425, -6.760013919724047859 ) ) ;
#18190=CARTESIAN_POINT ( 'NONE',  ( -9.709808591512000930, -79.82183361358998752, 0.8997258012745000810 ) ) ;
#18202=CARTESIAN_POINT ( 'NONE',  ( 6.123453098898000491, -78.27635213868897779, 7.292029784470999587 ) ) ;
#18207=DIRECTION ( 'NONE',  ( 1.000000000000000000, 0.000000000000000000, 0.000000000000000000 ) ) ;
#18212=VERTEX_POINT ( 'NONE', #21713 ) ;
#18213=ORIENTED_EDGE ( 'NONE', *, *, #39432, .F. ) ;
#18216=DIRECTION ( 'NONE',  ( 0.000000000000000000, 1.000000000000000000, 0.000000000000000000 ) ) ;
#18219=AXIS2_PLACEMENT_3D ( 'NONE', #18323, #36315, #12428 ) ;
#18223=EDGE_CURVE ( 'NONE', #1524, #21041, #54335, .T. ) ;
#18230=CARTESIAN_POINT ( 'NONE',  ( 6.112347209136727244, -79.28239249943922573, -6.968733846918607533 ) ) ;
#18239=CARTESIAN_POINT ( 'NONE',  ( 7.359266617186424497, -78.79822258401679846, -5.604483073908840929 ) ) ;
#18241=CARTESIAN_POINT ( 'NONE',  ( -2.879226727952121756, -78.49583333333333712, 10.71369944335146407 ) ) ;
#18270=CARTESIAN_POINT ( 'NONE',  ( -2.581517684854000017, -78.43283894841299286, -9.391243908516001326 ) ) ;
#18278=FACE_OUTER_BOUND ( 'NONE', #56693, .T. ) ;
#18284=CARTESIAN_POINT ( 'NONE',  ( -10.89239325544999915, -77.47401871959498010, 2.657546225328000222 ) ) ;
#18286=ORIENTED_EDGE ( 'NONE', *, *, #55680, .F. ) ;
#18290=CARTESIAN_POINT ( 'NONE',  ( -9.699833017908000343, -79.32079083895699512, 1.146274062705999963 ) ) ;
#18291=ORIENTED_EDGE ( 'NONE', *, *, #7675, .T. ) ;
#18299=EDGE_CURVE ( 'NONE', #47367, #27909, #57266, .T. ) ;
#18301=CARTESIAN_POINT ( 'NONE',  ( -2.183112477083999803, -77.64305730667976491, 9.455407409464999802 ) ) ;
#18302=CARTESIAN_POINT ( 'NONE',  ( 8.240049981720177996, -79.88800312984227503, 4.202220852354948910 ) ) ;
#18305=CARTESIAN_POINT ( 'NONE',  ( 9.670530767802999250, -76.99862249932546376, -0.1674091926992999912 ) ) ;
#18306=CARTESIAN_POINT ( 'NONE',  ( -1.829463144348593806, -77.20923816470673273, -9.073295249180375777 ) ) ;
#18315=CARTESIAN_POINT ( 'NONE',  ( -10.75000000005474732, -80.44999999999997442, -1.125737367057300542 ) ) ;
#18323=CARTESIAN_POINT ( 'NONE',  ( 7.000000000000000000, -81.99999999999998579, 0.000000000000000000 ) ) ;
#18328=CARTESIAN_POINT ( 'NONE',  ( 9.189097042878000110, -78.48113340475299538, 2.883349701574000168 ) ) ;
#18336=CARTESIAN_POINT ( 'NONE',  ( -8.631379868284000167, -78.37716771312298647, 6.779623747090999686 ) ) ;
#18337=FACE_OUTER_BOUND ( 'NONE', #955, .T. ) ;
#18348=AXIS2_PLACEMENT_3D ( 'NONE', #44930, #22485, #13325 ) ;
#18350=CARTESIAN_POINT ( 'NONE',  ( -7.035077178968999867, -79.31377255320299469, -8.660212973301998574 ) ) ;
#18355=CARTESIAN_POINT ( 'NONE',  ( 1.748323643227930546, -79.56240695551150566, 10.92574688943146022 ) ) ;
#18361=ORIENTED_EDGE ( 'NONE', *, *, #35746, .F. ) ;
#18367=CARTESIAN_POINT ( 'NONE',  ( -5.253916984369498167, -78.17694262828045737, -7.614320282445113719 ) ) ;
#18371=DIRECTION ( 'NONE',  ( 0.000000000000000000, -1.000000000000000000, 1.147693051705999857E-13 ) ) ;
#18373=CARTESIAN_POINT ( 'NONE',  ( -0.1831506106021379421, -77.47674350841900548, 9.248349794432215276 ) ) ;
#18374=CARTESIAN_POINT ( 'NONE',  ( 10.07768261906999996, -78.08637430045799022, -4.508174471003999706 ) ) ;
#18377=CARTESIAN_POINT ( 'NONE',  ( -2.572125540837000290, -78.49410694809398592, -9.357076443458000270 ) ) ;
#18382=CARTESIAN_POINT ( 'NONE',  ( -4.263934386054000214, -79.02232678876399063, -10.07505235160000012 ) ) ;
#18383=AXIS2_PLACEMENT_3D ( 'NONE', #57981, #17536, #4256 ) ;
#18388=ORIENTED_EDGE ( 'NONE', *, *, #46008, .F. ) ;
#18395=DIRECTION ( 'NONE',  ( 0.000000000000000000, 1.000000000000000000, 0.000000000000000000 ) ) ;
#18398=CARTESIAN_POINT ( 'NONE',  ( 4.580390730373999908, -80.21517580634099431, -10.32100728648999954 ) ) ;
#18403=VERTEX_POINT ( 'NONE', #4295 ) ;
#18404=CARTESIAN_POINT ( 'NONE',  ( 2.460597059312418899, -77.04635416667788661, 9.159220230504379501 ) ) ;
#18408=CARTESIAN_POINT ( 'NONE',  ( -9.611650271896834852, -79.74166666666666003, -5.539808784079895965 ) ) ;
#18423=CARTESIAN_POINT ( 'NONE',  ( 5.491552160713999875, -77.15710211417409425, 7.961786551375001686 ) ) ;
#18426=CARTESIAN_POINT ( 'NONE',  ( 10.28103400416999946, -78.12846167599104774, 3.842432268884000024 ) ) ;
#18444=ADVANCED_FACE ( 'NONE', ( #35570 ), #206, .F. ) ;
#18448=ORIENTED_EDGE ( 'NONE', *, *, #9620, .F. ) ;
#18453=CARTESIAN_POINT ( 'NONE',  ( 2.867548251969000095, -77.85841690501798951, -9.270807752789000489 ) ) ;
#18458=CONICAL_SURFACE ( 'NONE', #42014, 9.400000000000000355, 0.7853981633972997312 ) ;
#18471=CARTESIAN_POINT ( 'NONE',  ( 8.819914771577233026, -77.20000000000000284, -6.294782460796893631 ) ) ;
#18474=CARTESIAN_POINT ( 'NONE',  ( 7.059844924164999647, -78.29877966580299642, -8.992308036032000018 ) ) ;
#18475=DIRECTION ( 'NONE',  ( 1.000000000000000000, 0.000000000000000000, 0.000000000000000000 ) ) ;
#18477=CARTESIAN_POINT ( 'NONE',  ( 6.466048582241999299, -79.64649766404198772, 7.299322155150999691 ) ) ;
#18483=CARTESIAN_POINT ( 'NONE',  ( -9.833765687860001492, -77.70380051491399342, 5.287935106362000148 ) ) ;
#18486=CARTESIAN_POINT ( 'NONE',  ( 7.429344776774999382, -78.82343297466498200, 5.780660057059999524 ) ) ;
#18504=AXIS2_PLACEMENT_3D ( 'NONE', #55133, #51821, #14678 ) ;
#18510=DIRECTION ( 'NONE',  ( -0.7071067811865969777, 0.7071067811864980568, 2.974164013349989944E-09 ) ) ;
#18524=CARTESIAN_POINT ( 'NONE',  ( 0.8942477714561651858, -78.73292111987908015, -9.209421948466326668 ) ) ;
#18547=CARTESIAN_POINT ( 'NONE',  ( -1.017498374054518706, -77.33295997921678122, 10.79023145527350991 ) ) ;
#18550=CARTESIAN_POINT ( 'NONE',  ( 8.000000000000000000, -81.99999999999998579, 0.000000000000000000 ) ) ;
#18566=CARTESIAN_POINT ( 'NONE',  ( -9.801770080294998522, -79.26010532903798378, 1.326986863057000088 ) ) ;
#18572=CARTESIAN_POINT ( 'NONE',  ( -1.983076742770497836, -76.97083333328025390, -9.322644974446816946 ) ) ;
#18579=CARTESIAN_POINT ( 'NONE',  ( 0.3796936798447000383, -77.62075755425598800, -11.20547256801999936 ) ) ;
#18581=ORIENTED_EDGE ( 'NONE', *, *, #55117, .F. ) ;
#18583=CARTESIAN_POINT ( 'NONE',  ( -2.217000330786000450, -79.22337286418299129, 9.512392227823999846 ) ) ;
#18595=B_SPLINE_CURVE_WITH_KNOTS ( 'NONE', 3,
 ( #42492, #51938, #11205, #34761, #29183, #47231, #46940, #43647, #6759, #2912 ),
 .UNSPECIFIED., .F., .F.,
 ( 4, 2, 2, 2, 4 ),
 ( 0.000000000000000000, 0.1875000001591858589, 0.3750000003183717179, 0.5625000004775576601, 0.7500000006367434358 ),
 .UNSPECIFIED. ) ;
#18596=CARTESIAN_POINT ( 'NONE',  ( 8.993737204470543034, -79.86887876594592228, 2.161928414312813906 ) ) ;
#18600=CARTESIAN_POINT ( 'NONE',  ( 8.211976133158094271, -76.95750447567392882, -4.859042301739362024 ) ) ;
#18620=CARTESIAN_POINT ( 'NONE',  ( 9.617254819657999221, -78.45270957562398451, -0.5114877307952000463 ) ) ;
#18630=CARTESIAN_POINT ( 'NONE',  ( 9.981840466370998755, -78.77457889078598896, 4.563647388395000171 ) ) ;
#18644=CARTESIAN_POINT ( 'NONE',  ( 0.2631036358232000105, -79.43383300265197988, -11.04575348828999992 ) ) ;
#18651=CARTESIAN_POINT ( 'NONE',  ( -5.755267649934913798, -78.36902568785910717, 9.345839351064629597 ) ) ;
#18652=EDGE_CURVE ( 'NONE', #21753, #27560, #3664, .T. ) ;
#18653=CARTESIAN_POINT ( 'NONE',  ( 0.000000000000000000, -78.59999999921299718, -2.699999999213000379 ) ) ;
#18659=DIRECTION ( 'NONE',  ( -1.000000000000000000, 0.000000000000000000, 0.000000000000000000 ) ) ;
#18669=CARTESIAN_POINT ( 'NONE',  ( -0.5489994406321448972, -77.47989606497139903, 9.234366156267499903 ) ) ;
#18670=CARTESIAN_POINT ( 'NONE',  ( 9.507661145905998978, -77.63772188748299641, -5.611464101879999333 ) ) ;
#18672=CARTESIAN_POINT ( 'NONE',  ( 4.746041175454999816, -77.55612058683698251, -8.464384343845999581 ) ) ;
#18677=CARTESIAN_POINT ( 'NONE',  ( 1.678937288468000055, -78.29192557611499126, 10.81059606312000021 ) ) ;
#18697=CARTESIAN_POINT ( 'NONE',  ( 6.612939829087000732, -79.63308722408299900, 8.759739992124000452 ) ) ;
#18699=DIRECTION ( 'NONE',  ( 0.000000000000000000, 1.000000000000000000, 0.000000000000000000 ) ) ;
#18708=CARTESIAN_POINT ( 'NONE',  ( -8.272053489104999713, -78.23857205644399926, -7.648664291178000063 ) ) ;
#18711=CARTESIAN_POINT ( 'NONE',  ( 5.212684961665999595, -77.00044591236508040, -8.147089634514999901 ) ) ;
#18713=DIRECTION ( 'NONE',  ( 0.000000000000000000, -1.000000000000000000, 0.000000000000000000 ) ) ;
#18714=CARTESIAN_POINT ( 'NONE',  ( 2.550499813263000348, -78.49366228231559717, -10.67515654612000020 ) ) ;
#18720=EDGE_CURVE ( 'NONE', #13326, #49672, #57084, .T. ) ;
#18732=CARTESIAN_POINT ( 'NONE',  ( 2.860217300723919998, -78.25014487812663333, -8.801743088242798052 ) ) ;
#18735=EDGE_LOOP ( 'NONE', ( #20040, #56608, #51639 ) ) ;
#18740=CARTESIAN_POINT ( 'NONE',  ( 4.299999999593000055, -81.99999999959300112, 2.324861064693000045E-09 ) ) ;
#18741=CARTESIAN_POINT ( 'NONE',  ( -9.702231720816998362, -78.71113177888697976, -0.1934140619087000024 ) ) ;
#18757=CARTESIAN_POINT ( 'NONE',  ( 3.887965725239291181, -79.99999999999998579, -8.725614487856105939 ) ) ;
#18764=CARTESIAN_POINT ( 'NONE',  ( -4.854815601933999858, -79.41271639797899695, -8.456988451204999535 ) ) ;
#18773=CARTESIAN_POINT ( 'NONE',  ( -3.967749344305000037, -77.58280535679998025, 10.55286236287999913 ) ) ;
#18777=CARTESIAN_POINT ( 'NONE',  ( 4.657000555087000393, -77.62260406872297835, -8.305583776142999142 ) ) ;
#18811=LINE ( 'NONE', #22650, #32550 ) ;
#18814=CARTESIAN_POINT ( 'NONE',  ( -1.765078173649822668, -78.70978827431009961, -9.079997777801024128 ) ) ;
#18818=CARTESIAN_POINT ( 'NONE',  ( -9.174184873855057987, -80.14666432379901551, -6.068958411681329324 ) ) ;
#18827=CARTESIAN_POINT ( 'NONE',  ( 6.528141900500715522, -79.99999999999998579, 6.772142874866426077 ) ) ;
#18830=CARTESIAN_POINT ( 'NONE',  ( 6.969247251738771354, -79.79316764611728274, -6.112684341057344817 ) ) ;
#18837=CARTESIAN_POINT ( 'NONE',  ( -11.00000000000000000, -78.10953167777607575, -1.317564550621140196 ) ) ;
#18841=EDGE_LOOP ( 'NONE', ( #27690, #45896, #19373, #41519 ) ) ;
#18846=CARTESIAN_POINT ( 'NONE',  ( -8.597176310153894718, -79.99999999999998579, -3.571827255421711200 ) ) ;
#18864=CARTESIAN_POINT ( 'NONE',  ( 10.82024634786000128, -78.24439760156698753, 0.1816028081696000052 ) ) ;
#18868=CARTESIAN_POINT ( 'NONE',  ( 9.523132023602000729, -80.14961334339898258, 1.108936319727999997 ) ) ;
#18878=CARTESIAN_POINT ( 'NONE',  ( 7.032399328097561408, -79.90636888539235372, 6.008881161021868422 ) ) ;
#18894=CARTESIAN_POINT ( 'NONE',  ( -7.730500772889000061, -79.99284890031098882, 8.045567737375000306 ) ) ;
#18905=CARTESIAN_POINT ( 'NONE',  ( 7.201320854070999644, -77.51472321436799007, 6.394856364399000626 ) ) ;
#18911=CARTESIAN_POINT ( 'NONE',  ( 1.210731304718440926, -77.96474580276972688, 9.250079891894303685 ) ) ;
#18915=CARTESIAN_POINT ( 'NONE',  ( -2.879226727952096443, -79.20416666666665151, -10.71369944335146940 ) ) ;
#18935=CARTESIAN_POINT ( 'NONE',  ( 9.009247259181915268, -79.77083333333335702, 2.421167930323361972 ) ) ;
#18936=CARTESIAN_POINT ( 'NONE',  ( -6.920450493081392374, -79.52081221549906331, -8.519106985839389523 ) ) ;
#18942=VERTEX_POINT ( 'NONE', #23106 ) ;
#18954=CARTESIAN_POINT ( 'NONE',  ( 9.147648472655747653, -77.36201978443682492, 1.373573847259280889 ) ) ;
#18955=CARTESIAN_POINT ( 'NONE',  ( -8.283402485401001769, -77.98762868280198290, -7.298588567667000149 ) ) ;
#18965=CARTESIAN_POINT ( 'NONE',  ( 10.68099162494999987, -79.69654329274898430, 2.367326398803000220 ) ) ;
#18976=AXIS2_PLACEMENT_3D ( 'NONE', #25740, #16026, #3032 ) ;
#18980=CARTESIAN_POINT ( 'NONE',  ( 8.297164401012999235, -78.86501084750798896, 4.009864491784999707 ) ) ;
#18985=ORIENTED_EDGE ( 'NONE', *, *, #54547, .T. ) ;
#18986=DIRECTION ( 'NONE',  ( 0.000000000000000000, -1.000000000000000000, 0.000000000000000000 ) ) ;
#18989=CARTESIAN_POINT ( 'NONE',  ( 10.74341457190999982, -79.04314778309698397, -2.245675826504000216 ) ) ;
#18998=CARTESIAN_POINT ( 'NONE',  ( 6.245083526999000156, -78.35094147377398599, -9.376985981987999708 ) ) ;
#19011=LINE ( 'NONE', #37004, #8246 ) ;
#19025=CARTESIAN_POINT ( 'NONE',  ( 3.543073089441956203, -78.25632233163848639, -8.544503082031068786 ) ) ;
#19029=CARTESIAN_POINT ( 'NONE',  ( -8.797281764083550115, -77.57502926220332995, 2.858311938275306385 ) ) ;
#19033=CARTESIAN_POINT ( 'NONE',  ( 9.662203867310999783, -79.02724916671898825, 0.9012207007054000574 ) ) ;
#19054=ORIENTED_EDGE ( 'NONE', *, *, #13316, .T. ) ;
#19059=CARTESIAN_POINT ( 'NONE',  ( -8.906990490675001482, -79.29582576494699708, 3.969308329408999469 ) ) ;
#19067=CARTESIAN_POINT ( 'NONE',  ( 3.020225255027999989, -77.32576797881199582, -10.86205221496000028 ) ) ;
#19070=CARTESIAN_POINT ( 'NONE',  ( 5.750341064076999409, -78.19810873382799343, -7.452836517345999390 ) ) ;
#19077=CARTESIAN_POINT ( 'NONE',  ( 0.000000000000000000, -77.19999999999998863, -9.250000000000047962 ) ) ;
#19088=ORIENTED_EDGE ( 'NONE', *, *, #33890, .T. ) ;
#19096=CARTESIAN_POINT ( 'NONE',  ( -5.681466576401967394, -78.42513435468593741, -7.867322627890024123 ) ) ;
#19100=DIRECTION ( 'NONE',  ( 0.000000000000000000, 1.000000000000000000, 0.000000000000000000 ) ) ;
#19104=CARTESIAN_POINT ( 'NONE',  ( 6.577769324041149446, -78.78812245580762408, -6.503367146901806173 ) ) ;
#19106=EDGE_CURVE ( 'NONE', #2535, #26886, #17617, .T. ) ;
#19109=CARTESIAN_POINT ( 'NONE',  ( -9.956980069057893346, -80.13546169738316394, -4.683283042152130982 ) ) ;
#19119=AXIS2_PLACEMENT_3D ( 'NONE', #11512, #11224, #56092 ) ;
#19125=CARTESIAN_POINT ( 'NONE',  ( -9.733207905157767570, -77.41453182438010572, 4.714720079839265665 ) ) ;
#19126=FACE_OUTER_BOUND ( 'NONE', #42847, .T. ) ;
#19128=CARTESIAN_POINT ( 'NONE',  ( 10.94409238583000032, -78.60603169964656445, 0.8311789410725000105 ) ) ;
#19137=CARTESIAN_POINT ( 'NONE',  ( 8.488869829350999652, -79.17888658829198789, 4.102512142575000631 ) ) ;
#19152=CARTESIAN_POINT ( 'NONE',  ( -9.580931538672000869, -77.88704419146098701, 5.608155544205999377 ) ) ;
#19161=CARTESIAN_POINT ( 'NONE',  ( 8.249323304235000265, -80.21534508975349809, -5.229696851825000437 ) ) ;
#19173=CARTESIAN_POINT ( 'NONE',  ( -8.995441680298000620, -77.13613897360269789, 3.759289608065000010 ) ) ;
#19193=CARTESIAN_POINT ( 'NONE',  ( 7.705600964031999567, -77.19390341397898680, 5.723878957493999664 ) ) ;
#19199=CARTESIAN_POINT ( 'NONE',  ( 5.053427186728000287, -78.53798106301098869, 8.198541555267000902 ) ) ;
#19205=DIRECTION ( 'NONE',  ( 0.000000000000000000, -1.000000000000000000, 0.000000000000000000 ) ) ;
#19208=CARTESIAN_POINT ( 'NONE',  ( 6.718030245586000149, -79.16787185144298178, -8.679405866825000260 ) ) ;
#19224=CARTESIAN_POINT ( 'NONE',  ( 11.00000000000000000, -77.94999999999998863, 0.000000000000000000 ) ) ;
#19225=CARTESIAN_POINT ( 'NONE',  ( 10.87605760524872345, -79.68936634149505949, -1.476207922926128457 ) ) ;
#19244=CARTESIAN_POINT ( 'NONE',  ( 8.964791593824459781, -77.37004751899343091, 2.291628598551814999 ) ) ;
#19245=CARTESIAN_POINT ( 'NONE',  ( 3.792698199283999649, -78.14336073446899888, -10.36819406884000117 ) ) ;
#19247=CARTESIAN_POINT ( 'NONE',  ( 7.256139241522999939, -77.69823973248199422, 6.443535727668999513 ) ) ;
#19253=CARTESIAN_POINT ( 'NONE',  ( 10.94008345411999983, -78.17955615878399556, 0.05084573220516999670 ) ) ;
#19257=EDGE_CURVE ( 'NONE', #55023, #30580, #41737, .T. ) ;
#19270=CARTESIAN_POINT ( 'NONE',  ( 5.750341064076999409, -77.75648151147798615, -7.452836517345999390 ) ) ;
#19276=AXIS2_PLACEMENT_3D ( 'NONE', #51900, #48622, #16169 ) ;
#19277=CARTESIAN_POINT ( 'NONE',  ( -4.299999999593000055, -81.99999999959300112, -2.324862195016999523E-09 ) ) ;
#19280=CARTESIAN_POINT ( 'NONE',  ( 7.218984044805000444, -79.12742484609498206, 8.267423174273998754 ) ) ;
#19292=DIRECTION ( 'NONE',  ( 0.000000000000000000, 1.000000000000000000, 0.000000000000000000 ) ) ;
#19317=CARTESIAN_POINT ( 'NONE',  ( 1.852771442128949175, -78.24118117197441791, -9.062483227336022296 ) ) ;
#19321=CARTESIAN_POINT ( 'NONE',  ( -7.746552609361182284, -77.55398491059833077, 5.056132427002594909 ) ) ;
#19325=CARTESIAN_POINT ( 'NONE',  ( -4.814859605045999302, -78.68616321717099993, 8.425427962446999430 ) ) ;
#19339=CARTESIAN_POINT ( 'NONE',  ( 0.6056868765398906174, -79.46999359693003839, 9.249787030607762972 ) ) ;
#19356=CARTESIAN_POINT ( 'NONE',  ( 3.952028055797999873, -77.52568593946898545, 10.55876001981000023 ) ) ;
#19366=DIRECTION ( 'NONE',  ( -0.7071067811864970576, -0.7071067811865969777, -3.680441358138984842E-08 ) ) ;
#19367=ORIENTED_EDGE ( 'NONE', *, *, #39188, .T. ) ;
#19373=ORIENTED_EDGE ( 'NONE', *, *, #51295, .T. ) ;
#19381=CARTESIAN_POINT ( 'NONE',  ( -9.312499999988999022, -77.13750000001088836, -2.050180145195999796E-09 ) ) ;
#19384=ORIENTED_EDGE ( 'NONE', *, *, #48516, .F. ) ;
#19387=ORIENTED_EDGE ( 'NONE', *, *, #5120, .T. ) ;
#19392=CARTESIAN_POINT ( 'NONE',  ( 8.898653440358000211, -78.46734835141977271, -3.871004561473999850 ) ) ;
#19396=CARTESIAN_POINT ( 'NONE',  ( -7.227278212944055369, -78.65368819820857027, -5.773064082365189975 ) ) ;
#19409=LINE ( 'NONE', #19700, #11065 ) ;
#19418=CARTESIAN_POINT ( 'NONE',  ( 10.02592289919787305, -77.23099517276321535, 4.055125067876876876 ) ) ;
#19425=AXIS2_PLACEMENT_3D ( 'NONE', #55430, #31807, #9394 ) ;
#19427=CARTESIAN_POINT ( 'NONE',  ( 9.197769436456411540, -78.34157941349792509, -0.9820442832495991370 ) ) ;
#19430=DIRECTION ( 'NONE',  ( 1.000000000000000000, 0.000000000000000000, 0.000000000000000000 ) ) ;
#19431=CARTESIAN_POINT ( 'NONE',  ( 9.618404959434000645, -78.09175299886499033, 1.531659799953999812 ) ) ;
#19436=CIRCLE ( 'NONE', #37368, 10.69999999999999929 ) ;
#19443=CARTESIAN_POINT ( 'NONE',  ( 9.250000000000000000, -77.74999999999998579, 0.000000000000000000 ) ) ;
#19444=CARTESIAN_POINT ( 'NONE',  ( 1.838439579890999820, -80.04146898612899008, 11.40569499701999945 ) ) ;
#19451=CARTESIAN_POINT ( 'NONE',  ( -9.387315177295000979, -79.98803648194748916, 2.697965643110000311 ) ) ;
#19466=EDGE_CURVE ( 'NONE', #54466, #55944, #26239, .T. ) ;
#19467=AXIS2_PLACEMENT_3D ( 'NONE', #11198, #52493, #34462 ) ;
#19474=DIRECTION ( 'NONE',  ( 1.000000000000000000, 0.000000000000000000, 0.000000000000000000 ) ) ;
#19479=CARTESIAN_POINT ( 'NONE',  ( -6.246652488582999929, -77.32445024881999984, 7.288235269262000493 ) ) ;
#19484=CARTESIAN_POINT ( 'NONE',  ( -6.424145201942000227, -78.14004745520499284, 7.175205111309999495 ) ) ;
#19486=CARTESIAN_POINT ( 'NONE',  ( 10.26300017817221999, -77.91922858884991854, -4.172146172881584292 ) ) ;
#19493=CARTESIAN_POINT ( 'NONE',  ( -9.813193589766999736, -79.02741007977999743, -4.915816122623000162 ) ) ;
#19495=CARTESIAN_POINT ( 'NONE',  ( 4.081138785858000162, -78.91908747365698673, 8.644947643559998340 ) ) ;
#19500=CARTESIAN_POINT ( 'NONE',  ( -9.164301350569918014, -77.48739481387521266, 1.453017405635841808 ) ) ;
#19507=ADVANCED_FACE ( 'NONE', ( #50475 ), #13480, .F. ) ;
#19514=CARTESIAN_POINT ( 'NONE',  ( -10.13801387673548682, -78.48139510519006024, -4.205769073302976224 ) ) ;
#19522=AXIS2_PLACEMENT_3D ( 'NONE', #36793, #4929, #41521 ) ;
#19533=CARTESIAN_POINT ( 'NONE',  ( 8.794698800388047744, -77.37511376347532632, 2.866210580583882450 ) ) ;
#19540=CARTESIAN_POINT ( 'NONE',  ( 10.92979202429999930, -79.25475665554398574, 1.617881315982000245 ) ) ;
#19545=CARTESIAN_POINT ( 'NONE',  ( -10.96763318152921407, -77.20000000000001705, 0.8289010833759121732 ) ) ;
#19562=VECTOR ( 'NONE', #42029, 1000.000000000000114 ) ;
#19565=CARTESIAN_POINT ( 'NONE',  ( -7.508490145779999736, -78.87459365710098780, -8.005410190140000992 ) ) ;
#19574=CARTESIAN_POINT ( 'NONE',  ( -10.40633193566000081, -78.21047970211098743, -4.317081191017999586 ) ) ;
#19586=SURFACE_SIDE_STYLE ('',( #46477 ) ) ;
#19601=CARTESIAN_POINT ( 'NONE',  ( 6.545761160578629223, -78.28756486186320274, -6.535701422592273602 ) ) ;
#19610=CARTESIAN_POINT ( 'NONE',  ( 1.260641617779999946, -77.63448153939899044, 9.621927669549000584 ) ) ;
#19617=CYLINDRICAL_SURFACE ( 'NONE', #35667, 1.000000000000000000 ) ;
#19629=CARTESIAN_POINT ( 'NONE',  ( 8.600237018945074752, -77.19999999999998863, -6.594552368571869216 ) ) ;
#19634=CARTESIAN_POINT ( 'NONE',  ( -2.879226727952091114, -79.09583333333331723, 10.71369944335146940 ) ) ;
#19636=CARTESIAN_POINT ( 'NONE',  ( 6.393851920857000160, -79.71037340482598665, 7.217821578210998901 ) ) ;
#19642=CARTESIAN_POINT ( 'NONE',  ( 0.000000000000000000, -75.10000000032299283, 0.000000000000000000 ) ) ;
#19643=CARTESIAN_POINT ( 'NONE',  ( -4.822148453319999639, -77.33252430226399099, -10.07035697449999923 ) ) ;
#19646=CARTESIAN_POINT ( 'NONE',  ( -8.334831687997999339, -78.48234702511798844, 4.375131454052000102 ) ) ;
#19681=CARTESIAN_POINT ( 'NONE',  ( -5.681372509047000641, -78.32522920577524417, -7.867192369580999767 ) ) ;
#19686=CARTESIAN_POINT ( 'NONE',  ( -7.833419388303895836, -78.64479959160827605, -4.919153442762366879 ) ) ;
#19691=CARTESIAN_POINT ( 'NONE',  ( -5.622587949631386195, -80.18243779068814092, -9.454352941869160531 ) ) ;
#19700=CARTESIAN_POINT ( 'NONE',  ( 11.00000000000000000, -78.94999999999998863, -1.064824513673000067E-14 ) ) ;
#19709=CARTESIAN_POINT ( 'NONE',  ( 6.634077760214808883, -78.12828546955671527, -8.488125058123570099 ) ) ;
#19710=CARTESIAN_POINT ( 'NONE',  ( -0.1577822530794796563, -78.22391181108908143, -11.07750337872512780 ) ) ;
#19711=CARTESIAN_POINT ( 'NONE',  ( 8.867070753125000593, -78.54984699098105239, -6.468312982590000537 ) ) ;
#19718=CARTESIAN_POINT ( 'NONE',  ( 9.035162686194604831, -78.33298600581431970, -1.982237826727912156 ) ) ;
#19722=CARTESIAN_POINT ( 'NONE',  ( 9.189097042878000110, -78.66725766396999120, 2.883349701574000168 ) ) ;
#19733=CARTESIAN_POINT ( 'NONE',  ( -2.948156184611000263, -78.70343179000198575, 10.64829886688000116 ) ) ;
#19734=CARTESIAN_POINT ( 'NONE',  ( 7.421131282012294328, -77.69826720182105362, -5.651170926980095821 ) ) ;
#19738=CARTESIAN_POINT ( 'NONE',  ( -4.809507827685000514, -77.21046664206399157, -10.07512781268000168 ) ) ;
#19746=CARTESIAN_POINT ( 'NONE',  ( -5.809791519574999619, -79.31614844811198850, 7.851562197947999699 ) ) ;
#19755=DIRECTION ( 'NONE',  ( -1.308367906941000013E-10, -1.000000000000000000, -3.608117760387000167E-10 ) ) ;
#19757=CARTESIAN_POINT ( 'NONE',  ( 2.941330672729000284, -77.07006883366948102, 9.389085009981000596 ) ) ;
#19774=CARTESIAN_POINT ( 'NONE',  ( 2.291826089449000126, -77.03724721216990190, -9.321303964228999206 ) ) ;
#19781=CARTESIAN_POINT ( 'NONE',  ( -9.316314781052998484, -77.29436066386098503, -2.840095070410999956 ) ) ;
#19784=CARTESIAN_POINT ( 'NONE',  ( -9.834111732579202680, -77.73812671110431438, -5.101590220333413583 ) ) ;
#19792=CARTESIAN_POINT ( 'NONE',  ( -3.673218652927999539, -79.39261068610500161, 10.34270183798999909 ) ) ;
#19794=CARTESIAN_POINT ( 'NONE',  ( -9.029190506544999550, -79.10582576494698515, -3.140825197024999849 ) ) ;
#19811=CYLINDRICAL_SURFACE ( 'NONE', #6669, 5.000000000000000000 ) ;
#19812=CARTESIAN_POINT ( 'NONE',  ( 10.28119625626286116, -78.22856391619605176, 3.842492908960651210 ) ) ;
#19828=ORIENTED_EDGE ( 'NONE', *, *, #38046, .T. ) ;
#19831=CARTESIAN_POINT ( 'NONE',  ( 8.796562682441143366, -77.37506290377116613, 2.860481962223264230 ) ) ;
#19837=CARTESIAN_POINT ( 'NONE',  ( 0.1299632413661999941, -79.36712607287400090, 11.04812215732000169 ) ) ;
#19848=FACE_BOUND ( 'NONE', #49983, .T. ) ;
#19854=CARTESIAN_POINT ( 'NONE',  ( 0.8359750594766999221, -78.21126277754198952, -9.376158072868999938 ) ) ;
#19865=CARTESIAN_POINT ( 'NONE',  ( -7.022507694776999543, -79.23979426342499721, 8.434951230355999030 ) ) ;
#19866=CARTESIAN_POINT ( 'NONE',  ( 0.000000000000000000, -80.49999999999998579, -5.000000000000000000 ) ) ;
#19893=ORIENTED_EDGE ( 'NONE', *, *, #54006, .T. ) ;
#19895=ADVANCED_FACE ( 'NONE', ( #42640, #3350 ), #21346, .T. ) ;
#19897=CARTESIAN_POINT ( 'NONE',  ( 0.000000000000000000, -74.64999999999999147, 0.000000000000000000 ) ) ;
#19901=CARTESIAN_POINT ( 'NONE',  ( 7.109588333167061514, -78.29483705384265591, -5.917559077586919791 ) ) ;
#19903=ORIENTED_EDGE ( 'NONE', *, *, #24024, .T. ) ;
#19905=CARTESIAN_POINT ( 'NONE',  ( -9.079656017920873623, -77.58448292774525612, 1.803135903180888899 ) ) ;
#19907=CARTESIAN_POINT ( 'NONE',  ( 0.000000000000000000, -75.09999999979599750, 0.000000000000000000 ) ) ;
#19910=CARTESIAN_POINT ( 'NONE',  ( 2.867548251969000095, -77.91871983068898544, -9.270807752789000489 ) ) ;
#19918=FACE_OUTER_BOUND ( 'NONE', #32713, .T. ) ;
#19930=CARTESIAN_POINT ( 'NONE',  ( -6.760013919724056741, -78.27291666666666003, -8.796335266379987416 ) ) ;
#19932=CARTESIAN_POINT ( 'NONE',  ( -6.760013919724083387, -79.12708333333333144, 8.796335266379969653 ) ) ;
#19935=VECTOR ( 'NONE', #47203, 1000.000000000000114 ) ;
#19936=CARTESIAN_POINT ( 'NONE',  ( 9.531612390470000307, -79.15514289792399438, 1.458175310291999871 ) ) ;
#19938=CARTESIAN_POINT ( 'NONE',  ( -1.489475662155156366, -79.46257339460650826, -9.601386891029047632 ) ) ;
#19942=CARTESIAN_POINT ( 'NONE',  ( -5.700319242863999492, -77.22504179105499134, 9.473880686520999461 ) ) ;
#19947=CARTESIAN_POINT ( 'NONE',  ( -9.338489578732000140, -78.51077085424698510, 1.184823571421999899 ) ) ;
#19954=DIRECTION ( 'NONE',  ( -7.037892281487000491E-12, 1.000000000000000000, 4.198156442306999976E-10 ) ) ;
#19977=CARTESIAN_POINT ( 'NONE',  ( 4.635655000267153270, -79.26679008495354140, -8.026958512551585656 ) ) ;
#19982=CARTESIAN_POINT ( 'NONE',  ( -1.182190922889000184, -78.86528195922576856, -9.631881180458998770 ) ) ;
#19987=CARTESIAN_POINT ( 'NONE',  ( -5.529498250248094493, -78.67420770746792869, -7.421320449266156416 ) ) ;
#19991=CARTESIAN_POINT ( 'NONE',  ( -7.516303886515633970, -80.16556818807158891, -8.031330139908581245 ) ) ;
#20010=CARTESIAN_POINT ( 'NONE',  ( 5.542538650459465366, -77.61846143728747904, -9.237786168586172408 ) ) ;
#20012=CARTESIAN_POINT ( 'NONE',  ( -4.399243655502999673, -79.75781822728644954, 10.05537673064999993 ) ) ;
#20017=DIRECTION ( 'NONE',  ( 1.000000000000000000, 0.000000000000000000, 0.000000000000000000 ) ) ;
#20021=CARTESIAN_POINT ( 'NONE',  ( -5.177883096403999907, -77.40958109976999424, -8.249196342081999589 ) ) ;
#20031=CARTESIAN_POINT ( 'NONE',  ( 7.840491480036000382, -78.61915472700400187, 7.784894796889999746 ) ) ;
#20032=CARTESIAN_POINT ( 'NONE',  ( 11.39907318373000145, -79.91618549011299422, -1.879061223299000050 ) ) ;
#20035=CARTESIAN_POINT ( 'NONE',  ( -8.657507096519999834, -77.50120975171299165, 7.296561482783999075 ) ) ;
#20040=ORIENTED_EDGE ( 'NONE', *, *, #50103, .F. ) ;
#20045=CARTESIAN_POINT ( 'NONE',  ( 8.249323304235000265, -80.33519793320401448, -5.229696851825000437 ) ) ;
#20058=CARTESIAN_POINT ( 'NONE',  ( -6.259101251364000085, -77.20009236341799408, 7.707182931745999888 ) ) ;
#20072=AXIS2_PLACEMENT_3D ( 'NONE', #37842, #34558, #38421 ) ;
#20076=CARTESIAN_POINT ( 'NONE',  ( 7.282635111839001141, -77.57859895515098003, 6.467064367534000269 ) ) ;
#20078=CARTESIAN_POINT ( 'NONE',  ( 4.977885330626823368, -77.86203852219340149, -9.897304379485548864 ) ) ;
#20084=DIRECTION ( 'NONE',  ( 0.000000000000000000, -1.000000000000000000, 0.000000000000000000 ) ) ;
#20086=CARTESIAN_POINT ( 'NONE',  ( -10.95938340363141528, -80.09357446033341432, 0.9416311679418450931 ) ) ;
#20087=CARTESIAN_POINT ( 'NONE',  ( -7.768786981737000552, -79.62869298055800016, -5.571087248544999149 ) ) ;
#20106=CARTESIAN_POINT ( 'NONE',  ( -5.809791519574999619, -79.13523967109999546, 7.851562197947999699 ) ) ;
#20124=CARTESIAN_POINT ( 'NONE',  ( 9.219793351069757392, -77.35649433367561301, 0.7464174168656269037 ) ) ;
#20125=CARTESIAN_POINT ( 'NONE',  ( -1.776188306762000124, -77.60259568715798650, -10.89629776253999971 ) ) ;
#20130=DIRECTION ( 'NONE',  ( 0.000000000000000000, 1.000000000000000000, 0.000000000000000000 ) ) ;
#20134=CARTESIAN_POINT ( 'NONE',  ( -10.20553722967999910, -78.52435544289399161, -4.233781229625999565 ) ) ;
#20148=CARTESIAN_POINT ( 'NONE',  ( -5.004442145019999622, -77.15958109976958212, -7.972877152348999630 ) ) ;
#20151=DIRECTION ( 'NONE',  ( -1.000000000000000000, 0.000000000000000000, 0.000000000000000000 ) ) ;
#20159=CARTESIAN_POINT ( 'NONE',  ( 8.867070753125000593, -78.56969597644598480, -6.468312982590000537 ) ) ;
#20167=CARTESIAN_POINT ( 'NONE',  ( 8.796335266379964324, -78.00208333333334565, 6.760013919724087827 ) ) ;
#20170=CARTESIAN_POINT ( 'NONE',  ( 10.99934742197999960, -79.44654329274898430, 2.437886521773999782 ) ) ;
#20180=ADVANCED_FACE ( 'NONE', ( #42823 ), #30081, .T. ) ;
#20188=CARTESIAN_POINT ( 'NONE',  ( -10.49924843836999777, -80.37932778397052402, -4.054558598941000014 ) ) ;
#20194=CIRCLE ( 'NONE', #38088, 10.69999999999999929 ) ;
#20197=CARTESIAN_POINT ( 'NONE',  ( -9.195808504226482327, -77.59150866904204236, 1.005241119271180095 ) ) ;
#20201=CARTESIAN_POINT ( 'NONE',  ( 8.553489385229999797, -79.05567299584799912, 4.133741566275999979 ) ) ;
#20207=DIRECTION ( 'NONE',  ( 1.000000000000000000, 0.000000000000000000, 0.000000000000000000 ) ) ;
#20213=CARTESIAN_POINT ( 'NONE',  ( -10.02842745654077561, -80.28333333334607858, -4.462749333579311362 ) ) ;
#20219=CARTESIAN_POINT ( 'NONE',  ( -8.102049197848998574, -80.36951364748298943, 7.545907228784999532 ) ) ;
#20227=CARTESIAN_POINT ( 'NONE',  ( 2.018311730614999799, -79.59891319606099103, -9.317554422237000367 ) ) ;
#20231=CARTESIAN_POINT ( 'NONE',  ( -8.796335266379976758, -77.25208333333331723, -6.760013919724066511 ) ) ;
#20233=CARTESIAN_POINT ( 'NONE',  ( 9.634437611857999073, -77.66019374448798374, 5.199262921030999962 ) ) ;
#20240=CARTESIAN_POINT ( 'NONE',  ( -9.250000000000000000, -79.49999999999998579, 1.813240672189999963E-14 ) ) ;
#20258=ORIENTED_EDGE ( 'NONE', *, *, #30663, .F. ) ;
#20274=CARTESIAN_POINT ( 'NONE',  ( -7.891267276537118569, -78.64385383780864913, -4.825895275192899625 ) ) ;
#20285=AXIS2_PLACEMENT_3D ( 'NONE', #32888, #1931, #52090 ) ;
#20291=CARTESIAN_POINT ( 'NONE',  ( 10.47234974255967366, -77.67964032115997952, -2.795332386398399649 ) ) ;
#20294=CARTESIAN_POINT ( 'NONE',  ( -0.5193979750644999172, -78.97123230597145493, -10.96331347381999954 ) ) ;
#20299=CARTESIAN_POINT ( 'NONE',  ( 8.470860587981800194, -78.31708216412036450, -3.718899516019706919 ) ) ;
#20300=CARTESIAN_POINT ( 'NONE',  ( 0.000000000000000000, -74.99999999999998579, 0.000000000000000000 ) ) ;
#20303=CARTESIAN_POINT ( 'NONE',  ( 4.763371395742999503, -77.49485258715699842, -8.495292134120999705 ) ) ;
#20315=ORIENTED_EDGE ( 'NONE', *, *, #2345, .F. ) ;
#20318=CARTESIAN_POINT ( 'NONE',  ( -9.771309935692000792, -78.01479567302799012, 5.719592689793999263 ) ) ;
#20323=CARTESIAN_POINT ( 'NONE',  ( 3.269429986698999979, -80.09785153581056250, 9.203886808668999109 ) ) ;
#20336=CARTESIAN_POINT ( 'NONE',  ( 8.796335266379994522, -79.79791666666667993, -6.760013919724047859 ) ) ;
#20340=CARTESIAN_POINT ( 'NONE',  ( 8.082524092276875294, -77.79166666666667140, 4.658475568430836766 ) ) ;
#20352=FACE_OUTER_BOUND ( 'NONE', #50317, .T. ) ;
#20358=CARTESIAN_POINT ( 'NONE',  ( 4.561861969681999973, -77.60702278427999090, 8.605179316909000065 ) ) ;
#20360=CARTESIAN_POINT ( 'NONE',  ( -7.473530897346515545, -77.10494791667788661, 5.742368499590185138 ) ) ;
#20362=FACE_OUTER_BOUND ( 'NONE', #32319, .T. ) ;
#20367=CARTESIAN_POINT ( 'NONE',  ( -9.499121195477519208, -79.25069084405711806, -0.08246750231446209334 ) ) ;
#20368=CARTESIAN_POINT ( 'NONE',  ( 0.000000000000000000, -80.49999999999998579, 0.000000000000000000 ) ) ;
#20373=CARTESIAN_POINT ( 'NONE',  ( -10.99999999999999822, -78.61041666666666572, -1.439896632895323325 ) ) ;
#20384=CARTESIAN_POINT ( 'NONE',  ( 0.000000000000000000, -74.64999999999999147, 0.000000000000000000 ) ) ;
#20388=VERTEX_POINT ( 'NONE', #13545 ) ;
#20394=CONICAL_SURFACE ( 'NONE', #22278, 4.199999999630000147, 0.7853981633972997312 ) ;
#20408=CARTESIAN_POINT ( 'NONE',  ( 9.249917852137487628, -77.35035757946567969, 0.04157983743616296135 ) ) ;
#20409=CARTESIAN_POINT ( 'NONE',  ( -8.283402485401001769, -78.04793160847299305, -7.298588567667000149 ) ) ;
#20419=CARTESIAN_POINT ( 'NONE',  ( 1.695617993698999904, -78.35580131689798122, 10.91800231797999921 ) ) ;
#20433=CARTESIAN_POINT ( 'NONE',  ( -9.446372167179999835, -78.13301937267999620, 1.198511206093999970 ) ) ;
#20438=ORIENTED_EDGE ( 'NONE', *, *, #43478, .T. ) ;
#20445=CARTESIAN_POINT ( 'NONE',  ( 6.083963560182000130, -78.54160362211398194, -9.135064530700001129 ) ) ;
#20458=CARTESIAN_POINT ( 'NONE',  ( -0.5331530516160000177, -78.80041914309698825, -11.25365194899999999 ) ) ;
#20467=CARTESIAN_POINT ( 'NONE',  ( 0.000000000000000000, -78.69999999999998863, 0.000000000000000000 ) ) ;
#20479=CARTESIAN_POINT ( 'NONE',  ( -1.794546681526326459, -78.20953827855916529, -9.074208611156969084 ) ) ;
#20483=CARTESIAN_POINT ( 'NONE',  ( -7.483760668707474473, -77.55000130354729038, 5.436515708445330830 ) ) ;
#20484=DIRECTION ( 'NONE',  ( 0.000000000000000000, -1.000000000000000000, 0.000000000000000000 ) ) ;
#20487=CARTESIAN_POINT ( 'NONE',  ( -3.536681740116999872, -78.23483721851999917, 9.036735673663999435 ) ) ;
#20503=CARTESIAN_POINT ( 'NONE',  ( -8.564747023678000559, -80.00360881430898985, 6.787585331471000849 ) ) ;
#20510=DIRECTION ( 'NONE',  ( 0.000000000000000000, 0.000000000000000000, -1.000000000000000000 ) ) ;
#20513=CARTESIAN_POINT ( 'NONE',  ( -9.063895419714999235, -79.48202256302897695, -2.955706763204999810 ) ) ;
#20515=CARTESIAN_POINT ( 'NONE',  ( -9.237485228140851490, -79.37490541983250125, -3.012313834119925815 ) ) ;
#20517=DIRECTION ( 'NONE',  ( -1.000000000000000000, 0.000000000000000000, 0.000000000000000000 ) ) ;
#20520=CARTESIAN_POINT ( 'NONE',  ( -0.9587802219394000458, -77.48883549249599412, -10.90575368789999899 ) ) ;
#20525=CARTESIAN_POINT ( 'NONE',  ( -3.831287612370999796, -76.80151196011908610, -8.693171758988999187 ) ) ;
#20527=CARTESIAN_POINT ( 'NONE',  ( 10.71369944335146762, -77.37083333333333712, 2.879226727952103548 ) ) ;
#20550=EDGE_LOOP ( 'NONE', ( #26679, #7018, #11474, #44448 ) ) ;
#20561=CARTESIAN_POINT ( 'NONE',  ( -1.799702852821704058, -78.70948991200978639, -9.073181958675275993 ) ) ;
#20580=CARTESIAN_POINT ( 'NONE',  ( -10.25114915300409280, -77.97533825987605383, -3.311110282731340337 ) ) ;
#20592=CARTESIAN_POINT ( 'NONE',  ( 1.475792658273999969, -77.53030449881099173, -9.517102871385000995 ) ) ;
#20597=DIRECTION ( 'NONE',  ( 0.000000000000000000, -1.000000000000000000, 0.000000000000000000 ) ) ;
#20600=CARTESIAN_POINT ( 'NONE',  ( -1.293339008660999934, -78.48638398745899281, -10.86347506762000137 ) ) ;
#20601=CARTESIAN_POINT ( 'NONE',  ( 8.097906714174317955, -77.70861376145681731, -4.629560367825112266 ) ) ;
#20603=ORIENTED_EDGE ( 'NONE', *, *, #7583, .T. ) ;
#20604=CARTESIAN_POINT ( 'NONE',  ( -11.29558555235000128, -78.05148038169298275, 0.7758774409984000586 ) ) ;
#20610=CARTESIAN_POINT ( 'NONE',  ( 3.269429986698999979, -79.97799869236203563, 9.203886808668999109 ) ) ;
#20614=VERTEX_POINT ( 'NONE', #39405 ) ;
#20617=EDGE_CURVE ( 'NONE', #13297, #48890, #7822, .T. ) ;
#20632=DIRECTION ( 'NONE',  ( 1.000000000000000000, 0.000000000000000000, 0.000000000000000000 ) ) ;
#20637=CARTESIAN_POINT ( 'NONE',  ( 7.418149392330000147, -77.15334168688949035, -5.919552685632999633 ) ) ;
#20642=CARTESIAN_POINT ( 'NONE',  ( -9.190938788893999956, -78.74397594943899037, 3.222784492720999872 ) ) ;
#20651=CARTESIAN_POINT ( 'NONE',  ( 9.425379270812129562, -79.01124851720528852, 1.342142796262536963 ) ) ;
#20656=CARTESIAN_POINT ( 'NONE',  ( 3.149121100232000092, -79.92747424662198341, 9.026342880292000714 ) ) ;
#20658=CARTESIAN_POINT ( 'NONE',  ( -5.539808784079886195, -78.68333333333332291, -9.611650271896841957 ) ) ;
#20666=EDGE_LOOP ( 'NONE', ( #43748, #17476, #47135, #50466, #24679 ) ) ;
#20673=CARTESIAN_POINT ( 'NONE',  ( 6.728605944993000243, -79.39502093716299669, -7.080011783993000130 ) ) ;
#20681=CARTESIAN_POINT ( 'NONE',  ( 10.99999999999999822, -77.46041666666667425, 1.439896632895345086 ) ) ;
#20694=CARTESIAN_POINT ( 'NONE',  ( 3.218370493427320067, -77.25342817773334048, -8.672750898853246682 ) ) ;
#20704=CARTESIAN_POINT ( 'NONE',  ( -2.948156184611000263, -78.88955604921899578, 10.64829886688000116 ) ) ;
#20718=CARTESIAN_POINT ( 'NONE',  ( -0.5444512524326000635, -77.76350959400299701, -9.506521396690999381 ) ) ;
#20731=CARTESIAN_POINT ( 'NONE',  ( -3.548303639235999896, -79.46865131509198932, -10.38621961377000069 ) ) ;
#20740=CARTESIAN_POINT ( 'NONE',  ( -9.611650271896857944, -78.15833333333333144, 5.539808784079855997 ) ) ;
#20741=CARTESIAN_POINT ( 'NONE',  ( -2.205131412320000095, -78.13389367123097884, 10.93750404997000025 ) ) ;
#20751=CARTESIAN_POINT ( 'NONE',  ( -9.250000000000000000, -78.99999999999998579, 0.000000000000000000 ) ) ;
#20753=ORIENTED_EDGE ( 'NONE', *, *, #20888, .F. ) ;
#20762=CARTESIAN_POINT ( 'NONE',  ( 1.809879502519539995, -78.24079858881482608, -9.071132683527801888 ) ) ;
#20765=CONICAL_SURFACE ( 'NONE', #49043, 1.099999997149000430, 0.7853981633972997312 ) ;
#20767=CARTESIAN_POINT ( 'NONE',  ( -7.047464712085933947, -77.54400991620123307, 5.991240863339566403 ) ) ;
#20770=CARTESIAN_POINT ( 'NONE',  ( 4.545264886168000729, -77.66636063594098971, 8.573871732259998879 ) ) ;
#20772=CARTESIAN_POINT ( 'NONE',  ( -9.250000000000000000, -77.50056085624700586, -0.06519332902036732713 ) ) ;
#20774=CARTESIAN_POINT ( 'NONE',  ( -7.179058446792000225, -79.93980297709798322, -8.667882172381000672 ) ) ;
#20785=CARTESIAN_POINT ( 'NONE',  ( -0.2814639899600999695, -80.05216315943599170, -11.06814981317999980 ) ) ;
#20788=EDGE_LOOP ( 'NONE', ( #3930, #36929 ) ) ;
#20793=CARTESIAN_POINT ( 'NONE',  ( 3.376184802135000051, -79.73959606308299897, 9.032146306647000245 ) ) ;
#20795=CARTESIAN_POINT ( 'NONE',  ( 9.549999999999998934, -79.99999999999998579, 0.000000000000000000 ) ) ;
#20798=CARTESIAN_POINT ( 'NONE',  ( 2.879226727952094222, -77.34583333333328881, -10.71369944335146940 ) ) ;
#20800=CARTESIAN_POINT ( 'NONE',  ( 2.961948693619000039, -77.45351946037798996, -10.65246418773999970 ) ) ;
#20805=CARTESIAN_POINT ( 'NONE',  ( -2.880544446985999762, -76.87051800811249791, -9.112186890989001142 ) ) ;
#20821=CARTESIAN_POINT ( 'NONE',  ( 3.321932689531000182, -77.19999999999998863, 10.22385755016999909 ) ) ;
#20829=ORIENTED_EDGE ( 'NONE', *, *, #36869, .F. ) ;
#20839=CARTESIAN_POINT ( 'NONE',  ( -10.71369944335148361, -78.67916666666667425, 2.879226727952040044 ) ) ;
#20843=B_SPLINE_CURVE_WITH_KNOTS ( 'NONE', 3,
 ( #4658, #30117, #3278, #53959, #13496, #49533, #43726, #9079, #22355, #40369, #18241, #34545, #30407, #48165, #7696, #27066, #4945, #16562 ),
 .UNSPECIFIED., .F., .F.,
 ( 4, 2, 2, 2, 2, 2, 2, 2, 4 ),
 ( 0.000000000000000000, 0.1249999999999999445, 0.2499999999999998890, 0.3749999999999999445, 0.5000000000000000000, 0.6250000000000000000, 0.7500000000000001110, 0.8750000000000000000, 1.000000000000000000 ),
 .UNSPECIFIED. ) ;
#20845=CARTESIAN_POINT ( 'NONE',  ( -10.89688518808336148, -80.11107775181403667, -1.501841381199422898 ) ) ;
#20849=LINE ( 'NONE', #2568, #10045 ) ;
#20866=VERTEX_POINT ( 'NONE', #37295 ) ;
#20872=CARTESIAN_POINT ( 'NONE',  ( -6.424145201942000227, -78.32617171442198867, 7.175205111309999495 ) ) ;
#20878=CARTESIAN_POINT ( 'NONE',  ( 6.919235075806907886, -78.90838314311494628, 6.169169527640317341 ) ) ;
#20881=CARTESIAN_POINT ( 'NONE',  ( -4.969435546850999863, -78.45829163312599519, -9.746410964130999943 ) ) ;
#20883=CARTESIAN_POINT ( 'NONE',  ( 1.820702833782999797, -80.10534472691198005, 11.29565607131000071 ) ) ;
#20888=EDGE_CURVE ( 'NONE', #28211, #604, #45891, .T. ) ;
#20890=CARTESIAN_POINT ( 'NONE',  ( -8.448510849392999233, -79.58832679327100834, 4.901364000006999788 ) ) ;
#20891=B_SPLINE_CURVE_WITH_KNOTS ( 'NONE', 3,
 ( #5105, #23104, #22522, #10121 ),
 .UNSPECIFIED., .F., .F.,
 ( 4, 4 ),
 ( 0.000000000000000000, 1.000000000000000000 ),
 .UNSPECIFIED. ) ;
#20906=CARTESIAN_POINT ( 'NONE',  ( -11.00000000000000000, -78.59999999999999432, 0.000000000000000000 ) ) ;
#20910=CARTESIAN_POINT ( 'NONE',  ( 4.658475568430798575, -77.83333333333332860, 8.082524092276898386 ) ) ;
#20918=B_SPLINE_CURVE_WITH_KNOTS ( 'NONE', 3,
 ( #40683, #32383, #14101, #5529 ),
 .UNSPECIFIED., .F., .F.,
 ( 4, 4 ),
 ( 0.000000000000000000, 1.000000000000000000 ),
 .UNSPECIFIED. ) ;
#20926=CARTESIAN_POINT ( 'NONE',  ( -9.173272937381000247, -77.24698761531298885, 2.837265496132999942 ) ) ;
#20934=CARTESIAN_POINT ( 'NONE',  ( -1.329807244621280971, -79.13613989625301315, 9.426744174562156076 ) ) ;
#20935=CARTESIAN_POINT ( 'NONE',  ( -5.198192873473606035, -79.99999999999998579, -7.810577683091829648 ) ) ;
#20938=CARTESIAN_POINT ( 'NONE',  ( 4.128286005151000637, -78.98296321443997670, 8.744818112003999389 ) ) ;
#20953=CIRCLE ( 'NONE', #54927, 4.100000000000000533 ) ;
#20954=CARTESIAN_POINT ( 'NONE',  ( 3.176667715697470307, -79.80173575882605519, 10.50602662186070013 ) ) ;
#20957=EDGE_LOOP ( 'NONE', ( #36796, #45150, #13322, #1909, #51379 ) ) ;
#20969=DIRECTION ( 'NONE',  ( -1.000000000000000000, 0.000000000000000000, 0.000000000000000000 ) ) ;
#20972=CARTESIAN_POINT ( 'NONE',  ( 5.215253922439524459, -79.92783438175399624, 7.639483251372545247 ) ) ;
#20977=CARTESIAN_POINT ( 'NONE',  ( 9.478197642333000772, -79.91626286943099444, 6.090377947633999867 ) ) ;
#20978=CARTESIAN_POINT ( 'NONE',  ( 7.489645613629919652, -77.30016879572562516, -5.428330277087084710 ) ) ;
#20981=AXIS2_PLACEMENT_3D ( 'NONE', #51141, #46726, #5091 ) ;
#20989=CARTESIAN_POINT ( 'NONE',  ( 8.348568777154000031, -78.25112293168498923, -7.051780313135000533 ) ) ;
#21003=CARTESIAN_POINT ( 'NONE',  ( -6.351606481687999128, -78.07617171442198867, 7.094185741421999758 ) ) ;
#21014=CARTESIAN_POINT ( 'NONE',  ( -0.5193979750644999172, -78.99108129143698420, -10.96331347381999954 ) ) ;
#21016=CARTESIAN_POINT ( 'NONE',  ( -10.75651041663249607, -80.44348958333230826, 1.407171709692736083 ) ) ;
#21024=CARTESIAN_POINT ( 'NONE',  ( 9.249999999999996447, -78.23958333333334281, -1.210822168571094481 ) ) ;
#21025=CARTESIAN_POINT ( 'NONE',  ( -10.07307375010999984, -78.71614208009899016, -5.046000355766999235 ) ) ;
#21038=ORIENTED_EDGE ( 'NONE', *, *, #31373, .F. ) ;
#21041=VERTEX_POINT ( 'NONE', #5423 ) ;
#21042=VERTEX_POINT ( 'NONE', #6591 ) ;
#21049=ADVANCED_FACE ( 'NONE', ( #14567 ), #30866, .F. ) ;
#21052=CARTESIAN_POINT ( 'NONE',  ( -4.872763204610360610, -77.51918167194213538, 7.863451525103128503 ) ) ;
#21053=CARTESIAN_POINT ( 'NONE',  ( -9.808193611224998776, -77.77159370546399941, 5.067887917229000116 ) ) ;
#21056=CARTESIAN_POINT ( 'NONE',  ( -3.907230163516999699, -77.92217509810099330, -8.882807090995999744 ) ) ;
#21060=CARTESIAN_POINT ( 'NONE',  ( -4.017143116098000455, -80.27389229980698815, 10.51352533724000082 ) ) ;
#21062=CARTESIAN_POINT ( 'NONE',  ( 0.000000000000000000, -78.69999999999998863, 0.000000000000000000 ) ) ;
#21063=EDGE_LOOP ( 'NONE', ( #48000, #24281, #34613, #23870 ) ) ;
#21072=CARTESIAN_POINT ( 'NONE',  ( -8.182545292233999845, -80.43338938826599360, 7.620877899251000009 ) ) ;
#21089=EDGE_CURVE ( 'NONE', #8528, #47767, #19011, .T. ) ;
#21092=CARTESIAN_POINT ( 'NONE',  ( 1.918267526783000054, -77.23179811450799548, 10.77842959370000031 ) ) ;
#21097=CARTESIAN_POINT ( 'NONE',  ( 7.764258067048000811, -77.01038689586449948, 5.767450660628000492 ) ) ;
#21098=CARTESIAN_POINT ( 'NONE',  ( 7.396918292183172206, -78.30208333333331439, 5.684557159767955170 ) ) ;
#21107=VERTEX_POINT ( 'NONE', #52912 ) ;
#21110=ORIENTED_EDGE ( 'NONE', *, *, #56057, .T. ) ;
#21113=CIRCLE ( 'NONE', #13561, 10.69999999999999929 ) ;
#21116=ORIENTED_EDGE ( 'NONE', *, *, #12574, .F. ) ;
#21119=CARTESIAN_POINT ( 'NONE',  ( 7.396918292183175758, -79.69791666666667140, -5.684557159767951617 ) ) ;
#21121=FACE_OUTER_BOUND ( 'NONE', #45595, .T. ) ;
#21128=CARTESIAN_POINT ( 'NONE',  ( -3.592030622028691056, -77.25518602892395847, 8.980398724672147281 ) ) ;
#21130=CARTESIAN_POINT ( 'NONE',  ( -8.447183166110368902, -78.63346764869346828, -3.773792821381649620 ) ) ;
#21148=CARTESIAN_POINT ( 'NONE',  ( -10.96673197750000206, -78.31274657044698984, -0.4413686857046000278 ) ) ;
#21158=CARTESIAN_POINT ( 'NONE',  ( 6.852546780225999612, -78.64586191736599119, -6.611579150008999761 ) ) ;
#21164=CARTESIAN_POINT ( 'NONE',  ( 10.99999999999999822, -78.93958333333334565, -1.439896632895356188 ) ) ;
#21166=EDGE_CURVE ( 'NONE', #29378, #40036, #43174, .T. ) ;
#21168=CARTESIAN_POINT ( 'NONE',  ( 7.763360352781000451, -78.68303046778699184, 7.708310604078000061 ) ) ;
#21171=CARTESIAN_POINT ( 'NONE',  ( -7.101555135103000183, -80.37802629438799329, -8.827926690876999771 ) ) ;
#21172=ORIENTED_EDGE ( 'NONE', *, *, #7016, .T. ) ;
#21177=DIRECTION ( 'NONE',  ( 0.000000000000000000, -1.000000000000000000, 0.000000000000000000 ) ) ;
#21178=CARTESIAN_POINT ( 'NONE',  ( -7.479908383216000267, -79.68574476804501217, -6.281056869080000382 ) ) ;
#21180=ORIENTED_EDGE ( 'NONE', *, *, #43097, .F. ) ;
#21193=CARTESIAN_POINT ( 'NONE',  ( 8.823651773949475086, -78.82575552834812527, -2.782417521243436109 ) ) ;
#21198=CARTESIAN_POINT ( 'NONE',  ( 1.439896632895286466, -77.96458333333332291, 11.00000000000000711 ) ) ;
#21201=DIRECTION ( 'NONE',  ( 1.000000000000000000, 0.000000000000000000, 0.000000000000000000 ) ) ;
#21203=CARTESIAN_POINT ( 'NONE',  ( -2.794222306786000143, -77.12148308212269399, -8.839119250891998902 ) ) ;
#21218=CARTESIAN_POINT ( 'NONE',  ( -9.509637957782862472, -79.24022236790916907, 1.167149435952707259 ) ) ;
#21221=CARTESIAN_POINT ( 'NONE',  ( -6.977995179411893290, -79.99999999999998579, -6.220662632887979271 ) ) ;
#21224=CARTESIAN_POINT ( 'NONE',  ( 1.497466954355000102, -79.56970617083499064, 9.665433974424999519 ) ) ;
#21226=CARTESIAN_POINT ( 'NONE',  ( -4.658475568430814562, -79.08333333333332860, -8.082524092276884176 ) ) ;
#21227=VERTEX_POINT ( 'NONE', #47351 ) ;
#21229=AXIS2_PLACEMENT_3D ( 'NONE', #49548, #48664, #26211 ) ;
#21234=VECTOR ( 'NONE', #48863, 1000.000000000000114 ) ;
#21238=CARTESIAN_POINT ( 'NONE',  ( -4.670305506034999610, -77.01883941971439640, -9.783521845360001024 ) ) ;
#21240=DIRECTION ( 'NONE',  ( -1.000000000000000000, 0.000000000000000000, 0.000000000000000000 ) ) ;
#21242=CARTESIAN_POINT ( 'NONE',  ( -9.358268528169000788, -79.23265764587299032, -2.797054701638000296 ) ) ;
#21244=VERTEX_POINT ( 'NONE', #20751 ) ;
#21259=CARTESIAN_POINT ( 'NONE',  ( -1.037716418681747577, -79.98405221576109625, 9.192368781140272560 ) ) ;
#21263=CARTESIAN_POINT ( 'NONE',  ( 9.101894997447999458, -78.82066105045699089, -6.639611571546000235 ) ) ;
#21264=CARTESIAN_POINT ( 'NONE',  ( 4.311764069688931222, -77.26360251928231548, -8.183661215609575379 ) ) ;
#21273=CARTESIAN_POINT ( 'NONE',  ( -10.99582742793000101, -79.54337123098800078, 1.892981466416000069 ) ) ;
#21277=CYLINDRICAL_SURFACE ( 'NONE', #28524, 9.250000000000000000 ) ;
#21280=CARTESIAN_POINT ( 'NONE',  ( -7.330094131514235833, -77.20000000000001705, 8.056329451334999447 ) ) ;
#21288=CARTESIAN_POINT ( 'NONE',  ( -7.476203163627999970, -77.13115727064058547, -5.719923538308999689 ) ) ;
#21300=CARTESIAN_POINT ( 'NONE',  ( 10.55657102546000026, -78.59778833077898241, -3.003801718854000047 ) ) ;
#21304=LINE ( 'NONE', #15723, #10771 ) ;
#21307=CARTESIAN_POINT ( 'NONE',  ( 4.213602390902059902, -77.33743496812297735, 8.266346695140056156 ) ) ;
#21310=CARTESIAN_POINT ( 'NONE',  ( -9.757422770562000025, -79.13752739508899481, 5.632196307135999724 ) ) ;
#21312=DIRECTION ( 'NONE',  ( 0.000000000000000000, 1.000000000000000000, 0.000000000000000000 ) ) ;
#21323=ORIENTED_EDGE ( 'NONE', *, *, #37170, .T. ) ;
#21335=CARTESIAN_POINT ( 'NONE',  ( -5.453704473740694780, -77.52520987146617415, 7.471219652258522359 ) ) ;
#21340=CARTESIAN_POINT ( 'NONE',  ( 9.703485699160999900, -77.58108914855399973, 0.1143444355825999903 ) ) ;
#21344=CARTESIAN_POINT ( 'NONE',  ( -1.635010352784000087, -80.48269812649999722, -10.62493487727000030 ) ) ;
#21346=PLANE ( 'NONE',  #49708 ) ;
#21354=CARTESIAN_POINT ( 'NONE',  ( 4.635796264669566291, -79.43347470810225275, 8.027154431640754595 ) ) ;
#21359=CONICAL_SURFACE ( 'NONE', #41173, 10.80312499997999964, 0.7853981633972997312 ) ;
#21360=ORIENTED_EDGE ( 'NONE', *, *, #41212, .T. ) ;
#21367=CARTESIAN_POINT ( 'NONE',  ( -3.818323177486000031, -79.42900767078099022, 8.616648607789999303 ) ) ;
#21373=CARTESIAN_POINT ( 'NONE',  ( 9.611650271896843734, -77.40833333333328881, -5.539808784079876425 ) ) ;
#21381=CARTESIAN_POINT ( 'NONE',  ( 9.670530767802999250, -76.95816816192808574, -0.1674091926992999912 ) ) ;
#21417=DIRECTION ( 'NONE',  ( 1.000000000000000000, 0.000000000000000000, 0.000000000000000000 ) ) ;
#21418=B_SPLINE_CURVE_WITH_KNOTS ( 'NONE', 3,
 ( #327, #17718, #4725, #14148, #40736, #23015, #31261, #617, #28012, #29, #45765, #18305, #35702, #18600, #36589 ),
 .UNSPECIFIED., .F., .F.,
 ( 4, 1, 1, 1, 1, 1, 1, 1, 1, 1, 1, 1, 4 ),
 ( 0.000000000000000000, 0.05991653944398223075, 0.1464624072683559930, 0.2330082750926717738, 0.3195541429170455361, 0.4061000107414192706, 0.4926458785657931161, 0.5791917463901669061, 0.6657376142143087705, 0.7522834820388564214, 0.8388293498634040724, 0.9253752176879519453, 1.000000000000000000 ),
 .UNSPECIFIED. ) ;
#21439=CARTESIAN_POINT ( 'NONE',  ( -11.00000000000000000, -79.69999999999998863, 0.000000000000000000 ) ) ;
#21449=CARTESIAN_POINT ( 'NONE',  ( -0.1527179957142000277, -78.26932405616399535, 9.629635879864999026 ) ) ;
#21460=ORIENTED_EDGE ( 'NONE', *, *, #52626, .T. ) ;
#21461=CARTESIAN_POINT ( 'NONE',  ( -10.62234821842000088, -78.85158459378298801, 2.617925641156000349 ) ) ;
#21463=DIRECTION ( 'NONE',  ( 0.000000000000000000, 0.000000000000000000, -1.000000000000000000 ) ) ;
#21464=ORIENTED_EDGE ( 'NONE', *, *, #46109, .T. ) ;
#21470=CARTESIAN_POINT ( 'NONE',  ( 0.000000000000000000, -74.64999999999999147, 0.000000000000000000 ) ) ;
#21481=EDGE_CURVE ( 'NONE', #4986, #25253, #1237, .T. ) ;
#21490=CARTESIAN_POINT ( 'NONE',  ( 11.00000000000000000, -77.84999999999999432, 0.000000000000000000 ) ) ;
#21496=CARTESIAN_POINT ( 'NONE',  ( 2.265947762240999808, -77.10112295295309082, -9.216051757218000517 ) ) ;
#21506=ORIENTED_EDGE ( 'NONE', *, *, #1465, .F. ) ;
#21510=CARTESIAN_POINT ( 'NONE',  ( -4.833288342901160384, -79.16736403866717353, 8.201749509104971025 ) ) ;
#21511=DIRECTION ( 'NONE',  ( 0.000000000000000000, -1.000000000000000000, 0.000000000000000000 ) ) ;
#21512=CARTESIAN_POINT ( 'NONE',  ( -8.796335266380006956, -79.04791666666669414, 6.760013919724027431 ) ) ;
#21514=CARTESIAN_POINT ( 'NONE',  ( -7.948284285155000184, -79.75644446212498906, -5.699806846671999772 ) ) ;
#21520=VECTOR ( 'NONE', #34645, 1000.000000000000000 ) ;
#21533=CARTESIAN_POINT ( 'NONE',  ( -8.448510849392999233, -79.28831818069899384, 4.901364000006999788 ) ) ;
#21534=ORIENTED_EDGE ( 'NONE', *, *, #23830, .T. ) ;
#21544=PRODUCT_DEFINITION_CONTEXT ( 'detailed design', #8898, 'design' ) ;
#21553=CARTESIAN_POINT ( 'NONE',  ( -7.208482872893000604, -79.55106226310599027, 8.658331769851001170 ) ) ;
#21554=CARTESIAN_POINT ( 'NONE',  ( 9.249971803402324610, -77.34340569116132258, -0.7721083477804356887 ) ) ;
#21562=CARTESIAN_POINT ( 'NONE',  ( 0.000000000000000000, -75.09999999979599750, -4.899999999795999983 ) ) ;
#21564=CARTESIAN_POINT ( 'NONE',  ( -9.242272388666000538, -79.00961649866798098, 6.250760013846000440 ) ) ;
#21573=CARTESIAN_POINT ( 'NONE',  ( 9.249827694200002171, -79.25056085624731850, 0.06519332901358350363 ) ) ;
#21588=CARTESIAN_POINT ( 'NONE',  ( 10.71556987377000070, -79.69750836675898142, 2.374990294079000197 ) ) ;
#21598=CARTESIAN_POINT ( 'NONE',  ( 2.879226727952094222, -77.74583333333333712, -10.71369944335146940 ) ) ;
#21600=CARTESIAN_POINT ( 'NONE',  ( 7.338671297540000360, -79.06094136420898622, 8.404493039061998516 ) ) ;
#21602=DIRECTION ( 'NONE',  ( 0.000000000000000000, 1.000000000000000000, 0.000000000000000000 ) ) ;
#21613=CARTESIAN_POINT ( 'NONE',  ( -3.359581381603320871, -79.84641223401524712, -8.956518138560074505 ) ) ;
#21617=AXIS2_PLACEMENT_3D ( 'NONE', #46488, #46783, #6012 ) ;
#21620=CARTESIAN_POINT ( 'NONE',  ( -6.539419588528526894, -78.16268753938295788, -6.541902902125212194 ) ) ;
#21623=ADVANCED_FACE ( 'NONE', ( #33659 ), #11819, .T. ) ;
#21625=CARTESIAN_POINT ( 'NONE',  ( -4.757657419345691530, -77.51803282916795013, 7.934074630878104273 ) ) ;
#21628=CARTESIAN_POINT ( 'NONE',  ( 7.658860137760000519, -78.63277082632598081, 5.959242465009999989 ) ) ;
#21632=CARTESIAN_POINT ( 'NONE',  ( -8.744140569415000286, -80.25535053947399433, 7.086030162020000134 ) ) ;
#21636=CARTESIAN_POINT ( 'NONE',  ( -9.009247259181922374, -78.52083333333334281, -2.421167930323344653 ) ) ;
#21649=CARTESIAN_POINT ( 'NONE',  ( 10.99999999999999822, -79.96041666666779690, 1.439896632895345086 ) ) ;
#21691=CARTESIAN_POINT ( 'NONE',  ( 10.36935812844000004, -78.07876026662599145, -2.835297515976000327 ) ) ;
#21695=DIRECTION ( 'NONE',  ( 0.000000000000000000, 1.000000000000000000, 0.000000000000000000 ) ) ;
#21700=CARTESIAN_POINT ( 'NONE',  ( -9.312149464823921363, -77.13785053516166101, -0.06563382585331917207 ) ) ;
#21707=ADVANCED_FACE ( 'NONE', ( #7956 ), #53548, .T. ) ;
#21708=CARTESIAN_POINT ( 'NONE',  ( -8.719367347793284040, -78.62710504220744667, -3.087874295618068476 ) ) ;
#21713=CARTESIAN_POINT ( 'NONE',  ( -9.469606800734000629, -79.65752053325199711, 5.597012331546999953 ) ) ;
#21715=LINE ( 'NONE', #13139, #22183 ) ;
#21717=CARTESIAN_POINT ( 'NONE',  ( 10.75503897980323309, -77.20000000000001705, -0.4084248854891507352 ) ) ;
#21727=ORIENTED_EDGE ( 'NONE', *, *, #9620, .T. ) ;
#21728=CARTESIAN_POINT ( 'NONE',  ( 0.000000000000000000, -74.64999999999999147, 0.000000000000000000 ) ) ;
#21732=CARTESIAN_POINT ( 'NONE',  ( 7.201320854070999644, -77.70084747358500010, 6.394856364399000626 ) ) ;
#21738=DIRECTION ( 'NONE',  ( 3.342393029126999711E-11, -1.000000000000000000, 3.127660138207999783E-09 ) ) ;
#21739=CARTESIAN_POINT ( 'NONE',  ( 11.00000000000000000, -78.94999999999998863, -1.064824513673000067E-14 ) ) ;
#21745=CARTESIAN_POINT ( 'NONE',  ( 10.82226978776999893, -79.13250813710999410, 1.601965348215999896 ) ) ;
#21747=CARTESIAN_POINT ( 'NONE',  ( -10.67332088312999971, -80.27238938826599224, -4.121781213195999882 ) ) ;
#21750=ORIENTED_EDGE ( 'NONE', *, *, #54901, .T. ) ;
#21753=VERTEX_POINT ( 'NONE', #13181 ) ;
#21755=ORIENTED_EDGE ( 'NONE', *, *, #37094, .T. ) ;
#21766=DIRECTION ( 'NONE',  ( 0.000000000000000000, 1.000000000000000000, 0.000000000000000000 ) ) ;
#21770=CIRCLE ( 'NONE', #6750, 1.000000000000000000 ) ;
#21775=CARTESIAN_POINT ( 'NONE',  ( 0.5437984056370208652, -79.97105364439701702, 11.05137384886682916 ) ) ;
#21779=CARTESIAN_POINT ( 'NONE',  ( 8.827998080066999265, -77.24332679464099272, -3.176622877762000030 ) ) ;
#21798=CARTESIAN_POINT ( 'NONE',  ( 7.637074688270999445, -78.94561555618199122, 5.932176574774000066 ) ) ;
#21819=CARTESIAN_POINT ( 'NONE',  ( 9.226480760116999136, -79.00070664722298375, -2.263195259622999611 ) ) ;
#21826=CARTESIAN_POINT ( 'NONE',  ( -5.159130208082606472, -77.43030033517193544, -8.219319990131634057 ) ) ;
#21832=CARTESIAN_POINT ( 'NONE',  ( 3.393132750703385270, -79.94520027180968214, 8.605390363453048863 ) ) ;
#21836=CARTESIAN_POINT ( 'NONE',  ( 10.24618685648000138, -78.90493811345498898, 4.684505231889000143 ) ) ;
#21837=CARTESIAN_POINT ( 'NONE',  ( -2.699182493562976681, -77.20154682869322471, -8.848940700691480643 ) ) ;
#21843=CARTESIAN_POINT ( 'NONE',  ( -10.75000000000000000, -80.44999999999998863, 5.225043809877999334E-10 ) ) ;
#21844=CARTESIAN_POINT ( 'NONE',  ( 8.456503675551001464, -78.36349234901598493, 7.278678959607000287 ) ) ;
#21855=CARTESIAN_POINT ( 'NONE',  ( -9.397813699260852971, -80.00762368868254271, 5.554579860211124931 ) ) ;
#21859=CARTESIAN_POINT ( 'NONE',  ( -4.441436338936000539, -78.79379552517198704, -8.545575054271999704 ) ) ;
#21866=CARTESIAN_POINT ( 'NONE',  ( 9.009247259181915268, -78.77083333333334281, 2.421167930323361972 ) ) ;
#21871=CARTESIAN_POINT ( 'NONE',  ( 9.632126701410999914, -79.21993834310299576, 5.261763182588000021 ) ) ;
#21872=CARTESIAN_POINT ( 'NONE',  ( 6.673790874065899104, -80.33932291666529579, 8.685525953824821954 ) ) ;
#21874=CARTESIAN_POINT ( 'NONE',  ( -9.469606800734000629, -79.65752053325199711, 5.597012331546999953 ) ) ;
#21879=CARTESIAN_POINT ( 'NONE',  ( 10.71369944335147473, -77.82916666666666572, -2.879226727952063580 ) ) ;
#21881=CARTESIAN_POINT ( 'NONE',  ( 9.386754667005000385, -79.53851138786500030, 6.031619700400000283 ) ) ;
#21883=DIRECTION ( 'NONE',  ( 0.000000000000000000, 1.000000000000000000, 0.000000000000000000 ) ) ;
#21888=EDGE_CURVE ( 'NONE', #33386, #20388, #25168, .T. ) ;
#21900=CARTESIAN_POINT ( 'NONE',  ( -6.395610860418600829, -78.16440346101558134, -6.682817714148057142 ) ) ;
#21906=CARTESIAN_POINT ( 'NONE',  ( -0.2651902714627518143, -77.47745245132422554, 9.246255095149187753 ) ) ;
#21907=CARTESIAN_POINT ( 'NONE',  ( 2.604371601988999974, -77.45349661881098768, -10.72853197743999942 ) ) ;
#21909=CARTESIAN_POINT ( 'NONE',  ( -5.351292223237999579, -77.81193504899798086, 8.095330809056001442 ) ) ;
#21914=CARTESIAN_POINT ( 'NONE',  ( -9.459258931978000717, -79.82843986952799753, 5.442530770145999952 ) ) ;
#21924=CARTESIAN_POINT ( 'NONE',  ( -2.420948490244752449, -78.49585695048426714, 9.008675488125174269 ) ) ;
#21931=CARTESIAN_POINT ( 'NONE',  ( -10.99999999999000089, -80.20000000002698926, -2.639066790267999940E-09 ) ) ;
#21932=EDGE_LOOP ( 'NONE', ( #41224, #42831, #39045, #15813, #40746, #57038, #5569 ) ) ;
#21937=CARTESIAN_POINT ( 'NONE',  ( -0.08960567475284000882, -79.89657020290799494, 9.424340550334999733 ) ) ;
#21940=CARTESIAN_POINT ( 'NONE',  ( 5.399973277016593798, -77.19999999999998863, 9.364213316283096944 ) ) ;
#21945=EDGE_CURVE ( 'NONE', #24388, #21041, #54233, .T. ) ;
#21951=CARTESIAN_POINT ( 'NONE',  ( 2.632967082928999947, -77.18321148114229402, 9.306700570505000769 ) ) ;
#21969=ORIENTED_EDGE ( 'NONE', *, *, #57125, .F. ) ;
#21977=CARTESIAN_POINT ( 'NONE',  ( -10.79754810891999917, -77.36671284630264722, -2.301543980132999767 ) ) ;
#21979=ORIENTED_EDGE ( 'NONE', *, *, #48239, .F. ) ;
#21986=CARTESIAN_POINT ( 'NONE',  ( 9.690463944985998168, -78.45531731672599562, -0.5153813127049999832 ) ) ;
#21993=CARTESIAN_POINT ( 'NONE',  ( -9.216383265370728495, -78.60684264245168151, -0.7874879489689852186 ) ) ;
#22016=CARTESIAN_POINT ( 'NONE',  ( 1.975443078346000192, -77.04017089215798819, 11.09968961003999866 ) ) ;
#22020=CARTESIAN_POINT ( 'NONE',  ( -6.639445101857000431, -78.02053767652898841, -6.825550891425999467 ) ) ;
#22030=CARTESIAN_POINT ( 'NONE',  ( -10.53745838584999994, -79.85354523164899376, 2.317267403318000074 ) ) ;
#22034=CARTESIAN_POINT ( 'NONE',  ( 8.837556037038000412, -79.93830006555698731, -7.266664171576000086 ) ) ;
#22052=CARTESIAN_POINT ( 'NONE',  ( 8.872594700925422018, -78.82720320433729455, -2.619895919442627008 ) ) ;
#22060=FACE_OUTER_BOUND ( 'NONE', #7356, .T. ) ;
#22072=DIRECTION ( 'NONE',  ( 0.000000000000000000, 0.000000000000000000, -1.000000000000000000 ) ) ;
#22083=CARTESIAN_POINT ( 'NONE',  ( 8.584722543520001636, -79.11501084750798896, 4.148835967969999317 ) ) ;
#22085=CARTESIAN_POINT ( 'NONE',  ( 5.850913721802999845, -79.38296787954499223, -7.837718406031999763 ) ) ;
#22108=CARTESIAN_POINT ( 'NONE',  ( 6.653382217586999658, -79.58521449586598351, 7.150748904218000135 ) ) ;
#22116=CARTESIAN_POINT ( 'NONE',  ( 5.091979538295729135, -78.68094881684694997, 8.261087832219587312 ) ) ;
#22117=EDGE_CURVE ( 'NONE', #3901, #22275, #34524, .T. ) ;
#22124=CARTESIAN_POINT ( 'NONE',  ( 5.428802703023839271, -79.92556352659003949, 7.489012433513578593 ) ) ;
#22126=ORIENTED_EDGE ( 'NONE', *, *, #32128, .T. ) ;
#22127=CARTESIAN_POINT ( 'NONE',  ( -9.757422770562000025, -79.57915461743898788, 5.632196307135999724 ) ) ;
#22153=CARTESIAN_POINT ( 'NONE',  ( 4.459991035765999534, -77.47927130271399676, 8.413017068390001185 ) ) ;
#22165=CARTESIAN_POINT ( 'NONE',  ( -9.438868967565998247, -79.47276953209699002, -5.601050722391000214 ) ) ;
#22166=CARTESIAN_POINT ( 'NONE',  ( -10.75000000000000000, -80.44999999999998863, 5.225043809877999334E-10 ) ) ;
#22175=CARTESIAN_POINT ( 'NONE',  ( -11.08844420678000020, -78.75192546654999148, -1.240163186867999867 ) ) ;
#22183=VECTOR ( 'NONE', #31132, 1000.000000000000000 ) ;
#22197=CARTESIAN_POINT ( 'NONE',  ( -9.022067442310994778, -78.11871138684033156, -2.130921441519212145 ) ) ;
#22202=CARTESIAN_POINT ( 'NONE',  ( -0.09048081827621948237, -77.47593987896340195, 9.249522775818471487 ) ) ;
#22203=CARTESIAN_POINT ( 'NONE',  ( 10.77519778174000109, -77.17117949372459407, -1.228540277667999892 ) ) ;
#22205=CARTESIAN_POINT ( 'NONE',  ( 9.259046916275000427, -78.66464992286799429, 2.905298533503999803 ) ) ;
#22229=DIRECTION ( 'NONE',  ( 0.000000000000000000, 1.000000000000000000, 0.000000000000000000 ) ) ;
#22235=CARTESIAN_POINT ( 'NONE',  ( -8.608637500484000782, -79.48745298729599540, 3.836350400429999752 ) ) ;
#22237=CARTESIAN_POINT ( 'NONE',  ( 9.408852130907261468, -77.30624999999999147, -5.763669873574839286 ) ) ;
#22249=CARTESIAN_POINT ( 'NONE',  ( 7.764258067048000811, -77.19129567287669147, 5.767450660628000492 ) ) ;
#22253=DIRECTION ( 'NONE',  ( 0.000000000000000000, -0.7071067811866525998, -0.7071067811864425456 ) ) ;
#22256=CARTESIAN_POINT ( 'NONE',  ( 9.611650271896843734, -79.39166666666663730, 5.539808784079872872 ) ) ;
#22263=SURFACE_STYLE_FILL_AREA ( #13402 ) ;
#22272=ORIENTED_EDGE ( 'NONE', *, *, #58090, .F. ) ;
#22275=VERTEX_POINT ( 'NONE', #42484 ) ;
#22278=AXIS2_PLACEMENT_3D ( 'NONE', #58397, #32102, #49554 ) ;
#22280=CARTESIAN_POINT ( 'NONE',  ( -5.681372509047000641, -78.28477434195299622, -7.867192369580999767 ) ) ;
#22283=AXIS2_PLACEMENT_3D ( 'NONE', #8434, #32028, #18475 ) ;
#22290=CARTESIAN_POINT ( 'NONE',  ( -5.088691759813757095E-08, -76.94999999999998863, -9.499908983443795307 ) ) ;
#22300=ORIENTED_EDGE ( 'NONE', *, *, #11460, .T. ) ;
#22301=CARTESIAN_POINT ( 'NONE',  ( 11.00000000000000000, -78.44999999999998863, 0.000000000000000000 ) ) ;
#22311=CARTESIAN_POINT ( 'NONE',  ( -10.73206714754000046, -77.15440972681939513, 3.453790258818999703 ) ) ;
#22314=CARTESIAN_POINT ( 'NONE',  ( 1.459128634122999868, -77.59418023959399591, -9.409639786240999726 ) ) ;
#22339=CARTESIAN_POINT ( 'NONE',  ( 8.944729675425000082, -80.03290621929455995, 3.923329690209000908 ) ) ;
#22348=EDGE_CURVE ( 'NONE', #55096, #11974, #29174, .T. ) ;
#22353=DIRECTION ( 'NONE',  ( 0.000000000000000000, -1.000000000000000000, 0.000000000000000000 ) ) ;
#22355=CARTESIAN_POINT ( 'NONE',  ( 1.439896632895286466, -78.46458333333332291, 11.00000000000000711 ) ) ;
#22363=CARTESIAN_POINT ( 'NONE',  ( -1.454020682123249530, -80.00000000000000000, 9.185157777585660099 ) ) ;
#22367=VECTOR ( 'NONE', #52984, 1000.000000000000000 ) ;
#22378=CARTESIAN_POINT ( 'NONE',  ( -11.00000000000000000, -78.19999999999998863, 0.000000000000000000 ) ) ;
#22380=ORIENTED_EDGE ( 'NONE', *, *, #24024, .F. ) ;
#22399=EDGE_LOOP ( 'NONE', ( #53870, #50560, #36642, #40832, #48003 ) ) ;
#22408=CARTESIAN_POINT ( 'NONE',  ( -7.545891804452000251, -79.77540805456798978, 6.201630566990999682 ) ) ;
#22423=CARTESIAN_POINT ( 'NONE',  ( 8.230920277480567648, -79.88818024824762176, 4.220077749870753792 ) ) ;
#22424=CARTESIAN_POINT ( 'NONE',  ( -5.016174693291526765, -80.03806740382935914, -9.911088353662746542 ) ) ;
#22432=DIRECTION ( 'NONE',  ( 0.000000000000000000, 0.000000000000000000, -1.000000000000000000 ) ) ;
#22450=CARTESIAN_POINT ( 'NONE',  ( -9.108272167377998940, -77.16660918229489141, -2.776672910959999907 ) ) ;
#22460=CARTESIAN_POINT ( 'NONE',  ( 3.303001513109999898, -79.07947657143998299, -10.46681410869999951 ) ) ;
#22461=CARTESIAN_POINT ( 'NONE',  ( 10.99999999999999645, -79.33958333333332291, -1.439896632895355522 ) ) ;
#22465=ORIENTED_EDGE ( 'NONE', *, *, #54547, .F. ) ;
#22472=B_SPLINE_CURVE_WITH_KNOTS ( 'NONE', 3,
 ( #31601, #57900, #8310, #49644 ),
 .UNSPECIFIED., .F., .F.,
 ( 4, 4 ),
 ( 0.000000000000000000, 1.000000000000000000 ),
 .UNSPECIFIED. ) ;
#22473=CARTESIAN_POINT ( 'NONE',  ( 9.088959790636000236, -78.01048704979598369, -6.010253266999000310 ) ) ;
#22478=CARTESIAN_POINT ( 'NONE',  ( -9.250000000000007105, -79.98958333333334281, 1.210822168571027868 ) ) ;
#22480=CARTESIAN_POINT ( 'NONE',  ( -8.861449449424648961, -79.64887384436650564, 6.625956105248707928 ) ) ;
#22483=EDGE_LOOP ( 'NONE', ( #50900, #51266, #38025, #6195 ) ) ;
#22485=DIRECTION ( 'NONE',  ( 0.000000000000000000, -1.000000000000000000, 0.000000000000000000 ) ) ;
#22488=CARTESIAN_POINT ( 'NONE',  ( 8.926771828799410002, -79.52861684990361368, 3.353330014368605561 ) ) ;
#22491=CIRCLE ( 'NONE', #33820, 4.799999999999999822 ) ;
#22493=CARTESIAN_POINT ( 'NONE',  ( -8.082524092276882399, -79.54166666666665719, -4.658475568430820779 ) ) ;
#22495=CARTESIAN_POINT ( 'NONE',  ( -9.250000000000000000, -78.09999999999999432, 0.000000000000000000 ) ) ;
#22500=EDGE_CURVE ( 'NONE', #3819, #21753, #37356, .T. ) ;
#22501=CARTESIAN_POINT ( 'NONE',  ( 6.073699447519306460, -77.41819971103011255, 6.993117814290229717 ) ) ;
#22502=CARTESIAN_POINT ( 'NONE',  ( -0.5413127449341000874, -77.99094517446199859, -11.02683867434999954 ) ) ;
#22505=CARTESIAN_POINT ( 'NONE',  ( 9.662203867310999783, -79.14785501805998535, 0.9012207007054000574 ) ) ;
#22522=CARTESIAN_POINT ( 'NONE',  ( 10.52982398497215577, -78.27927571967974529, -2.879177815852805633 ) ) ;
#22525=CARTESIAN_POINT ( 'NONE',  ( -8.263041386619001116, -80.49726512904899778, 7.695848569717000487 ) ) ;
#22559=CARTESIAN_POINT ( 'NONE',  ( -1.439896632895332207, -79.48541666666665151, 10.99999999999999822 ) ) ;
#22569=CARTESIAN_POINT ( 'NONE',  ( -9.254388464354001087, -79.80752053325198858, 5.469807505829999528 ) ) ;
#22574=CARTESIAN_POINT ( 'NONE',  ( -9.050627908548998235, -77.39852255496806777, -6.322205650057998838 ) ) ;
#22578=ORIENTED_EDGE ( 'NONE', *, *, #30223, .F. ) ;
#22581=CARTESIAN_POINT ( 'NONE',  ( -7.456816947376000648, -78.65428412062898644, 6.210200510404999541 ) ) ;
#22582=AXIS2_PLACEMENT_3D ( 'NONE', #12787, #22229, #44679 ) ;
#22588=CARTESIAN_POINT ( 'NONE',  ( -2.935661446561999899, -76.94999999999998863, -9.035036904803998681 ) ) ;
#22598=DIRECTION ( 'NONE',  ( 1.000000000000000000, 0.000000000000000000, 0.000000000000000000 ) ) ;
#22617=CARTESIAN_POINT ( 'NONE',  ( 2.813750093493999849, -78.10580916391599260, -9.096877851405000825 ) ) ;
#22627=ORIENTED_EDGE ( 'NONE', *, *, #36437, .F. ) ;
#22642=CARTESIAN_POINT ( 'NONE',  ( 8.985706068735000329, -79.96796090277857161, -3.828549499589000149 ) ) ;
#22646=CARTESIAN_POINT ( 'NONE',  ( 9.008013791555782745, -79.32919974289639242, -2.421050323904322177 ) ) ;
#22650=CARTESIAN_POINT ( 'NONE',  ( 0.9999999970599000587, -81.20000000293998710, -6.999999982650000341 ) ) ;
#22653=CARTESIAN_POINT ( 'NONE',  ( 0.002314721400742156526, -78.72516494628735018, -9.249912767016533977 ) ) ;
#22654=CARTESIAN_POINT ( 'NONE',  ( 0.000000000000000000, -81.99999999999998579, 0.000000000000000000 ) ) ;
#22658=CARTESIAN_POINT ( 'NONE',  ( 8.954446855713042552, -77.82933363352677247, -2.398406063174361336 ) ) ;
#22668=CARTESIAN_POINT ( 'NONE',  ( 8.954706589602396960, -79.82963375756635571, -2.398204254170784200 ) ) ;
#22671=CARTESIAN_POINT ( 'NONE',  ( 9.250000000000000000, -78.74999999999998579, 0.000000000000000000 ) ) ;
#22672=DIRECTION ( 'NONE',  ( 0.000000000000000000, -1.000000000000000000, 0.000000000000000000 ) ) ;
#22676=CARTESIAN_POINT ( 'NONE',  ( -4.043136777828877371, -78.19531677776082290, -10.31450538517581883 ) ) ;
#22686=CARTESIAN_POINT ( 'NONE',  ( 4.202230864774000096, -78.48968660667100039, -8.786407198941001084 ) ) ;
#22695=EDGE_CURVE ( 'NONE', #31318, #17717, #26666, .T. ) ;
#22698=CARTESIAN_POINT ( 'NONE',  ( 0.000000000000000000, -81.10000000285099020, 7.000000000000000000 ) ) ;
#22706=CARTESIAN_POINT ( 'NONE',  ( -7.479908383216000267, -79.38573615547299767, -6.281056869080000382 ) ) ;
#22714=AXIS2_PLACEMENT_3D ( 'NONE', #44492, #40055, #31182 ) ;
#22719=CARTESIAN_POINT ( 'NONE',  ( -4.814859605045999302, -78.66631515532277774, 8.425427962446999430 ) ) ;
#22720=CARTESIAN_POINT ( 'NONE',  ( 5.435707952731398507, -79.92548822285989729, 7.484002565572681398 ) ) ;
#22724=CARTESIAN_POINT ( 'NONE',  ( 2.868090520736068516, -77.25025914830622753, -8.794003640997004823 ) ) ;
#22731=CARTESIAN_POINT ( 'NONE',  ( 0.000000000000000000, -76.89999999999999147, -9.549999999999952749 ) ) ;
#22745=CARTESIAN_POINT ( 'NONE',  ( 9.078688998878000405, -79.04716346014799910, 3.126726393672000004 ) ) ;
#22754=CARTESIAN_POINT ( 'NONE',  ( -0.5193979750644999172, -79.05138421710698537, -10.96331347381999954 ) ) ;
#22766=CARTESIAN_POINT ( 'NONE',  ( 0.9241086513771999966, -78.61146369488598395, 11.11924560648999893 ) ) ;
#22770=CARTESIAN_POINT ( 'NONE',  ( 7.396918292183153554, -79.80208333333332860, 5.684557159767984480 ) ) ;
#22771=CARTESIAN_POINT ( 'NONE',  ( -3.023821996898441000, -79.59699371105349996, 10.64354645710085201 ) ) ;
#22777=STYLED_ITEM ( 'NONE', ( #55604 ), #42678 ) ;
#22785=CARTESIAN_POINT ( 'NONE',  ( 9.009247259181924150, -79.72916666666665719, -2.421167930323326001 ) ) ;
#22787=CARTESIAN_POINT ( 'NONE',  ( -5.757354885052930804, -78.17157179074094131, -7.240009484917052873 ) ) ;
#22793=CARTESIAN_POINT ( 'NONE',  ( 1.801927416992543218, -77.45946252748643701, 9.073133184625993053 ) ) ;
#22794=CARTESIAN_POINT ( 'NONE',  ( -1.996894868142000012, -77.37992772649998585, 10.85801781015000067 ) ) ;
#22797=VECTOR ( 'NONE', #27111, 1000.000000000000000 ) ;
#22798=CARTESIAN_POINT ( 'NONE',  ( 8.553489385229999797, -79.17627884718898201, 4.133741566275999979 ) ) ;
#22803=CARTESIAN_POINT ( 'NONE',  ( 0.1286847231337999997, -79.30325033209098251, 10.93943584368999922 ) ) ;
#22814=CARTESIAN_POINT ( 'NONE',  ( 0.000000000000000000, -81.99999999999998579, 0.000000000000000000 ) ) ;
#22827=CARTESIAN_POINT ( 'NONE',  ( -6.760013919724056741, -79.77291666666666003, -8.796335266379987416 ) ) ;
#22830=CARTESIAN_POINT ( 'NONE',  ( -10.69999999999999929, -76.39999999999999147, 0.000000000000000000 ) ) ;
#22839=CARTESIAN_POINT ( 'NONE',  ( -8.324924863653999196, -77.34795187468598954, 4.923709561474999497 ) ) ;
#22840=CARTESIAN_POINT ( 'NONE',  ( 9.250000000000000000, -78.24999999999998579, -1.152201742116999973E-14 ) ) ;
#22853=EDGE_CURVE ( 'NONE', #31523, #55944, #55303, .T. ) ;
#22866=CARTESIAN_POINT ( 'NONE',  ( 7.528714304400998536, -78.03471672827505756, -8.074838600060001426 ) ) ;
#22869=ORIENTED_EDGE ( 'NONE', *, *, #27165, .T. ) ;
#22872=CARTESIAN_POINT ( 'NONE',  ( 9.512131559252001267, -77.94368839240499369, -1.920953556448999899 ) ) ;
#22890=CARTESIAN_POINT ( 'NONE',  ( -1.704234056905189032, -77.20000000000001705, -10.88120482596699468 ) ) ;
#22895=CARTESIAN_POINT ( 'NONE',  ( -9.611650271896834852, -79.24166666666666003, -5.539808784079895965 ) ) ;
#22896=CARTESIAN_POINT ( 'NONE',  ( -11.00000000000000000, -78.69999999999998863, 0.000000000000000000 ) ) ;
#22909=CARTESIAN_POINT ( 'NONE',  ( -8.883074525067000238, -78.99397594943899037, 3.114832498031999908 ) ) ;
#22927=ORIENTED_EDGE ( 'NONE', *, *, #1079, .T. ) ;
#22947=CARTESIAN_POINT ( 'NONE',  ( -1.239656168602880193, -78.71434633308196283, -9.167881758628666944 ) ) ;
#22951=CARTESIAN_POINT ( 'NONE',  ( 0.000000000000000000, -76.19999999999998863, 0.000000000000000000 ) ) ;
#22968=CARTESIAN_POINT ( 'NONE',  ( -9.781286103897478768, -77.48590718889759899, -4.665239663755555100 ) ) ;
#22981=CARTESIAN_POINT ( 'NONE',  ( -7.229693382246000333, -78.88762021447698203, -6.526195624661000672 ) ) ;
#22988=CARTESIAN_POINT ( 'NONE',  ( 0.000000000000000000, -74.64999999999999147, 0.000000000000000000 ) ) ;
#22994=CARTESIAN_POINT ( 'NONE',  ( 10.68751571525999999, -77.76749638891799066, 3.388774203076999836 ) ) ;
#22999=CARTESIAN_POINT ( 'NONE',  ( -8.396223008680999911, -80.05298179846350592, -4.990405176070999538 ) ) ;
#23005=EDGE_LOOP ( 'NONE', ( #7470, #39053, #4978, #8760 ) ) ;
#23012=CARTESIAN_POINT ( 'NONE',  ( 8.991799503152567041, -79.86894767324388056, 2.169986940879844894 ) ) ;
#23015=CARTESIAN_POINT ( 'NONE',  ( -3.591972190522999764, -77.15527870113453446, 8.980252640667000463 ) ) ;
#23016=CARTESIAN_POINT ( 'NONE',  ( 2.968291740961590985, -77.25116615474895809, -8.760739757934345562 ) ) ;
#23023=EDGE_CURVE ( 'NONE', #44068, #13297, #720, .T. ) ;
#23026=FACE_OUTER_BOUND ( 'NONE', #57989, .T. ) ;
#23032=CARTESIAN_POINT ( 'NONE',  ( 2.943243612629382611, -76.94999999999997442, -9.063334067170245589 ) ) ;
#23035=CARTESIAN_POINT ( 'NONE',  ( 5.436864099232999514, -78.94294275334198119, -8.080855302300999909 ) ) ;
#23041=EDGE_CURVE ( 'NONE', #39698, #24542, #36995, .T. ) ;
#23044=CARTESIAN_POINT ( 'NONE',  ( 7.318097147681000614, -79.67353422943199348, -8.179820946710000484 ) ) ;
#23049=ORIENTED_EDGE ( 'NONE', *, *, #54218, .T. ) ;
#23054=AXIS2_PLACEMENT_3D ( 'NONE', #4848, #49129, #8981 ) ;
#23056=CARTESIAN_POINT ( 'NONE',  ( 10.04848221952999943, -78.59106237267099004, 4.594115663639000147 ) ) ;
#23057=DIRECTION ( 'NONE',  ( 1.000000000000000000, 0.000000000000000000, 0.000000000000000000 ) ) ;
#23062=CARTESIAN_POINT ( 'NONE',  ( -10.96690505107538449, -78.45330275085734684, -0.4413756512486020078 ) ) ;
#23068=VERTEX_POINT ( 'NONE', #46768 ) ;
#23081=CARTESIAN_POINT ( 'NONE',  ( 2.134072831818245142, -77.45658836226374433, 9.000378734383811974 ) ) ;
#23082=CARTESIAN_POINT ( 'NONE',  ( 10.94195044575999987, -77.60922867047798945, -1.468969119710000104 ) ) ;
#23085=CARTESIAN_POINT ( 'NONE',  ( 6.983565664416999219, -78.57937843548099011, -6.737990796766999857 ) ) ;
#23090=CARTESIAN_POINT ( 'NONE',  ( -2.919153588227000107, -78.82568030843599161, 10.54354582977000021 ) ) ;
#23104=CARTESIAN_POINT ( 'NONE',  ( 10.44944364268402026, -78.22927179638983830, -2.857199357458220401 ) ) ;
#23106=CARTESIAN_POINT ( 'NONE',  ( -1.199999999999999956, -80.99999999999998579, 7.000000000000000000 ) ) ;
#23115=EDGE_CURVE ( 'NONE', #36426, #57837, #16703, .T. ) ;
#23132=CARTESIAN_POINT ( 'NONE',  ( -9.467475792354999697, -77.37406124165399035, 1.978357023055999919 ) ) ;
#23136=CARTESIAN_POINT ( 'NONE',  ( -4.985523414424999800, -78.43747757365058249, -9.777963635945001286 ) ) ;
#23162=CARTESIAN_POINT ( 'NONE',  ( 5.927986824875999261, -77.88684073414698616, -7.683077610609999830 ) ) ;
#23166=B_SPLINE_SURFACE_WITH_KNOTS ( 'NONE', 3, 3, ( 
 ( #12499, #52949, #34344, #52380, #11366, #15778, #20785, #52093, #16075, #47682, #6631, #34055, #3077, #11651, #11934, #20219, #47964, #47099, #47387 ),
 ( #29628, #24639, #7499, #25497, #42651, #52662, #12216, #2785, #38786, #2218, #38208, #56805, #33770, #29912, #51809, #21072, #29341, #30204, #6919 ),
 ( #20503, #43814, #38499, #39077, #56517, #57085, #3359, #18398, #31064, #8356, #57657, #18106, #13066, #26354, #40828, #22525, #9245, #35496, #48813 ),
 ( #36101, #39935, #12781, #420, #8652, #54118, #4226, #31654, #49698, #13659, #130, #26936, #44373, #40535, #45269, #30497, #3925, #26638, #54416 ) ),
 .UNSPECIFIED., .F., .F., .F.,
 ( 4, 4 ),
 ( 4, 1, 1, 1, 1, 1, 1, 1, 1, 1, 1, 1, 1, 1, 1, 1, 4 ),
 ( -0.1387574078320999993, 1.138757407831999968 ),
 ( -0.006275936313672000021, 0.01412085670576000013, 0.03451764972519000274, 0.05491444274463000430, 0.07531123576405999998, 0.09570802878349000953, 0.1161048218028999934, 0.1365016148224000025, 0.1568984078418000083, 0.1772952008611999863, 0.1976919938806999955, 0.2180887869001000012, 0.2384855799195000070, 0.2588823729390000161, 0.2792791659584000219, 0.2996759589778000277, 0.3200727519973000090 ),
 .UNSPECIFIED. ) ;
#23169=DIRECTION ( 'NONE',  ( 1.000000000000000000, 0.000000000000000000, 0.000000000000000000 ) ) ;
#23182=CARTESIAN_POINT ( 'NONE',  ( 6.391066299911739357, -79.99999999999998579, -7.100169416382021481 ) ) ;
#23188=CARTESIAN_POINT ( 'NONE',  ( -5.539808784079909287, -79.11666666666667425, 9.611650271896829523 ) ) ;
#23190=CARTESIAN_POINT ( 'NONE',  ( 7.919239162352998740, -79.52960703100998785, -5.689950727604999869 ) ) ;
#23197=CARTESIAN_POINT ( 'NONE',  ( 10.99516458417999942, -77.41144710480799063, -2.492447527329999968 ) ) ;
#23200=CARTESIAN_POINT ( 'NONE',  ( -4.341134711875000107, -79.10767126595499121, -8.352589043283000336 ) ) ;
#23210=CARTESIAN_POINT ( 'NONE',  ( 10.68099162494999987, -79.63817051509798262, 2.367326398803000220 ) ) ;
#23227=CONICAL_SURFACE ( 'NONE', #30742, 2.699999999213000379, 0.7853981633972997312 ) ;
#23230=CARTESIAN_POINT ( 'NONE',  ( 8.445116086859872695, -78.14089606339597083, 4.780569220243218176 ) ) ;
#23237=CARTESIAN_POINT ( 'NONE',  ( 0.6886906644032062541, -78.73113614952505657, -9.226155803845061953 ) ) ;
#23241=CARTESIAN_POINT ( 'NONE',  ( -7.310560282016263400, -80.16762514998541178, -8.219721594426141920 ) ) ;
#23248=DIRECTION ( 'NONE',  ( -1.000000000000000000, 0.000000000000000000, 0.000000000000000000 ) ) ;
#23251=DIRECTION ( 'NONE',  ( 0.000000000000000000, 0.7071067811866525998, -0.7071067811864425456 ) ) ;
#23258=AXIS2_PLACEMENT_3D ( 'NONE', #4389, #49262, #45432 ) ;
#23265=CONICAL_SURFACE ( 'NONE', #35501, 10.59999999995999964, 0.7853981633972997312 ) ;
#23285=CARTESIAN_POINT ( 'NONE',  ( 3.606090020748000224, -77.20773208238998109, -10.73262889482999860 ) ) ;
#23292=CARTESIAN_POINT ( 'NONE',  ( 8.985706068735000329, -79.72825521588151787, -3.828549499589000149 ) ) ;
#23304=CARTESIAN_POINT ( 'NONE',  ( 8.994180132603776912, -79.86886303493331241, 2.160082921624130403 ) ) ;
#23318=DIRECTION ( 'NONE',  ( 1.308348598714000038E-10, -1.000000000000000000, 3.608116327059999754E-10 ) ) ;
#23321=DIRECTION ( 'NONE',  ( 1.000000000000000000, 0.000000000000000000, 0.000000000000000000 ) ) ;
#23331=CARTESIAN_POINT ( 'NONE',  ( -8.614692902062000002, -77.17363726482008701, 3.831263898871999807 ) ) ;
#23338=CARTESIAN_POINT ( 'NONE',  ( -7.604423127187000198, -79.92636541842598774, 7.914351627518998455 ) ) ;
#23358=CARTESIAN_POINT ( 'NONE',  ( 9.981997996688200203, -78.73422629418405450, 4.563719410465792770 ) ) ;
#23378=CARTESIAN_POINT ( 'NONE',  ( 9.068127558788219744, -77.36599329621280674, 1.827539330042447174 ) ) ;
#23379=CARTESIAN_POINT ( 'NONE',  ( 6.393001003723999709, -77.25600538349898727, 9.000752526674000720 ) ) ;
#23386=CARTESIAN_POINT ( 'NONE',  ( 4.025753977166000475, -79.58417387541800281, -10.17256709246999868 ) ) ;
#23390=ORIENTED_EDGE ( 'NONE', *, *, #51415, .T. ) ;
#23401=CARTESIAN_POINT ( 'NONE',  ( 9.227078657215999513, -77.81332916973599367, -1.863387764540999969 ) ) ;
#23410=CARTESIAN_POINT ( 'NONE',  ( -3.548303639235999896, -79.40834838942097917, -10.38621961377000069 ) ) ;
#23422=CARTESIAN_POINT ( 'NONE',  ( 0.000000000000000000, -74.99999999999998579, 0.000000000000000000 ) ) ;
#23443=CARTESIAN_POINT ( 'NONE',  ( 3.792898146759813738, -78.25866108564824231, -8.437158711453742299 ) ) ;
#23451=CARTESIAN_POINT ( 'NONE',  ( -9.669247687117000112, -77.77660068504400215, -0.8224101967608999919 ) ) ;
#23466=VECTOR ( 'NONE', #55554, 1000.000000000000000 ) ;
#23473=CARTESIAN_POINT ( 'NONE',  ( 9.611650271896847286, -78.99166666666666003, 5.539808784079873760 ) ) ;
#23474=CARTESIAN_POINT ( 'NONE',  ( -7.567403614301999148, -79.38349373972098988, -6.150145586324001101 ) ) ;
#23479=DIRECTION ( 'NONE',  ( 0.000000000000000000, -1.000000000000000000, 0.000000000000000000 ) ) ;
#23481=CARTESIAN_POINT ( 'NONE',  ( -4.869124390976999450, -77.26864856148100102, -10.16845940041999974 ) ) ;
#23485=CARTESIAN_POINT ( 'NONE',  ( -9.004250860540000900, -77.54436066386098503, -2.744961831234999927 ) ) ;
#23515=CARTESIAN_POINT ( 'NONE',  ( -9.479095156995775540, -77.35887667588667682, -1.070679073321031183 ) ) ;
#23523=CARTESIAN_POINT ( 'NONE',  ( 7.802584695901705558, -78.80492006119759196, -4.968624645346182866 ) ) ;
#23527=CARTESIAN_POINT ( 'NONE',  ( -7.600204320007741821, -80.16470501430156048, -7.951820076216480793 ) ) ;
#23542=CARTESIAN_POINT ( 'NONE',  ( -10.68003080091532375, -77.44002302599371035, 1.404162012696734463 ) ) ;
#23551=CARTESIAN_POINT ( 'NONE',  ( 8.326085669973442904, -78.31415593885135706, -4.029697569531446533 ) ) ;
#23555=CARTESIAN_POINT ( 'NONE',  ( -9.628933692773001596, -78.89464829700199289, -0.1919528651714999812 ) ) ;
#23557=CYLINDRICAL_SURFACE ( 'NONE', #5346, 11.00000000000000000 ) ;
#23568=DIRECTION ( 'NONE',  ( 0.000000000000000000, 0.000000000000000000, -1.000000000000000000 ) ) ;
#23572=CARTESIAN_POINT ( 'NONE',  ( -6.091193159344999941, -77.07048692427588321, -8.944723388890000848 ) ) ;
#23576=CARTESIAN_POINT ( 'NONE',  ( 5.411006671257999834, -79.21873047333799889, 8.131518144102999557 ) ) ;
#23579=EDGE_CURVE ( 'NONE', #2832, #45010, #54202, .T. ) ;
#23582=EDGE_CURVE ( 'NONE', #45667, #12448, #55654, .T. ) ;
#23589=CARTESIAN_POINT ( 'NONE',  ( -1.867777256262999952, -77.16087362948169925, 9.751254915078000352 ) ) ;
#23602=CARTESIAN_POINT ( 'NONE',  ( 5.471330588277999674, -78.45546044413198672, 9.848526282906998830 ) ) ;
#23608=CARTESIAN_POINT ( 'NONE',  ( -8.262032057783999406, -77.35055961578798644, 4.886512119495000306 ) ) ;
#23609=DIRECTION ( 'NONE',  ( 0.000000000000000000, -1.000000000000000000, 0.000000000000000000 ) ) ;
#23614=CARTESIAN_POINT ( 'NONE',  ( 2.845884614340000063, -77.85580916391599260, -9.200769029100998253 ) ) ;
#23625=CARTESIAN_POINT ( 'NONE',  ( -10.81649518602000093, -79.47688774910298548, 1.862108609190000097 ) ) ;
#23626=CARTESIAN_POINT ( 'NONE',  ( 6.760013919724043419, -79.27708333333333712, -8.796335266379996298 ) ) ;
#23644=CARTESIAN_POINT ( 'NONE',  ( -2.169201898071945855, -78.34093333352706168, 10.75929280804342447 ) ) ;
#23663=CARTESIAN_POINT ( 'NONE',  ( 8.795818401383446172, -77.37508321831271019, 2.862770402330162334 ) ) ;
#23664=CARTESIAN_POINT ( 'NONE',  ( -9.050627908549000011, -77.53897626982698910, -6.322205650057999726 ) ) ;
#23671=DIRECTION ( 'NONE',  ( 0.000000000000000000, 0.7071067811866525998, -0.7071067811864425456 ) ) ;
#23672=CARTESIAN_POINT ( 'NONE',  ( 6.591600424694998850, -79.75272800141398477, 8.731473042948000085 ) ) ;
#23684=AXIS2_PLACEMENT_3D ( 'NONE', #24882, #21312, #2457 ) ;
#23688=CARTESIAN_POINT ( 'NONE',  ( -7.831519877845000366, -78.12599129015498534, -5.222881475815000840 ) ) ;
#23698=CARTESIAN_POINT ( 'NONE',  ( -9.091539081997000338, -78.76222423976999210, 6.148815634104000338 ) ) ;
#23708=( GEOMETRIC_REPRESENTATION_CONTEXT ( 3 ) GLOBAL_UNCERTAINTY_ASSIGNED_CONTEXT ( ( #25408 ) ) GLOBAL_UNIT_ASSIGNED_CONTEXT ( ( #48490, #52341, #6880 ) ) REPRESENTATION_CONTEXT ( 'NONE', 'WORKASPACE' ) );
#23715=CARTESIAN_POINT ( 'NONE',  ( 10.36935812844000004, -78.07876026662599145, -2.835297515976000327 ) ) ;
#23723=ORIENTED_EDGE ( 'NONE', *, *, #54792, .T. ) ;
#23727=ORIENTED_EDGE ( 'NONE', *, *, #40552, .T. ) ;
#23734=CARTESIAN_POINT ( 'NONE',  ( 3.571212153075712159, -78.25658151030941667, -8.532799217283892901 ) ) ;
#23736=VERTEX_POINT ( 'NONE', #17521 ) ;
#23738=CARTESIAN_POINT ( 'NONE',  ( -8.069289515393755607, -77.55933884297279235, 4.525049359534452087 ) ) ;
#23742=CARTESIAN_POINT ( 'NONE',  ( 8.898653440358000211, -78.48719641326798069, -3.871004561473999850 ) ) ;
#23749=B_SPLINE_CURVE_WITH_KNOTS ( 'NONE', 3,
 ( #27018, #45054, #44750, #4606, #40615, #19932, #23188, #19634, #32606, #1353, #41780, #5756, #1645, #32897, #23473, #37631, #37922, #5182 ),
 .UNSPECIFIED., .F., .F.,
 ( 4, 2, 2, 2, 2, 2, 2, 2, 4 ),
 ( 0.000000000000000000, 0.1250000000000000000, 0.2500000000000000000, 0.3750000000000000000, 0.5000000000000000000, 0.6250000000000000000, 0.7500000000000000000, 0.8750000000000000000, 1.000000000000000000 ),
 .UNSPECIFIED. ) ;
#23757=CARTESIAN_POINT ( 'NONE',  ( -5.685008486195640032, -79.52738042223084847, 7.397161007072386774 ) ) ;
#23759=CARTESIAN_POINT ( 'NONE',  ( -2.561320322697239860, -77.20000000000000284, -10.72273578054103105 ) ) ;
#23761=CARTESIAN_POINT ( 'NONE',  ( -11.00000000000000000, -78.21041666666667425, -1.439896632895322881 ) ) ;
#23765=CARTESIAN_POINT ( 'NONE',  ( -3.950656329793999610, -79.23738044843098294, 8.915279242129001247 ) ) ;
#23769=VECTOR ( 'NONE', #40690, 1000.000000000000000 ) ;
#23772=CARTESIAN_POINT ( 'NONE',  ( -3.929469618655000218, -77.64668109758299863, 10.45105132569000084 ) ) ;
#23773=EDGE_CURVE ( 'NONE', #43973, #31318, #35883, .T. ) ;
#23776=CARTESIAN_POINT ( 'NONE',  ( -8.866000417715000026, -77.49698761531298885, 2.742227037787000388 ) ) ;
#23783=LINE ( 'NONE', #41799, #46439 ) ;
#23789=DIRECTION ( 'NONE',  ( 0.000000000000000000, 1.000000000000000000, 0.000000000000000000 ) ) ;
#23802=CARTESIAN_POINT ( 'NONE',  ( -9.250000000000000000, -79.09999999999999432, 1.813240672189999963E-14 ) ) ;
#23803=CARTESIAN_POINT ( 'NONE',  ( 11.00000000000000000, -78.84999999999999432, 0.000000000000000000 ) ) ;
#23808=CARTESIAN_POINT ( 'NONE',  ( 9.703485699160999900, -77.50093816103475319, 0.1143444355825999903 ) ) ;
#23813=CARTESIAN_POINT ( 'NONE',  ( 0.4089082674944940488, -78.72870479441709790, -9.241335590917220344 ) ) ;
#23825=CARTESIAN_POINT ( 'NONE',  ( 0.007687615972125512107, -79.99999999999997158, 9.299168372948120265 ) ) ;
#23830=EDGE_CURVE ( 'NONE', #13151, #55023, #14759, .T. ) ;
#23834=CARTESIAN_POINT ( 'NONE',  ( -9.834111732579202680, -78.13812671110433428, -5.101590220333411807 ) ) ;
#23842=CARTESIAN_POINT ( 'NONE',  ( 8.766282146675060005, -78.32424052224494915, -2.952264042087271001 ) ) ;
#23846=CARTESIAN_POINT ( 'NONE',  ( -1.966850719965000494, -77.43800492889899090, -9.538930191946999315 ) ) ;
#23857=CARTESIAN_POINT ( 'NONE',  ( -1.919663510025999997, -79.79090199409699835, -11.39231233529999976 ) ) ;
#23860=CARTESIAN_POINT ( 'NONE',  ( -8.573168234377000374, -77.43733401092899271, 7.225480548498000033 ) ) ;
#23866=LINE ( 'NONE', #31839, #44286 ) ;
#23867=VECTOR ( 'NONE', #27532, 1000.000000000000000 ) ;
#23869=CARTESIAN_POINT ( 'NONE',  ( 1.841371367509999857, -80.15039977323749554, -9.592189096167999196 ) ) ;
#23870=ORIENTED_EDGE ( 'NONE', *, *, #24591, .F. ) ;
#23879=DIRECTION ( 'NONE',  ( 3.675128825892999315E-09, -0.9999999999999997780, -2.168720766502999921E-08 ) ) ;
#23898=CARTESIAN_POINT ( 'NONE',  ( -9.358039826156000274, -77.40277834972398807, -1.148306349242000035 ) ) ;
#23904=CARTESIAN_POINT ( 'NONE',  ( 1.867960828343000035, -78.56640489213999956, 9.447959161044998666 ) ) ;
#23906=DIRECTION ( 'NONE',  ( 0.000000000000000000, 1.000000000000000000, 0.000000000000000000 ) ) ;
#23912=EDGE_CURVE ( 'NONE', #6475, #33222, #40192, .T. ) ;
#23914=CARTESIAN_POINT ( 'NONE',  ( -8.631379868284000167, -78.43747063879398240, 6.779623747090999686 ) ) ;
#23917=CARTESIAN_POINT ( 'NONE',  ( -2.833621800687999848, -79.24439682224598869, -9.245833289607000793 ) ) ;
#23920=EDGE_LOOP ( 'NONE', ( #2478, #6598, #38828, #6370, #13843, #6225, #12108, #24445, #29531, #14121, #36602 ) ) ;
#23932=CARTESIAN_POINT ( 'NONE',  ( -2.928650166838424607, -78.84659571151506441, 10.57784605029244318 ) ) ;
#23936=ORIENTED_EDGE ( 'NONE', *, *, #7844, .T. ) ;
#23940=CYLINDRICAL_SURFACE ( 'NONE', #56686, 10.69999999999999929 ) ;
#23951=CARTESIAN_POINT ( 'NONE',  ( 8.775623107093144526, -77.37563063860072532, 2.924238520614950598 ) ) ;
#23959=CARTESIAN_POINT ( 'NONE',  ( -9.475012188928999990, -79.38752739508899481, 5.469182786826999987 ) ) ;
#23976=CARTESIAN_POINT ( 'NONE',  ( -9.066428667704000688, -77.55751470757499533, 2.532008238717000204 ) ) ;
#23988=CARTESIAN_POINT ( 'NONE',  ( 8.318585563179999198, -78.17640301578899198, 7.159970128962999780 ) ) ;
#24000=PLANE ( 'NONE',  #56563 ) ;
#24024=EDGE_CURVE ( 'NONE', #40455, #25733, #11843, .T. ) ;
#24027=CARTESIAN_POINT ( 'NONE',  ( 6.647991942108485652, -78.28881406770516094, -6.431782383451233542 ) ) ;
#24031=CARTESIAN_POINT ( 'NONE',  ( -7.514168461771876473, -77.55044855222018896, 5.394443598068082935 ) ) ;
#24035=CARTESIAN_POINT ( 'NONE',  ( -8.771427373352999268, -77.80502451417299881, -4.151237309591000013 ) ) ;
#24052=CARTESIAN_POINT ( 'NONE',  ( 9.760313732895301797, -77.19999999999998863, -4.644364491930659256 ) ) ;
#24054=CARTESIAN_POINT ( 'NONE',  ( -2.879226727952071574, -78.30416666666667425, -10.71369944335147473 ) ) ;
#24055=CARTESIAN_POINT ( 'NONE',  ( -2.899238502638000092, -78.22541024847198798, -11.05877603816999866 ) ) ;
#24059=CARTESIAN_POINT ( 'NONE',  ( 6.097124503614000268, -79.21358821443999432, 7.470160346181000222 ) ) ;
#24062=AXIS2_PLACEMENT_3D ( 'NONE', #25353, #53092, #12644 ) ;
#24066=CARTESIAN_POINT ( 'NONE',  ( 1.004082900143999924, -77.81128302612299308, -11.22932683135000076 ) ) ;
#24070=CARTESIAN_POINT ( 'NONE',  ( 0.8359750594766999221, -78.65288999989098784, -9.376158072868999938 ) ) ;
#24075=DIRECTION ( 'NONE',  ( 0.000000000000000000, -1.000000000000000000, 0.000000000000000000 ) ) ;
#24086=ORIENTED_EDGE ( 'NONE', *, *, #31333, .F. ) ;
#24087=ORIENTED_EDGE ( 'NONE', *, *, #40552, .F. ) ;
#24098=CARTESIAN_POINT ( 'NONE',  ( 2.398213954452620644, -79.24598686563928140, -8.954150635807138769 ) ) ;
#24110=CARTESIAN_POINT ( 'NONE',  ( -7.168972154839425848, -78.65447478827950079, -5.845467487007924845 ) ) ;
#24130=CARTESIAN_POINT ( 'NONE',  ( 10.61050599188999932, -78.32876026662599145, -2.901234667509999809 ) ) ;
#24131=CARTESIAN_POINT ( 'NONE',  ( -10.90760146693999921, -78.85886288864057292, -1.219937219691999974 ) ) ;
#24137=CARTESIAN_POINT ( 'NONE',  ( 7.542821534244515291, -78.30104360775493433, -5.354097004516040315 ) ) ;
#24141=CARTESIAN_POINT ( 'NONE',  ( -8.954089450906998593, -78.92307212613098955, -3.546476007522999740 ) ) ;
#24152=VERTEX_POINT ( 'NONE', #9476 ) ;
#24154=CARTESIAN_POINT ( 'NONE',  ( 9.759566573192998362, -79.51811006564999218, -5.179648052473000419 ) ) ;
#24155=CARTESIAN_POINT ( 'NONE',  ( -2.309473414332742891, -77.60514816509892455, -9.037436301258047422 ) ) ;
#24156=LINE ( 'NONE', #56042, #52023 ) ;
#24159=CARTESIAN_POINT ( 'NONE',  ( -11.15272124962999989, -77.63845490982699005, -2.513729164015999995 ) ) ;
#24166=CARTESIAN_POINT ( 'NONE',  ( -9.699833017908000343, -79.38109376462799105, 1.146274062705999963 ) ) ;
#24178=CARTESIAN_POINT ( 'NONE',  ( -9.404328087084998344, -77.22694376941500138, -0.9147582690626000490 ) ) ;
#24197=CARTESIAN_POINT ( 'NONE',  ( 5.173304380012000436, -77.06335657913808745, -8.085540331045999451 ) ) ;
#24203=CARTESIAN_POINT ( 'NONE',  ( 9.084121021304000010, -77.55017512602198337, 3.512611703280999809 ) ) ;
#24205=CARTESIAN_POINT ( 'NONE',  ( -5.751575622429521140, -77.09192708334455801, 7.482738014362807277 ) ) ;
#24211=DIRECTION ( 'NONE',  ( 1.000000000000000000, 0.000000000000000000, 0.000000000000000000 ) ) ;
#24212=CARTESIAN_POINT ( 'NONE',  ( 4.634563706678000550, -78.83076359945098943, 9.949112313689999709 ) ) ;
#24213=CARTESIAN_POINT ( 'NONE',  ( -10.96337388901621424, -80.09393029936845210, 0.8942561643144778527 ) ) ;
#24214=CARTESIAN_POINT ( 'NONE',  ( 5.718781654312999230, -79.25521639797898388, -7.660718028547000458 ) ) ;
#24233=CARTESIAN_POINT ( 'NONE',  ( -9.091682561854286249, -78.90278042018009330, 6.148912672809537128 ) ) ;
#24250=ADVANCED_FACE ( 'NONE', ( #36623, #18337 ), #54061, .F. ) ;
#24254=CARTESIAN_POINT ( 'NONE',  ( 7.625531225268916913, -77.39806426064797051, 5.241218712637033761 ) ) ;
#24262=CARTESIAN_POINT ( 'NONE',  ( 3.325053339351000226, -79.14238723821299004, -10.53669369097999997 ) ) ;
#24272=AXIS2_PLACEMENT_3D ( 'NONE', #14225, #54400, #979 ) ;
#24276=CARTESIAN_POINT ( 'NONE',  ( 6.774287055642999711, -78.26811043579999705, -6.536071403775000732 ) ) ;
#24281=ORIENTED_EDGE ( 'NONE', *, *, #125, .F. ) ;
#24287=CARTESIAN_POINT ( 'NONE',  ( -9.438868967565998247, -79.35216368075597870, -5.601050722391000214 ) ) ;
#24288=AXIS2_PLACEMENT_3D ( 'NONE', #40899, #44444, #22598 ) ;
#24298=EDGE_CURVE ( 'NONE', #47767, #21227, #28031, .T. ) ;
#24311=( NAMED_UNIT ( * ) PLANE_ANGLE_UNIT ( ) SI_UNIT ( $, .RADIAN. ) );
#24321=DIRECTION ( 'NONE',  ( 0.000000000000000000, -1.000000000000000000, 0.000000000000000000 ) ) ;
#24325=CARTESIAN_POINT ( 'NONE',  ( 7.369188213045021918, -78.29848014924698418, -5.592313299527890358 ) ) ;
#24330=VERTEX_POINT ( 'NONE', #39279 ) ;
#24335=DIRECTION ( 'NONE',  ( -0.3090169943748909409, 0.000000000000000000, -0.9510565162951718499 ) ) ;
#24337=CARTESIAN_POINT ( 'NONE',  ( 8.240135455977000589, -77.97556748894699297, -5.125512367919999868 ) ) ;
#24341=DIRECTION ( 'NONE',  ( -1.000000000000000000, 0.000000000000000000, 0.000000000000000000 ) ) ;
#24352=CARTESIAN_POINT ( 'NONE',  ( -7.397034735012056217, -79.54824835870380184, 5.685233668030444498 ) ) ;
#24357=CARTESIAN_POINT ( 'NONE',  ( -11.00000000000000000, -78.19999999999998863, 0.000000000000000000 ) ) ;
#24360=CARTESIAN_POINT ( 'NONE',  ( -1.461485599008999881, -79.56969053780299816, -9.420958682499000147 ) ) ;
#24362=CARTESIAN_POINT ( 'NONE',  ( 9.499157866768639380, -79.10080562451891240, 0.1004279358040388037 ) ) ;
#24368=CARTESIAN_POINT ( 'NONE',  ( 9.328312098178999534, -77.44676313692498582, -6.135780202701999642 ) ) ;
#24371=CARTESIAN_POINT ( 'NONE',  ( 6.774287055642999711, -78.70973765814899537, -6.536071403775000732 ) ) ;
#24388=VERTEX_POINT ( 'NONE', #15983 ) ;
#24393=ORIENTED_EDGE ( 'NONE', *, *, #24763, .F. ) ;
#24404=CARTESIAN_POINT ( 'NONE',  ( -1.565122400816999937, -78.63789132619378108, 9.577113408380000692 ) ) ;
#24409=CARTESIAN_POINT ( 'NONE',  ( -6.537703431114865182, -78.66257577246084054, -6.543724569677213054 ) ) ;
#24412=CARTESIAN_POINT ( 'NONE',  ( -5.423101880016904630, -80.18407044839175057, -9.570620509585031854 ) ) ;
#24418=ADVANCED_FACE ( 'NONE', ( #16564 ), #7211, .F. ) ;
#24424=CARTESIAN_POINT ( 'NONE',  ( -9.250000000000000000, -79.59999999999999432, 0.000000000000000000 ) ) ;
#24425=CARTESIAN_POINT ( 'NONE',  ( 0.000000000000000000, -81.10000000285099020, -7.000000000000000000 ) ) ;
#24428=CARTESIAN_POINT ( 'NONE',  ( 10.07284277676071227, -77.73062272438683351, 4.003573653696650858 ) ) ;
#24430=CARTESIAN_POINT ( 'NONE',  ( 3.176617583302000725, -79.70163351862059642, 10.50586082162000068 ) ) ;
#24437=CARTESIAN_POINT ( 'NONE',  ( 7.497431372734266297, -78.30036608647220930, -5.417634822929890959 ) ) ;
#24441=CARTESIAN_POINT ( 'NONE',  ( 7.433005562543999467, -77.52327641628599508, -6.293657445383999516 ) ) ;
#24443=CARTESIAN_POINT ( 'NONE',  ( 7.588757936995927963E-07, -80.21583927563050054, -10.98470495943546688 ) ) ;
#24445=ORIENTED_EDGE ( 'NONE', *, *, #17110, .F. ) ;
#24451=CARTESIAN_POINT ( 'NONE',  ( -7.299994274544086892, -77.55341536691996396, -5.806806862848980622 ) ) ;
#24452=CARTESIAN_POINT ( 'NONE',  ( -10.77729720431999993, -80.20851364748298806, -4.161934381267000660 ) ) ;
#24455=CARTESIAN_POINT ( 'NONE',  ( 0.5827356580765999938, -77.42784033438199742, 11.30719494610999831 ) ) ;
#24463=CARTESIAN_POINT ( 'NONE',  ( -7.545891804452000251, -80.19526951059052067, 6.201630566990999682 ) ) ;
#24464=ORIENTED_EDGE ( 'NONE', *, *, #5184, .F. ) ;
#24473=CARTESIAN_POINT ( 'NONE',  ( 9.279687143926999227, -76.88845924204508719, 2.683876840368999872 ) ) ;
#24475=CARTESIAN_POINT ( 'NONE',  ( -11.00000000000000000, -79.59999999999999432, 0.000000000000000000 ) ) ;
#24477=CARTESIAN_POINT ( 'NONE',  ( -1.210822168571097146, -77.88541666666665719, 9.249999999999992895 ) ) ;
#24494=CARTESIAN_POINT ( 'NONE',  ( 4.763371395742999503, -77.43647980950599674, -8.495292134120999705 ) ) ;
#24505=CARTESIAN_POINT ( 'NONE',  ( 9.417408019640999939, -79.81543127184799857, -1.644225498658999918 ) ) ;
#24507=CARTESIAN_POINT ( 'NONE',  ( -1.210822168571057400, -79.11458333333335702, -9.250000000000001776 ) ) ;
#24516=EDGE_CURVE ( 'NONE', #38602, #4702, #9160, .T. ) ;
#24525=ORIENTED_EDGE ( 'NONE', *, *, #51735, .F. ) ;
#24529=VERTEX_POINT ( 'NONE', #40742 ) ;
#24532=B_SPLINE_CURVE_WITH_KNOTS ( 'NONE', 3,
 ( #5028, #50495, #15043, #32450 ),
 .UNSPECIFIED., .F., .F.,
 ( 4, 4 ),
 ( 0.000000000000000000, 1.000000000000000000 ),
 .UNSPECIFIED. ) ;
#24542=VERTEX_POINT ( 'NONE', #22731 ) ;
#24543=CARTESIAN_POINT ( 'NONE',  ( 9.134591787879230651, -77.36274324294630844, 1.455986419346108507 ) ) ;
#24544=CARTESIAN_POINT ( 'NONE',  ( -7.062685404271999978, -77.92069277381098402, 8.485436034813998774 ) ) ;
#24547=DIRECTION ( 'NONE',  ( 0.7071067811864980568, 0.7071067811865969777, -6.547095300151979771E-10 ) ) ;
#24552=CARTESIAN_POINT ( 'NONE',  ( 8.374122929021998729, -78.29961660823299496, 7.207772231549999908 ) ) ;
#24566=CARTESIAN_POINT ( 'NONE',  ( -4.391285525405000278, -78.72991978438899707, -8.449082048777999177 ) ) ;
#24580=CARTESIAN_POINT ( 'NONE',  ( 10.28103400416999946, -78.20861358712699030, 3.842432268884000024 ) ) ;
#24589=CARTESIAN_POINT ( 'NONE',  ( -11.00000000000000711, -78.18958333333333144, 1.439896632895276696 ) ) ;
#24591=EDGE_CURVE ( 'NONE', #25733, #29374, #56185, .T. ) ;
#24592=CARTESIAN_POINT ( 'NONE',  ( 9.887211716164999942, -78.96897326909299863, 5.401109038458000278 ) ) ;
#24599=ORIENTED_EDGE ( 'NONE', *, *, #37170, .F. ) ;
#24601=CARTESIAN_POINT ( 'NONE',  ( -11.00000000000000711, -79.58958333333332291, 1.439896632895279138 ) ) ;
#24610=CARTESIAN_POINT ( 'NONE',  ( -4.559293336502967087, -80.44036368348199062, -9.818763842569914857 ) ) ;
#24615=CARTESIAN_POINT ( 'NONE',  ( -1.525577938756555785, -78.21193052228882436, -9.123864793022928410 ) ) ;
#24619=CARTESIAN_POINT ( 'NONE',  ( -8.891768023477260030, -77.57778467934028299, 2.551063254158453475 ) ) ;
#24624=CARTESIAN_POINT ( 'NONE',  ( 9.583411031200000707, -78.03241514720498628, 1.526087275887999972 ) ) ;
#24639=CARTESIAN_POINT ( 'NONE',  ( -9.474082757681998146, -79.95148679530498725, 5.468759164920000693 ) ) ;
#24649=CARTESIAN_POINT ( 'NONE',  ( -6.456202977062000414, -79.89113977864099070, 7.014830417985999489 ) ) ;
#24656=CARTESIAN_POINT ( 'NONE',  ( 6.450682458815999887, -77.54595490982698891, -8.845531009145000567 ) ) ;
#24661=CARTESIAN_POINT ( 'NONE',  ( -2.495045882587000108, -78.62446617076199118, -9.076670124625998426 ) ) ;
#24679=ORIENTED_EDGE ( 'NONE', *, *, #29166, .F. ) ;
#24693=CARTESIAN_POINT ( 'NONE',  ( 9.259046916275000427, -78.52419600967778024, 2.905298533503999803 ) ) ;
#24697=CARTESIAN_POINT ( 'NONE',  ( -5.539808784079931492, -78.61666666666667425, 9.611650271896815312 ) ) ;
#24699=CARTESIAN_POINT ( 'NONE',  ( -7.448626198570991619, -78.65061730849956234, -5.485182927975110090 ) ) ;
#24702=CARTESIAN_POINT ( 'NONE',  ( -10.88354252222900520, -80.11174396849405355, -1.596899905050069401 ) ) ;
#24710=B_SPLINE_CURVE_WITH_KNOTS ( 'NONE', 3,
 ( #5368, #36945, #54956, #14509 ),
 .UNSPECIFIED., .F., .F.,
 ( 4, 4 ),
 ( 0.000000000000000000, 1.000000000000000000 ),
 .UNSPECIFIED. ) ;
#24719=CARTESIAN_POINT ( 'NONE',  ( 7.782819286693597682, -77.76121216632311928, 7.448878563881510040 ) ) ;
#24722=DIRECTION ( 'NONE',  ( 0.000000000000000000, 1.000000000000000000, 0.000000000000000000 ) ) ;
#24726=CARTESIAN_POINT ( 'NONE',  ( 9.191416345675177624, -78.34109437452993063, -1.039168553220889635 ) ) ;
#24730=CARTESIAN_POINT ( 'NONE',  ( -8.803456334546002182, -77.86436236583298864, -4.166395597179999299 ) ) ;
#24743=CARTESIAN_POINT ( 'NONE',  ( 0.3834289305765000155, -77.68463329503899217, -11.31570682219000012 ) ) ;
#24752=CARTESIAN_POINT ( 'NONE',  ( -5.726462542197000793, -80.32516014362252577, -7.912542777261000637 ) ) ;
#24761=B_SPLINE_CURVE_WITH_KNOTS ( 'NONE', 3,
 ( #5272, #40705, #18572, #26811 ),
 .UNSPECIFIED., .F., .F.,
 ( 4, 4 ),
 ( 0.7500000006367434358, 1.000000000000000000 ),
 .UNSPECIFIED. ) ;
#24763=EDGE_CURVE ( 'NONE', #33222, #46115, #5588, .T. ) ;
#24765=CARTESIAN_POINT ( 'NONE',  ( -9.078045636453000000, -77.18772503547859287, 3.793810669397000179 ) ) ;
#24767=CARTESIAN_POINT ( 'NONE',  ( 5.539808784079905735, -79.76666666666666572, -9.611650271896829523 ) ) ;
#24773=DIRECTION ( 'NONE',  ( 0.000000000000000000, 1.000000000000000000, 0.000000000000000000 ) ) ;
#24779=CARTESIAN_POINT ( 'NONE',  ( -0.8436256567094999603, -76.94726210441848480, -9.670559092448998584 ) ) ;
#24784=CARTESIAN_POINT ( 'NONE',  ( -9.480927541711999140, -78.28919468337598175, -2.229732866345000009 ) ) ;
#24796=CARTESIAN_POINT ( 'NONE',  ( -2.967406986365000332, -79.47930234752600143, 9.087659770315999808 ) ) ;
#24814=CARTESIAN_POINT ( 'NONE',  ( 9.202039358297998461, -79.97952878580598224, 2.360608321670000453 ) ) ;
#24832=CARTESIAN_POINT ( 'NONE',  ( 5.585446503142362573, -77.27674399426018681, -7.373492375193941406 ) ) ;
#24834=CARTESIAN_POINT ( 'NONE',  ( 10.50000000000000000, -76.19999999999998863, 0.000000000000000000 ) ) ;
#24843=CARTESIAN_POINT ( 'NONE',  ( 10.78711022396000097, -79.76041903353200269, 2.390846439793999689 ) ) ;
#24857=CARTESIAN_POINT ( 'NONE',  ( -0.1509935689429000305, -78.01932405616399535, 9.520902119764999227 ) ) ;
#24868=CARTESIAN_POINT ( 'NONE',  ( 1.684372618195999927, -78.29289065012498838, 10.84559388857000073 ) ) ;
#24879=CARTESIAN_POINT ( 'NONE',  ( -7.208482872893000604, -79.10943504075699195, 8.658331769851001170 ) ) ;
#24882=CARTESIAN_POINT ( 'NONE',  ( 0.000000000000000000, -81.10000000285099020, 7.000000000000000000 ) ) ;
#24894=EDGE_LOOP ( 'NONE', ( #49139, #53096 ) ) ;
#24899=DIRECTION ( 'NONE',  ( 1.000000000000000000, 0.000000000000000000, 0.000000000000000000 ) ) ;
#24902=CARTESIAN_POINT ( 'NONE',  ( -5.706960677091378997, -79.42732870794154110, 7.378979574796262320 ) ) ;
#24906=ADVANCED_FACE ( 'NONE', ( #29471 ), #21359, .T. ) ;
#24907=CARTESIAN_POINT ( 'NONE',  ( -9.139685035454183648, -77.58784146180079233, 1.423788756781738885 ) ) ;
#24911=CARTESIAN_POINT ( 'NONE',  ( -9.022250383429000209, -78.86016145935799670, -3.573472734901999903 ) ) ;
#24932=CARTESIAN_POINT ( 'NONE',  ( -9.109442592336732147, -77.14879300455254452, -2.108685836323368257 ) ) ;
#24933=CARTESIAN_POINT ( 'NONE',  ( 8.372594970691999094, -79.18436555618200146, 4.783109303148000535 ) ) ;
#24935=CARTESIAN_POINT ( 'NONE',  ( 6.143730674703169470, -79.17034681202650859, 7.527261947263182762 ) ) ;
#24939=B_SPLINE_CURVE_WITH_KNOTS ( 'NONE', 3,
 ( #27465, #35149, #44616, #44320 ),
 .UNSPECIFIED., .F., .F.,
 ( 4, 4 ),
 ( 0.0008525611273306000007, 1.000000000000000000 ),
 .UNSPECIFIED. ) ;
#24941=CARTESIAN_POINT ( 'NONE',  ( -10.67331332832999991, -77.88867141381099657, -2.436207225683000299 ) ) ;
#24946=CARTESIAN_POINT ( 'NONE',  ( 2.309272084855999996, -76.91403361972609787, -9.392260232199999948 ) ) ;
#24950=ADVANCED_FACE ( 'NONE', ( #51362 ), #23265, .T. ) ;
#24977=CARTESIAN_POINT ( 'NONE',  ( -6.579851013319285791, -79.78402246038903911, 7.149177186347576374 ) ) ;
#24978=CARTESIAN_POINT ( 'NONE',  ( -8.325060287279862692, -77.30740476286068485, 4.923789656685126914 ) ) ;
#24981=EDGE_CURVE ( 'NONE', #20866, #43667, #50632, .T. ) ;
#24982=CARTESIAN_POINT ( 'NONE',  ( -2.851745628345378591, -78.70021968422466330, -8.800581811362720330 ) ) ;
#25001=CARTESIAN_POINT ( 'NONE',  ( -10.63212904442447559, -77.96514177923053524, -1.980916397344540281 ) ) ;
#25011=CARTESIAN_POINT ( 'NONE',  ( -7.068247108407000212, -79.01537169604299038, -6.380459158363000149 ) ) ;
#25017=FACE_OUTER_BOUND ( 'NONE', #58288, .T. ) ;
#25021=CARTESIAN_POINT ( 'NONE',  ( 9.696433660856000003, -79.09672475065998754, 5.296892287724999981 ) ) ;
#25022=LINE ( 'NONE', #51907, #19935 ) ;
#25027=CARTESIAN_POINT ( 'NONE',  ( 5.605860879773000072, -77.45503136649999476, 9.963751779642000983 ) ) ;
#25033=CARTESIAN_POINT ( 'NONE',  ( -9.699833017908000343, -79.50094660807849323, 1.146274062705999963 ) ) ;
#25037=EDGE_LOOP ( 'NONE', ( #1817, #3459, #27496, #18361, #16018, #19828 ) ) ;
#25058=AXIS2_PLACEMENT_3D ( 'NONE', #22988, #44840, #35970 ) ;
#25061=CARTESIAN_POINT ( 'NONE',  ( -8.168740699428001406, -77.41443535657099062, 4.831335699206999124 ) ) ;
#25067=CARTESIAN_POINT ( 'NONE',  ( 7.009066229391000213, -78.45973765814899537, -6.762594642477000484 ) ) ;
#25068=EDGE_CURVE ( 'NONE', #49432, #23068, #14544, .T. ) ;
#25070=CARTESIAN_POINT ( 'NONE',  ( -11.00000000000000000, -77.70953167777609849, -1.317564550621139752 ) ) ;
#25076=CARTESIAN_POINT ( 'NONE',  ( -9.424992723873112155, -79.26013535444967317, -1.207054387620474456 ) ) ;
#25079=CARTESIAN_POINT ( 'NONE',  ( -10.41975891551938638, -80.07426127834554563, 3.525701440006863585 ) ) ;
#25080=CARTESIAN_POINT ( 'NONE',  ( 8.565252427040000782, -79.29256405623699777, -4.245882144487000076 ) ) ;
#25086=CARTESIAN_POINT ( 'NONE',  ( 7.588757936995927963E-07, -80.21583927563050054, -10.98470495943546688 ) ) ;
#25095=CARTESIAN_POINT ( 'NONE',  ( 9.233810704722001717, -79.74555105016035839, 5.933342942490105187 ) ) ;
#25102=ORIENTED_EDGE ( 'NONE', *, *, #52449, .F. ) ;
#25104=CARTESIAN_POINT ( 'NONE',  ( -11.00000000000000000, -77.69999999999998863, 0.000000000000000000 ) ) ;
#25109=CARTESIAN_POINT ( 'NONE',  ( 9.250000000000000000, -79.74999999999998579, 1.907449677260999760E-14 ) ) ;
#25117=CARTESIAN_POINT ( 'NONE',  ( 4.202209046443865503, -77.26254981315187820, -8.240357924581044102 ) ) ;
#25126=CARTESIAN_POINT ( 'NONE',  ( 10.04848221952999943, -78.77718663188798587, 4.594115663639000147 ) ) ;
#25131=CARTESIAN_POINT ( 'NONE',  ( -8.157105063561195024, -77.20000000000001705, 7.261158152830655688 ) ) ;
#25133=CYLINDRICAL_SURFACE ( 'NONE', #330, 11.00000000000000000 ) ;
#25139=CARTESIAN_POINT ( 'NONE',  ( 5.816771686847000744, -77.82035725226099032, -7.538935161885000014 ) ) ;
#25144=CARTESIAN_POINT ( 'NONE',  ( -11.00000000000000000, -78.09999999999999432, 2.733298954964999989E-14 ) ) ;
#25151=CARTESIAN_POINT ( 'NONE',  ( 9.694840914897000062, -79.58102073242298502, -5.145296513660000848 ) ) ;
#25155=FACE_OUTER_BOUND ( 'NONE', #20550, .T. ) ;
#25164=CARTESIAN_POINT ( 'NONE',  ( 5.418544735220999442, -78.07770896256499782, 9.753510481391998610 ) ) ;
#25168=CIRCLE ( 'NONE', #19522, 1.000000000000000000 ) ;
#25177=ORIENTED_EDGE ( 'NONE', *, *, #41614, .T. ) ;
#25184=CARTESIAN_POINT ( 'NONE',  ( -3.057959794837752820, -78.19827986707727518, -8.730403520994359567 ) ) ;
#25185=CARTESIAN_POINT ( 'NONE',  ( -9.250000000000003553, -79.48961838684877534, 1.206747585507256249 ) ) ;
#25187=ORIENTED_EDGE ( 'NONE', *, *, #10059, .F. ) ;
#25189=CARTESIAN_POINT ( 'NONE',  ( -5.446556518281947312, -77.52513256096960959, 7.476429722233334019 ) ) ;
#25194=CARTESIAN_POINT ( 'NONE',  ( 1.882180247600000245, -78.68961848458398833, 9.519879562373999349 ) ) ;
#25198=CARTESIAN_POINT ( 'NONE',  ( -11.11771682179999843, -80.29711170481299121, 1.751409206030000165 ) ) ;
#25210=FACE_OUTER_BOUND ( 'NONE', #3888, .T. ) ;
#25217=CARTESIAN_POINT ( 'NONE',  ( -9.309367086190000862, -77.13855160546319212, -0.1968645694141999969 ) ) ;
#25220=CARTESIAN_POINT ( 'NONE',  ( -1.861817488877999915, -80.00259998740499157, -9.461084334642999139 ) ) ;
#25223=CARTESIAN_POINT ( 'NONE',  ( -3.936406751843953167, -79.25801478680048717, 8.883122821548814940 ) ) ;
#25229=CARTESIAN_POINT ( 'NONE',  ( 10.06241996419999829, -78.08858937446798620, -4.313003509706000216 ) ) ;
#25235=CARTESIAN_POINT ( 'NONE',  ( 9.208615812369000508, -76.98427752889628550, 2.957800710608999850 ) ) ;
#25238=DIRECTION ( 'NONE',  ( 1.000000000000000000, 0.000000000000000000, 0.000000000000000000 ) ) ;
#25253=VERTEX_POINT ( 'NONE', #45705 ) ;
#25258=CARTESIAN_POINT ( 'NONE',  ( 1.210822168571075386, -79.63541666666664298, -9.249999999999996447 ) ) ;
#25259=ORIENTED_EDGE ( 'NONE', *, *, #5199, .F. ) ;
#25268=CARTESIAN_POINT ( 'NONE',  ( 6.442726462082567274, -79.66713182735726662, 7.272994535396923865 ) ) ;
#25271=CARTESIAN_POINT ( 'NONE',  ( -8.283973254211803194, -78.63679031283243148, -4.116528973202782105 ) ) ;
#25289=CIRCLE ( 'NONE', #44135, 9.250000000000000000 ) ;
#25290=DIRECTION ( 'NONE',  ( -1.000000000000000000, 0.000000000000000000, 0.000000000000000000 ) ) ;
#25300=CARTESIAN_POINT ( 'NONE',  ( 5.315453493860999856, -79.12906701255899122, -7.900401732693999257 ) ) ;
#25304=ORIENTED_EDGE ( 'NONE', *, *, #41429, .T. ) ;
#25308=CARTESIAN_POINT ( 'NONE',  ( 10.90877671396000004, -78.62684575912199136, 0.8284967960653000230 ) ) ;
#25311=CARTESIAN_POINT ( 'NONE',  ( -1.901143138367999974, -79.85477773487998832, -11.28240252173999991 ) ) ;
#25320=CARTESIAN_POINT ( 'NONE',  ( 8.193575559979001000, -79.30611065853049979, 5.316613930189999948 ) ) ;
#25329=DIRECTION ( 'NONE',  ( 1.776356839400000238E-14, -1.000000000000000000, 6.231126725709000317E-14 ) ) ;
#25336=CARTESIAN_POINT ( 'NONE',  ( 1.210822168571035418, -77.86458333333332860, 9.250000000000007105 ) ) ;
#25341=CARTESIAN_POINT ( 'NONE',  ( 0.000000000000000000, -78.69999999999998863, 0.000000000000000000 ) ) ;
#25350=CARTESIAN_POINT ( 'NONE',  ( 2.878019135186999922, -77.91968490469898256, -9.304660206797001010 ) ) ;
#25351=CIRCLE ( 'NONE', #58360, 4.100000000000000533 ) ;
#25353=CARTESIAN_POINT ( 'NONE',  ( 0.000000000000000000, -77.19999999999998863, 0.000000000000000000 ) ) ;
#25359=CARTESIAN_POINT ( 'NONE',  ( -6.339110262596877376, -79.18297630452198632, 7.102346778884022882 ) ) ;
#25361=CARTESIAN_POINT ( 'NONE',  ( 2.580008266957357410, -80.00000000000000000, -9.145130960450376989 ) ) ;
#25364=CARTESIAN_POINT ( 'NONE',  ( -0.09919819565124000926, -79.89501551942399260, -9.890690074140000121 ) ) ;
#25366=CARTESIAN_POINT ( 'NONE',  ( -2.421167930323333106, -79.10416666666664298, -9.009247259181917045 ) ) ;
#25381=CARTESIAN_POINT ( 'NONE',  ( -7.479908383216000267, -79.26513030413099159, -6.281056869080000382 ) ) ;
#25389=DIRECTION ( 'NONE',  ( 1.000000000000000000, 0.000000000000000000, 0.000000000000000000 ) ) ;
#25398=CARTESIAN_POINT ( 'NONE',  ( 4.912554240050883259, -79.93092688505531385, 7.839266877745309614 ) ) ;
#25401=CARTESIAN_POINT ( 'NONE',  ( -9.254388464354001087, -79.90752053325199711, 5.469807505829999528 ) ) ;
#25403=CARTESIAN_POINT ( 'NONE',  ( 1.728979404161999911, -78.48355279846498433, 11.13281482770999986 ) ) ;
#25404=CARTESIAN_POINT ( 'NONE',  ( 8.871203788894485243, -77.32666406881654098, -2.694563217664684096 ) ) ;
#25408=UNCERTAINTY_MEASURE_WITH_UNIT (LENGTH_MEASURE( 1.000000000000000082E-05 ), #48490, 'distance_accuracy_value', 'NONE');
#25418=CARTESIAN_POINT ( 'NONE',  ( -7.558619072263999428, -79.05811017521499195, -8.058856703501000140 ) ) ;
#25431=CARTESIAN_POINT ( 'NONE',  ( -7.068247108407000212, -78.70149595525998620, -6.380459158363000149 ) ) ;
#25437=CARTESIAN_POINT ( 'NONE',  ( 1.210822168571035418, -78.86458333333334281, 9.250000000000007105 ) ) ;
#25441=CARTESIAN_POINT ( 'NONE',  ( 6.718030245586000149, -79.04726600010199888, -8.679405866825000260 ) ) ;
#25443=CARTESIAN_POINT ( 'NONE',  ( -9.416284655759811884, -80.42395833333223720, 5.426231776061239742 ) ) ;
#25446=DIRECTION ( 'NONE',  ( -3.675131323893999047E-09, -0.9999999999999997780, 2.168720883760999791E-08 ) ) ;
#25452=CARTESIAN_POINT ( 'NONE',  ( -7.805809014822999714, -79.61509741874499468, 8.123945268076997905 ) ) ;
#25456=CIRCLE ( 'NONE', #57476, 1.200000000000000622 ) ;
#25460=DIRECTION ( 'NONE',  ( 0.000000000000000000, 1.000000000000000000, 0.000000000000000000 ) ) ;
#25477=CARTESIAN_POINT ( 'NONE',  ( -5.786494162132466812, -77.52886857143271016, 7.216877617947186963 ) ) ;
#25479=CARTESIAN_POINT ( 'NONE',  ( 11.00000000000000000, -78.34999999999999432, 0.000000000000000000 ) ) ;
#25480=CARTESIAN_POINT ( 'NONE',  ( -8.073459667400001649, -78.37695636416498246, -5.384232384047000330 ) ) ;
#25484=CARTESIAN_POINT ( 'NONE',  ( -9.459258931978000717, -79.76813694385799636, 5.442530770145999952 ) ) ;
#25493=CARTESIAN_POINT ( 'NONE',  ( 9.250000000000000000, -78.34999999999999432, 0.000000000000000000 ) ) ;
#25497=CARTESIAN_POINT ( 'NONE',  ( -10.92178492054000039, -80.01025540420299365, -2.397173661657999943 ) ) ;
#25509=CARTESIAN_POINT ( 'NONE',  ( -0.4755896768997000534, -79.33590927173898422, 9.521775672420998760 ) ) ;
#25516=CARTESIAN_POINT ( 'NONE',  ( -10.05598257587000077, -77.40315636649998510, -4.328040802368000151 ) ) ;
#25521=CARTESIAN_POINT ( 'NONE',  ( -2.880544446985999762, -76.81021508244178619, -9.112186890989001142 ) ) ;
#25522=CARTESIAN_POINT ( 'NONE',  ( -2.421167930323349982, -78.39583333333332860, 9.009247259181918821 ) ) ;
#25523=CARTESIAN_POINT ( 'NONE',  ( 10.99999999999999645, -77.36041666666666572, 1.439896632895345974 ) ) ;
#25528=ORIENTED_EDGE ( 'NONE', *, *, #10383, .T. ) ;
#25534=AXIS2_PLACEMENT_3D ( 'NONE', #47631, #23479, #38733 ) ;
#25558=CARTESIAN_POINT ( 'NONE',  ( -9.230872287500126561, -78.60521422558908000, -0.6021493626502718577 ) ) ;
#25575=VECTOR ( 'NONE', #14703, 1000.000000000000114 ) ;
#25576=CARTESIAN_POINT ( 'NONE',  ( -10.44304457033000055, -78.28465421611399222, 3.377400876517000050 ) ) ;
#25577=CARTESIAN_POINT ( 'NONE',  ( -9.497876546326999403, -77.35168256874098347, -0.2008509664869000122 ) ) ;
#25586=CARTESIAN_POINT ( 'NONE',  ( 9.085337660295000006, -78.73113340475299538, 2.850792140868000146 ) ) ;
#25593=CARTESIAN_POINT ( 'NONE',  ( -7.367791399714448630, -79.04847752305433062, 5.626431170726755582 ) ) ;
#25596=CARTESIAN_POINT ( 'NONE',  ( -7.655192530954000318, -79.74284890031098882, 7.967190206674000130 ) ) ;
#25598=CARTESIAN_POINT ( 'NONE',  ( -11.19194202533000038, -80.29450396371099430, 1.763102137848999940 ) ) ;
#25605=CARTESIAN_POINT ( 'NONE',  ( 9.630577183392999174, -79.39349084372300069, 1.628483183780000010 ) ) ;
#25645=CARTESIAN_POINT ( 'NONE',  ( -9.478081404219775408, -79.25540238611779387, -0.6444716196238855499 ) ) ;
#25649=CARTESIAN_POINT ( 'NONE',  ( -4.178495327992000519, -80.18134756606798419, 8.699161539798998533 ) ) ;
#25653=DIRECTION ( 'NONE',  ( 0.000000000000000000, 0.000000000000000000, -1.000000000000000000 ) ) ;
#25669=AXIS2_PLACEMENT_3D ( 'NONE', #29927, #7514, #39092 ) ;
#25677=CARTESIAN_POINT ( 'NONE',  ( 2.879226727952050258, -77.55416666666666003, 10.71369944335148361 ) ) ;
#25685=CARTESIAN_POINT ( 'NONE',  ( -0.7292915032463275216, -79.98137597068046034, 9.221144000337346824 ) ) ;
#25687=CARTESIAN_POINT ( 'NONE',  ( 0.7246619768400597295, -80.32015672653835736, 11.08451829927562926 ) ) ;
#25690=CARTESIAN_POINT ( 'NONE',  ( 5.455175217613329686, -77.27533145166849238, -7.470068744196724175 ) ) ;
#25697=CARTESIAN_POINT ( 'NONE',  ( 1.000000000000000000, -81.99999999999998579, -7.000000000000000000 ) ) ;
#25700=CARTESIAN_POINT ( 'NONE',  ( -5.850594862776000049, -78.47586176634699484, 9.500638896661000032 ) ) ;
#25717=CARTESIAN_POINT ( 'NONE',  ( 7.184025905720999639, -77.27327641628599508, -6.082841960620999799 ) ) ;
#25728=CARTESIAN_POINT ( 'NONE',  ( -4.277738290159001089, -78.96298893710398659, -10.10766895494000117 ) ) ;
#25733=VERTEX_POINT ( 'NONE', #30201 ) ;
#25736=CARTESIAN_POINT ( 'NONE',  ( 1.210822168571049851, -78.13541666666667140, -9.250000000000003553 ) ) ;
#25737=CARTESIAN_POINT ( 'NONE',  ( 8.348568777154000031, -77.93724719090198505, -7.051780313135000533 ) ) ;
#25740=CARTESIAN_POINT ( 'NONE',  ( 0.000000000000000000, -81.19999999999998863, 7.000000000000000000 ) ) ;
#25758=CARTESIAN_POINT ( 'NONE',  ( -4.696659842484057101, -79.66604136332699682, 8.289744325010493853 ) ) ;
#25765=CARTESIAN_POINT ( 'NONE',  ( 0.3345645958933402553, -78.22793362420514995, -9.244204907905819724 ) ) ;
#25769=CARTESIAN_POINT ( 'NONE',  ( -7.491156050946263356, -77.55010980111761398, 5.426323088073407241 ) ) ;
#25770=CARTESIAN_POINT ( 'NONE',  ( -9.050627908549000011, -77.41837041848599199, -6.322205650057999726 ) ) ;
#25773=CARTESIAN_POINT ( 'NONE',  ( 9.583411031200000707, -78.09271807287498746, 1.526087275887999972 ) ) ;
#25776=CARTESIAN_POINT ( 'NONE',  ( -11.09141466634999951, -79.91658357209098540, 1.909950515085000022 ) ) ;
#25779=ORIENTED_EDGE ( 'NONE', *, *, #2515, .T. ) ;
#25786=CARTESIAN_POINT ( 'NONE',  ( 8.083193604682708866, -79.39173883515665864, 4.658712740633392357 ) ) ;
#25789=CARTESIAN_POINT ( 'NONE',  ( -9.191308745188409901, -79.61083708887171895, -1.210837173519272447 ) ) ;
#25797=CARTESIAN_POINT ( 'NONE',  ( 6.028278362248999933, -79.27746395522298428, 7.385810467003000035 ) ) ;
#25806=CARTESIAN_POINT ( 'NONE',  ( -8.579474846409000932, -77.31747724050399029, 6.800540979835000499 ) ) ;
#25825=EDGE_LOOP ( 'NONE', ( #4501, #27402, #3680, #17078 ) ) ;
#25865=EDGE_CURVE ( 'NONE', #37493, #23736, #28004, .T. ) ;
#25866=CARTESIAN_POINT ( 'NONE',  ( -9.414505844818329194, -77.40158925224952213, -0.1990887029408508757 ) ) ;
#25874=CARTESIAN_POINT ( 'NONE',  ( 7.742244746672000133, -79.15749084168798788, -5.543281135378999913 ) ) ;
#25879=CARTESIAN_POINT ( 'NONE',  ( 8.796335266379967877, -78.89791666666668846, -6.760013919724086051 ) ) ;
#25883=CARTESIAN_POINT ( 'NONE',  ( 0.9061038674864000386, -78.73921517645298707, 10.90260483175000061 ) ) ;
#25885=CARTESIAN_POINT ( 'NONE',  ( -7.031693321690999809, -80.44190203517098325, -8.741081632921000377 ) ) ;
#25898=CARTESIAN_POINT ( 'NONE',  ( -2.600000000000000089, -77.49999999999998579, 0.000000000000000000 ) ) ;
#25907=CARTESIAN_POINT ( 'NONE',  ( 9.124907197977810469, -78.83697965493469439, -1.519474258559118329 ) ) ;
#25913=DIRECTION ( 'NONE',  ( 3.675126883001999395E-09, -0.9999999999999997780, -2.168720882565999754E-08 ) ) ;
#25919=CARTESIAN_POINT ( 'NONE',  ( 7.333430185446000671, -77.21721742767299190, -5.851948249255000789 ) ) ;
#25924=CARTESIAN_POINT ( 'NONE',  ( 9.250000000000000000, -78.84999999999999432, 1.340711541092999922E-14 ) ) ;
#25933=CARTESIAN_POINT ( 'NONE',  ( 7.093757948711532535, -79.05808181110914745, 6.348225669172625096 ) ) ;
#25935=CARTESIAN_POINT ( 'NONE',  ( -5.539808784079933268, -79.01666666666669414, 9.611650271896811759 ) ) ;
#25938=CARTESIAN_POINT ( 'NONE',  ( 8.780551327949000395, -79.55888659510199545, 4.553845519790999496 ) ) ;
#25940=CARTESIAN_POINT ( 'NONE',  ( 0.000000000000000000, -74.64999999999999147, 0.000000000000000000 ) ) ;
#25943=AXIS2_PLACEMENT_3D ( 'NONE', #57804, #56663, #34197 ) ;
#25949=ORIENTED_EDGE ( 'NONE', *, *, #2432, .T. ) ;
#25955=CARTESIAN_POINT ( 'NONE',  ( -4.373213035511999358, -79.41820881373098473, -8.733596771889999388 ) ) ;
#25963=CARTESIAN_POINT ( 'NONE',  ( -9.611650271896857944, -77.65833333333331723, 5.539808784079855997 ) ) ;
#25971=CARTESIAN_POINT ( 'NONE',  ( -0.7414790400310934393, -79.98147823536180567, 9.220178373586891851 ) ) ;
#25974=CARTESIAN_POINT ( 'NONE',  ( 5.874297357630430483, -77.27991952769977502, -7.146146602706561879 ) ) ;
#25978=CIRCLE ( 'NONE', #15632, 1.199999999999999734 ) ;
#25983=DIRECTION ( 'NONE',  ( 0.000000000000000000, 0.000000000000000000, -1.000000000000000000 ) ) ;
#25984=CARTESIAN_POINT ( 'NONE',  ( -7.035077178968999867, -79.62764829398598465, -8.660212973301998574 ) ) ;
#25991=CARTESIAN_POINT ( 'NONE',  ( 3.321932689531000182, -77.19999999999998863, 10.22385755016999909 ) ) ;
#26009=CARTESIAN_POINT ( 'NONE',  ( -3.548303639235999896, -79.52895424076298525, -10.38621961377000069 ) ) ;
#26017=CARTESIAN_POINT ( 'NONE',  ( 8.796335266379994522, -77.79791666666667993, -6.760013919724047859 ) ) ;
#26018=CARTESIAN_POINT ( 'NONE',  ( -3.734118835908999845, -79.14521842720699851, 10.51417881607000027 ) ) ;
#26019=ADVANCED_FACE ( 'NONE', ( #41698 ), #53338, .T. ) ;
#26031=EDGE_CURVE ( 'NONE', #2177, #6475, #14694, .T. ) ;
#26036=CARTESIAN_POINT ( 'NONE',  ( -9.578019072079097640, -79.75346114563041056, -0.4234131151099537749 ) ) ;
#26042=CARTESIAN_POINT ( 'NONE',  ( -4.265506261528114962, -78.18699093222700469, -8.208995969611063259 ) ) ;
#26044=ORIENTED_EDGE ( 'NONE', *, *, #21945, .T. ) ;
#26046=CARTESIAN_POINT ( 'NONE',  ( -7.039186935347679253, -77.54390228458088075, 6.000959365781699084 ) ) ;
#26049=CARTESIAN_POINT ( 'NONE',  ( 5.417083560473000325, -79.00228060500298000, -8.051455326762999576 ) ) ;
#26053=CARTESIAN_POINT ( 'NONE',  ( -8.254612054926999676, -79.81451948108198735, 6.886499823760000361 ) ) ;
#26056=CARTESIAN_POINT ( 'NONE',  ( -5.684557159767956058, -78.57291666666664298, -7.396918292183169541 ) ) ;
#26062=CIRCLE ( 'NONE', #23258, 11.00000000000000000 ) ;
#26076=CARTESIAN_POINT ( 'NONE',  ( -2.858407197967999913, -77.19999999999998863, -8.797272775729998884 ) ) ;
#26079=CARTESIAN_POINT ( 'NONE',  ( 4.318672206561768867, -77.60826495664210256, -9.868970905821345951 ) ) ;
#26080=CARTESIAN_POINT ( 'NONE',  ( -9.071080135827999769, -80.04268349419798767, -2.557679440262000448 ) ) ;
#26087=CARTESIAN_POINT ( 'NONE',  ( -2.879226727952071574, -77.30416666666666003, -10.71369944335147473 ) ) ;
#26089=DIRECTION ( 'NONE',  ( 0.000000000000000000, 1.000000000000000000, 0.000000000000000000 ) ) ;
#26094=CARTESIAN_POINT ( 'NONE',  ( -9.555818165766000405, -77.21055870928698539, -0.1257991660602000017 ) ) ;
#26114=CARTESIAN_POINT ( 'NONE',  ( -9.254189652385859333, -79.84085386658529160, 5.469689899798553689 ) ) ;
#26120=CARTESIAN_POINT ( 'NONE',  ( -3.203604947276998960, -77.74842935028665636, 10.56508708802999941 ) ) ;
#26123=ORIENTED_EDGE ( 'NONE', *, *, #12471, .F. ) ;
#26155=CARTESIAN_POINT ( 'NONE',  ( -8.058638732054999920, -78.36893127911199031, -7.451332657186999775 ) ) ;
#26165=CARTESIAN_POINT ( 'NONE',  ( 4.510926502723999754, -77.72927130271399676, 8.509098192649000580 ) ) ;
#26172=CARTESIAN_POINT ( 'NONE',  ( -8.956130479881542428, -79.07960960748528123, 2.390097164946143327 ) ) ;
#26177=CARTESIAN_POINT ( 'NONE',  ( -0.5177219211888000050, -78.99204636544698133, -10.92793577709999830 ) ) ;
#26179=CARTESIAN_POINT ( 'NONE',  ( -7.000000000000000000, -81.10000000285099020, 0.000000000000000000 ) ) ;
#26198=CARTESIAN_POINT ( 'NONE',  ( 9.177871051388377666, -78.84012010996477215, -1.162879483702742744 ) ) ;
#26205=CARTESIAN_POINT ( 'NONE',  ( 0.000000000000000000, -81.19999999999998863, -7.000000000000000000 ) ) ;
#26206=CARTESIAN_POINT ( 'NONE',  ( 7.137508353459041111, -79.91917351108399714, 8.454853940648142441 ) ) ;
#26207=ADVANCED_FACE ( 'NONE', ( #13203, #35636 ), #45114, .T. ) ;
#26210=CARTESIAN_POINT ( 'NONE',  ( -0.8247866532291000530, -77.07501358598499053, -9.454605849501000137 ) ) ;
#26211=DIRECTION ( 'NONE',  ( -1.000000000000000000, 0.000000000000000000, 0.000000000000000000 ) ) ;
#26214=FACE_OUTER_BOUND ( 'NONE', #10741, .T. ) ;
#26228=CARTESIAN_POINT ( 'NONE',  ( 7.129854210758000299, -80.08175381071399102, 6.855691147963000276 ) ) ;
#26239=B_SPLINE_CURVE_WITH_KNOTS ( 'NONE', 3,
 ( #12967, #8263, #53423, #2973, #21259, #52279, #26543, #34823, #44569, #25971, #47866, #25685, #7396, #26263, #34244, #39264, #30966, #57853, #17120, #12117, #52851, #48153, #43712, #4124, #35105, #7973, #30395, #48431, #3267, #43997, #3547, #38688, #44276, #43415, #3835, #21832, #39555, #57559, #53139, #39838, #17410, #56708, #12687, #30680, #29815, #16265, #48718, #16550, #25398, #7684, #20972, #56988, #30102, #44870, #4423, #35699, #22124, #54318, #54022, #22720, #5007, #40733, #13858, #26, #14145, #32144, #40135, #13564, #31554, #17714, #614, #45171, #50183, #18006, #53728, #18878, #10026, #35997, #9729, #4721, #9149, #40436, #31854, #49895, #9439, #22423, #45465, #324, #18302, #54607, #13267, #27133, #31258, #49300, #36295, #41312, #8851, #28007, #27430, #49602, #23012, #45762, #18596, #26841, #23304, #27718, #5296, #41023, #36585, #897, #36874 ),
 .UNSPECIFIED., .F., .F.,
 ( 4, 2, 2, 2, 1, 1, 1, 1, 1, 2, 2, 2, 2, 2, 1, 1, 1, 1, 1, 2, 2, 2, 2, 2, 1, 1, 1, 1, 1, 2, 2, 2, 2, 2, 1, 1, 1, 1, 1, 2, 2, 2, 2, 2, 1, 1, 1, 1, 1, 2, 2, 2, 2, 2, 1, 1, 1, 1, 1, 2, 2, 2, 2, 2, 1, 1, 1, 1, 1, 2, 2, 2, 4 ),
 ( 0.000000000000000000, 0.06249999999997328526, 0.09374999999995992095, 0.1093749999999532596, 0.1171874999999499428, 0.1210937499999483052, 0.1230468749999474448, 0.1240234374999469730, 0.1245117187499466260, 0.1247558593749464040, 0.1249999999999461681, 0.1874999999998897826, 0.2187499999998615552, 0.2343749999998474831, 0.2421874999998404610, 0.2460937499998369360, 0.2480468749998351596, 0.2490234374998342437, 0.2495117187498337996, 0.2497558593748335498, 0.2499999999998333000, 0.3124999999997782330, 0.3437499999997506439, 0.3593749999997368216, 0.3671874999997298827, 0.3710937499997263855, 0.3730468749997248867, 0.3740234374997239430, 0.3745117187497231659, 0.3747558593747231104, 0.3749999999997231104, 0.4374999999997050137, 0.4687499999996960764, 0.4843749999996914135, 0.4921874999996889710, 0.4960937499996877498, 0.4980468749996871392, 0.4990234374996866396, 0.4995117187496862510, 0.4997558593746861955, 0.4999999999996861400, 0.5624999999996663780, 0.5937499999996566080, 0.6093749999996517230, 0.6171874999996492805, 0.6210937499996478373, 0.6230468749996470601, 0.6240234374996471711, 0.6245117187496469491, 0.6247558593746470601, 0.6249999999996471711, 0.6874999999996908029, 0.7187499999997127853, 0.7343749999997238875, 0.7421874999997295497, 0.7460937499997323252, 0.7480468749997337685, 0.7490234374997345457, 0.7495117187497348787, 0.7497558593747349898, 0.7499999999997351008, 0.8124999999997707389, 0.8437499999997886135, 0.8593749999997974953, 0.8671874999998018252, 0.8710937499998042677, 0.8730468749998057110, 0.8740234374998065991, 0.8745117187498072653, 0.8747558593748075983, 0.8749999999998079314, 0.9374999999999040767, 1.000000000000000000 ),
 .UNSPECIFIED. ) ;
#26246=CARTESIAN_POINT ( 'NONE',  ( -4.465297566879000257, -79.68263247063998733, 8.686876450551999085 ) ) ;
#26249=B_SPLINE_CURVE_WITH_KNOTS ( 'NONE', 3,
 ( #45486, #5030, #50204, #23032, #36317, #9753, #4150, #31875, #45193, #27739 ),
 .UNSPECIFIED., .F., .F.,
 ( 4, 2, 2, 2, 4 ),
 ( 0.2499999978686767710, 0.4374999984015075505, 0.6249999989343384410, 0.8124999994671692205, 1.000000000000000000 ),
 .UNSPECIFIED. ) ;
#26253=ORIENTED_EDGE ( 'NONE', *, *, #30923, .F. ) ;
#26263=CARTESIAN_POINT ( 'NONE',  ( -0.7267300686164063217, -79.98135465499143493, 9.221345538712327539 ) ) ;
#26266=CARTESIAN_POINT ( 'NONE',  ( 2.618044012240999585, -78.76447634179098145, -10.95786383906999895 ) ) ;
#26275=DIRECTION ( 'NONE',  ( 0.000000000000000000, 1.000000000000000000, 0.000000000000000000 ) ) ;
#26276=CARTESIAN_POINT ( 'NONE',  ( -10.64215094251999894, -79.97579375008199065, 2.340290094375000240 ) ) ;
#26292=CARTESIAN_POINT ( 'NONE',  ( -7.696817093642000174, -77.59296661922998339, 5.606191475415999825 ) ) ;
#26301=CARTESIAN_POINT ( 'NONE',  ( 3.176617583302000281, -79.78178542975699372, 10.50586082162000068 ) ) ;
#26308=CARTESIAN_POINT ( 'NONE',  ( 7.054366762047179940, -77.30619333359085488, 6.026930045153958027 ) ) ;
#26309=CARTESIAN_POINT ( 'NONE',  ( -6.760013919724058518, -77.67291666666665151, -8.796335266379987416 ) ) ;
#26311=CARTESIAN_POINT ( 'NONE',  ( -2.183649677207000206, -78.19776941201399723, 10.83095413486000069 ) ) ;
#26321=ORIENTED_EDGE ( 'NONE', *, *, #40478, .T. ) ;
#26322=DIRECTION ( 'NONE',  ( -1.000000000000000000, 0.000000000000000000, 0.000000000000000000 ) ) ;
#26330=CARTESIAN_POINT ( 'NONE',  ( -5.095949825044894688, -78.17859843627216776, -7.719699935279118463 ) ) ;
#26334=CARTESIAN_POINT ( 'NONE',  ( -4.209169930338003240, -77.51272233025383684, 8.236736021501149807 ) ) ;
#26335=CARTESIAN_POINT ( 'NONE',  ( 10.42639159904000046, -77.03997040616140168, -2.617796444239999687 ) ) ;
#26336=CARTESIAN_POINT ( 'NONE',  ( -0.5548610165507998904, -78.01090185290100010, -9.688283574444998436 ) ) ;
#26340=CARTESIAN_POINT ( 'NONE',  ( 3.942135768300999654, -80.14393115911698828, -10.54187931140000067 ) ) ;
#26354=CARTESIAN_POINT ( 'NONE',  ( 0.7366363428794999724, -80.42674279837198981, 11.26767966793000042 ) ) ;
#26362=EDGE_CURVE ( 'NONE', #54466, #15959, #45945, .T. ) ;
#26377=CARTESIAN_POINT ( 'NONE',  ( 9.670530767802999250, -77.13907693894029194, -0.1674091926992999912 ) ) ;
#26388=ORIENTED_EDGE ( 'NONE', *, *, #56057, .F. ) ;
#26404=VERTEX_POINT ( 'NONE', #40969 ) ;
#26409=CARTESIAN_POINT ( 'NONE',  ( 0.8618009059429999619, -78.34162200021098954, -9.665816497589000633 ) ) ;
#26412=FACE_BOUND ( 'NONE', #20788, .T. ) ;
#26416=CARTESIAN_POINT ( 'NONE',  ( -9.179332505514366858, -78.61010642507874024, -1.157977033747941809 ) ) ;
#26428=CARTESIAN_POINT ( 'NONE',  ( -6.760013919724056741, -79.27291666666666003, -8.796335266379987416 ) ) ;
#26432=EDGE_CURVE ( 'NONE', #52835, #11445, #19409, .T. ) ;
#26437=FACE_OUTER_BOUND ( 'NONE', #35310, .T. ) ;
#26441=CARTESIAN_POINT ( 'NONE',  ( -9.504204889957000191, -77.45206109394898419, 0.5832244475350000235 ) ) ;
#26447=CARTESIAN_POINT ( 'NONE',  ( -9.250265637099717608, -79.09517564970080628, 0.6034143313266543407 ) ) ;
#26452=CARTESIAN_POINT ( 'NONE',  ( 6.657089793739999983, -79.63047948297999312, 8.818222636911000833 ) ) ;
#26454=CARTESIAN_POINT ( 'NONE',  ( -11.30204317227000033, -80.23062822292799012, 1.780446720864000021 ) ) ;
#26457=ORIENTED_EDGE ( 'NONE', *, *, #24298, .F. ) ;
#26459=EDGE_CURVE ( 'NONE', #46260, #30832, #25978, .T. ) ;
#26466=EDGE_LOOP ( 'NONE', ( #39410, #27353, #40357 ) ) ;
#26474=DIRECTION ( 'NONE',  ( 0.000000000000000000, -1.000000000000000000, 0.000000000000000000 ) ) ;
#26484=CARTESIAN_POINT ( 'NONE',  ( 9.469145113845355510, -79.89323344442750852, 5.723973398464533346 ) ) ;
#26496=DIRECTION ( 'NONE',  ( -1.000000000000000000, 0.000000000000000000, 0.000000000000000000 ) ) ;
#26506=CARTESIAN_POINT ( 'NONE',  ( 8.682512087609998375, -79.49501085431899128, 4.502999560499000076 ) ) ;
#26527=CARTESIAN_POINT ( 'NONE',  ( 9.523132023602000729, -80.08931041772898141, 1.108936319727999997 ) ) ;
#26543=CARTESIAN_POINT ( 'NONE',  ( -0.8350858585606752982, -79.98228243800841142, 9.212292648074781098 ) ) ;
#26546=CARTESIAN_POINT ( 'NONE',  ( -1.331888048429999971, -78.73638398745899281, -11.18726993471000064 ) ) ;
#26553=CARTESIAN_POINT ( 'NONE',  ( 9.458764864882999390, -79.26244768766198945, -5.918054316060000097 ) ) ;
#26562=AXIS2_PLACEMENT_3D ( 'NONE', #15177, #6026, #55626 ) ;
#26568=CARTESIAN_POINT ( 'NONE',  ( -9.088317367618000020, -78.68010020865598619, 3.186800494491000002 ) ) ;
#26573=CARTESIAN_POINT ( 'NONE',  ( 0.000000000000000000, -76.39999999999999147, -10.70000000000050910 ) ) ;
#26578=CARTESIAN_POINT ( 'NONE',  ( 6.718030245586000149, -79.10756892577299482, -8.679405866825000260 ) ) ;
#26582=CARTESIAN_POINT ( 'NONE',  ( -9.250000000000000000, -77.49999999999998579, -1.203901273580999948E-14 ) ) ;
#26583=VERTEX_POINT ( 'NONE', #2288 ) ;
#26586=CARTESIAN_POINT ( 'NONE',  ( 0.000000000000000000, -80.49999999999998579, 0.000000000000000000 ) ) ;
#26589=CARTESIAN_POINT ( 'NONE',  ( -9.975891578018998729, -78.78001782088199434, -4.997317968730000004 ) ) ;
#26606=EDGE_CURVE ( 'NONE', #55023, #43973, #28972, .T. ) ;
#26608=CARTESIAN_POINT ( 'NONE',  ( -4.760515938158666138, -78.18205582176251767, -7.931580567799660031 ) ) ;
#26615=CARTESIAN_POINT ( 'NONE',  ( 1.923959828134896410, -77.45840880865959832, 9.047739647329839485 ) ) ;
#26616=CARTESIAN_POINT ( 'NONE',  ( 10.74764839381999870, -78.05788108345298326, -0.2248421733643000131 ) ) ;
#26618=CARTESIAN_POINT ( 'NONE',  ( 9.045658679128999680, -79.16680423747999384, 3.115350657311999782 ) ) ;
#26623=CARTESIAN_POINT ( 'NONE',  ( -1.635010352784000087, -80.60330397784099432, -10.62493487727000030 ) ) ;
#26624=AXIS2_PLACEMENT_3D ( 'NONE', #7641, #47546, #38072 ) ;
#26635=CARTESIAN_POINT ( 'NONE',  ( 4.658432487275518064, -78.43336646302013548, 8.082308736674995941 ) ) ;
#26638=CARTESIAN_POINT ( 'NONE',  ( -11.15381322820999976, -80.61990947872999413, 0.1149043147075999999 ) ) ;
#26642=CARTESIAN_POINT ( 'NONE',  ( 9.611650271896829523, -79.99166666667116488, 5.539808784079915505 ) ) ;
#26648=CARTESIAN_POINT ( 'NONE',  ( 8.278055182862001260, -79.24824129696499142, 4.729100463561999312 ) ) ;
#26664=CARTESIAN_POINT ( 'NONE',  ( 7.714905556308770507, -79.55033101189913225, -5.543136766205470245 ) ) ;
#26666=B_SPLINE_CURVE_WITH_KNOTS ( 'NONE', 3,
 ( #29366, #25523, #20527, #39396, #30233, #15804, #39104, #56831, #47990, #11677, #48276, #7812, #56254, #29652, #2813, #51834, #12242, #38814 ),
 .UNSPECIFIED., .F., .F.,
 ( 4, 2, 2, 2, 2, 2, 2, 2, 4 ),
 ( 0.000000000000000000, 0.1249999999999999445, 0.2499999999999998890, 0.3749999999999999445, 0.5000000000000000000, 0.6250000000000000000, 0.7500000000000001110, 0.8750000000000000000, 1.000000000000000000 ),
 .UNSPECIFIED. ) ;
#26679=ORIENTED_EDGE ( 'NONE', *, *, #11036, .F. ) ;
#26685=CARTESIAN_POINT ( 'NONE',  ( 3.942135768300999654, -80.00347729592307644, -10.54187931140000067 ) ) ;
#26692=CARTESIAN_POINT ( 'NONE',  ( -11.00724581733999941, -77.84385847628304589, 0.8512868710715000287 ) ) ;
#26701=CARTESIAN_POINT ( 'NONE',  ( 8.553489385229999797, -78.99537007017698897, 4.133741566275999979 ) ) ;
#26723=CARTESIAN_POINT ( 'NONE',  ( -11.00000000000000000, -79.21041666666666003, -1.439896632895322881 ) ) ;
#26734=CARTESIAN_POINT ( 'NONE',  ( -8.517419447173999458, -77.42363726481998754, 3.788002893487000033 ) ) ;
#26744=EDGE_LOOP ( 'NONE', ( #33388, #31988, #21460 ) ) ;
#26745=CARTESIAN_POINT ( 'NONE',  ( -9.475012188928999990, -79.32915461743898788, 5.469182786826999987 ) ) ;
#26756=CARTESIAN_POINT ( 'NONE',  ( -8.448510849392999233, -79.70817963672152473, 4.901364000006999788 ) ) ;
#26757=EDGE_LOOP ( 'NONE', ( #39824, #57528, #26816, #3468 ) ) ;
#26772=CARTESIAN_POINT ( 'NONE',  ( 8.082447335412272338, -77.80849359151311262, -4.658563211049076003 ) ) ;
#26779=CARTESIAN_POINT ( 'NONE',  ( -8.861449449424647185, -80.04887384436648290, 6.625956105248708816 ) ) ;
#26791=CARTESIAN_POINT ( 'NONE',  ( 10.61050599188999932, -78.32876026662599145, -2.901234667509999809 ) ) ;
#26803=CARTESIAN_POINT ( 'NONE',  ( 6.760013919724039866, -78.92291666666670835, 8.796335266379998075 ) ) ;
#26804=CARTESIAN_POINT ( 'NONE',  ( 5.110488341091000031, -78.66022958144499455, 8.291116005822999568 ) ) ;
#26811=CARTESIAN_POINT ( 'NONE',  ( -2.935661446561999899, -76.94999999999998863, -9.035036904803998681 ) ) ;
#26815=CIRCLE ( 'NONE', #8923, 11.00000000000000000 ) ;
#26816=ORIENTED_EDGE ( 'NONE', *, *, #410, .F. ) ;
#26817=EDGE_CURVE ( 'NONE', #58355, #51020, #50853, .T. ) ;
#26819=DIRECTION ( 'NONE',  ( -1.000000000000000000, 0.000000000000000000, 0.000000000000000000 ) ) ;
#26821=ORIENTED_EDGE ( 'NONE', *, *, #4135, .F. ) ;
#26824=CARTESIAN_POINT ( 'NONE',  ( -8.396223008680999911, -79.87282602934199360, -4.990405176070999538 ) ) ;
#26834=CARTESIAN_POINT ( 'NONE',  ( 1.260662490416350812, -77.71453862646123412, 9.622086981278945572 ) ) ;
#26841=CARTESIAN_POINT ( 'NONE',  ( 8.994003557245340730, -79.86886930543070662, 2.160818744066264951 ) ) ;
#26853=CARTESIAN_POINT ( 'NONE',  ( 11.05620287758999964, -79.79620241998199504, -1.500659051079999973 ) ) ;
#26869=CARTESIAN_POINT ( 'NONE',  ( -7.562571750566999818, -77.19503301142388807, -5.786002763631000079 ) ) ;
#26876=CARTESIAN_POINT ( 'NONE',  ( 9.249999999999998224, -78.76041666666667140, 1.210822168571084934 ) ) ;
#26881=CARTESIAN_POINT ( 'NONE',  ( 10.28103400416999946, -78.26891651279798623, 3.842432268884000024 ) ) ;
#26882=CARTESIAN_POINT ( 'NONE',  ( 5.539808784079871984, -79.26666666666666572, -9.611650271896849063 ) ) ;
#26886=VERTEX_POINT ( 'NONE', #38721 ) ;
#26892=CARTESIAN_POINT ( 'NONE',  ( 9.458764864882999390, -78.94857194687799051, -5.918054316060000097 ) ) ;
#26900=VERTEX_POINT ( 'NONE', #25144 ) ;
#26905=CARTESIAN_POINT ( 'NONE',  ( -8.834209325778934030, -79.71953728951929463, 3.560217370319449071 ) ) ;
#26915=CARTESIAN_POINT ( 'NONE',  ( 4.449028115235954317, -77.43534773065439936, 8.140145073587429891 ) ) ;
#26916=CARTESIAN_POINT ( 'NONE',  ( 1.160587285869999929, -77.79677043080998544, 10.97894289003999901 ) ) ;
#26918=CARTESIAN_POINT ( 'NONE',  ( -6.766389538252999714, -77.95405419464299257, -6.956053621355001049 ) ) ;
#26926=DIRECTION ( 'NONE',  ( 0.000000000000000000, 0.000000000000000000, -1.000000000000000000 ) ) ;
#26928=ORIENTED_EDGE ( 'NONE', *, *, #2515, .F. ) ;
#26936=CARTESIAN_POINT ( 'NONE',  ( 9.284235709610999976, -80.42009620847800022, 6.618340736769000365 ) ) ;
#26954=DIRECTION ( 'NONE',  ( 0.000000000000000000, -1.000000000000000000, 0.000000000000000000 ) ) ;
#26980=CARTESIAN_POINT ( 'NONE',  ( -5.000000000000000000, -80.49999999999998579, 0.000000000000000000 ) ) ;
#26986=CARTESIAN_POINT ( 'NONE',  ( 9.507661145905998978, -77.55757109829465890, -5.611464101879999333 ) ) ;
#26994=CARTESIAN_POINT ( 'NONE',  ( -8.592320330817999618, -78.17107902543699538, 4.510292750937000328 ) ) ;
#27010=DIRECTION ( 'NONE',  ( 0.7071067811865474617, 0.7071067811865474617, -7.319351672370483695E-10 ) ) ;
#27018=CARTESIAN_POINT ( 'NONE',  ( -11.00000000000000000, -79.19999999999998863, 0.000000000000000000 ) ) ;
#27029=CARTESIAN_POINT ( 'NONE',  ( 3.187402732789999860, -78.30477596781798866, 8.972783294553000388 ) ) ;
#27058=DIRECTION ( 'NONE',  ( 0.000000000000000000, 1.000000000000000000, 0.000000000000000000 ) ) ;
#27063=CARTESIAN_POINT ( 'NONE',  ( 0.004634250437275883386, -78.72518518586632297, -9.249911725680748376 ) ) ;
#27066=CARTESIAN_POINT ( 'NONE',  ( -10.71369944335148183, -78.57916666666665151, 2.879226727952040932 ) ) ;
#27073=CARTESIAN_POINT ( 'NONE',  ( 10.03798773386740351, -79.88458675554201704, 4.654823617294056248 ) ) ;
#27096=EDGE_CURVE ( 'NONE', #3055, #1033, #19436, .T. ) ;
#27100=CARTESIAN_POINT ( 'NONE',  ( 5.436864099232999514, -79.00131553099198811, -8.080855302300999909 ) ) ;
#27111=DIRECTION ( 'NONE',  ( -3.944178317128000824E-11, 1.000000000000000000, 1.496715873672999954E-09 ) ) ;
#27112=EDGE_LOOP ( 'NONE', ( #8454, #38890, #5556, #12893, #34311 ) ) ;
#27113=CARTESIAN_POINT ( 'NONE',  ( -4.464053075535999504, -77.40064930226400008, 10.28489246429000126 ) ) ;
#27118=CARTESIAN_POINT ( 'NONE',  ( 6.728605944993000243, -79.51562678850498855, -7.080011783993000130 ) ) ;
#27132=CARTESIAN_POINT ( 'NONE',  ( -5.351292223237999579, -77.67148113580876156, 8.095330809056001442 ) ) ;
#27133=CARTESIAN_POINT ( 'NONE',  ( 8.528027178079026882, -79.88239481433151923, 3.637236233294601995 ) ) ;
#27135=ORIENTED_EDGE ( 'NONE', *, *, #3920, .F. ) ;
#27157=CARTESIAN_POINT ( 'NONE',  ( -8.968424590936999508, -77.11923613374659681, 2.773906523901999766 ) ) ;
#27165=EDGE_CURVE ( 'NONE', #49174, #27720, #7638, .T. ) ;
#27167=CARTESIAN_POINT ( 'NONE',  ( 7.318097147681000614, -79.61323130376099755, -8.179820946710000484 ) ) ;
#27175=CARTESIAN_POINT ( 'NONE',  ( -8.796335266379978535, -77.65208333333332291, -6.760013919724068288 ) ) ;
#27178=CARTESIAN_POINT ( 'NONE',  ( -6.511242784100999437, -78.66764840355199340, 9.060646613982999753 ) ) ;
#27179=B_SPLINE_CURVE_WITH_KNOTS ( 'NONE', 3,
 ( #2476, #25185, #56493, #29316, #51788, #24902, #52638, #55918, #52358, #6896, #34031, #16048, #38476, #34321, #7185, #56206, #11909, #12194 ),
 .UNSPECIFIED., .F., .F.,
 ( 4, 2, 2, 2, 2, 2, 2, 2, 4 ),
 ( 0.000000000000000000, 0.1250000000000000833, 0.2500000000000001110, 0.3750000000000001110, 0.5000000000000001110, 0.6250000000000002220, 0.7500000000000001110, 0.8750000000000001110, 1.000000000000000000 ),
 .UNSPECIFIED. ) ;
#27197=EDGE_CURVE ( 'NONE', #30305, #26900, #53676, .T. ) ;
#27200=CARTESIAN_POINT ( 'NONE',  ( -4.418675353760038504, -78.18548855279971121, -8.128508495965080627 ) ) ;
#27204=CARTESIAN_POINT ( 'NONE',  ( 0.000000000000000000, -74.64999999999999147, 0.000000000000000000 ) ) ;
#27206=CARTESIAN_POINT ( 'NONE',  ( 1.445980050911830794, -77.46252241678527639, 9.136273426141869436 ) ) ;
#27207=CARTESIAN_POINT ( 'NONE',  ( -7.062685404271999978, -77.86038984814099706, 8.485436034813998774 ) ) ;
#27209=CARTESIAN_POINT ( 'NONE',  ( -8.771427373352999268, -77.92563036551399591, -4.151237309591000013 ) ) ;
#27215=CARTESIAN_POINT ( 'NONE',  ( -9.781527233834999890, -78.96614208009899016, -4.899953194656999855 ) ) ;
#27220=B_SPLINE_CURVE_WITH_KNOTS ( 'NONE', 3,
 ( #22301, #49776, #40317, #1938, #55647, #15495, #54772, #50357, #50940, #781, #24054, #33485, #19930, #36753, #33187, #37044, #23761, #24357 ),
 .UNSPECIFIED., .F., .F.,
 ( 4, 2, 2, 2, 2, 2, 2, 2, 4 ),
 ( 0.000000000000000000, 0.1250000000000000000, 0.2500000000000000000, 0.3750000000000000000, 0.5000000000000000000, 0.6250000000000000000, 0.7500000000000000000, 0.8750000000000000000, 1.000000000000000000 ),
 .UNSPECIFIED. ) ;
#27260=AXIS2_PLACEMENT_3D ( 'NONE', #3766, #22353, #58079 ) ;
#27265=CARTESIAN_POINT ( 'NONE',  ( -10.71369944335148006, -79.57916666666666572, 2.879226727952048037 ) ) ;
#27269=ORIENTED_EDGE ( 'NONE', *, *, #23023, .F. ) ;
#27276=CARTESIAN_POINT ( 'NONE',  ( 10.52776997023000050, -80.12876079193905809, 3.979665013433000720 ) ) ;
#27278=ADVANCED_FACE ( 'NONE', ( #854 ), #20394, .F. ) ;
#27281=CARTESIAN_POINT ( 'NONE',  ( 1.160587285869999707, -77.71661964162117897, 10.97894289003999901 ) ) ;
#27283=EDGE_LOOP ( 'NONE', ( #9004, #31616, #999, #5009, #8831 ) ) ;
#27288=CARTESIAN_POINT ( 'NONE',  ( 5.417083560473000325, -78.88167475366098813, -8.051455326762999576 ) ) ;
#27294=EDGE_CURVE ( 'NONE', #26886, #47367, #13807, .T. ) ;
#27297=B_SPLINE_CURVE_WITH_KNOTS ( 'NONE', 3,
 ( #16984, #58300, #9293, #36151, #8120, #49455, #35252, #21977, #22574, #35850, #40586, #39699, #9001, #26986, #44724, #8702, #17861, #53578, #27281, #26120, #17558, #39988, #26692, #4277, #13116, #54168, #53880, #30829, #22866, #44141, #3689, #21691 ),
 .UNSPECIFIED., .F., .F.,
 ( 4, 1, 1, 1, 1, 1, 1, 1, 1, 1, 1, 1, 1, 1, 1, 1, 1, 1, 1, 1, 1, 1, 1, 1, 1, 1, 1, 1, 1, 4 ),
 ( 0.000000000000000000, 0.008721705557737447975, 0.04492002831815160996, 0.08111835107876277928, 0.1173166738391771546, 0.1535149965995915300, 0.1897133193600056833, 0.2259116421206168734, 0.2621099648810312210, 0.2983082876414456241, 0.3345066104018599717, 0.3707049331624711619, 0.4069032559228853430, 0.4431015786832996906, 0.4792999014439106586, 0.5154982242043252283, 0.5516965469647395759, 0.5878948697251540345, 0.6240931924857650026, 0.6602915152461791282, 0.6964898380065934758, 0.7326881607672046659, 0.7688864835276190135, 0.8050848062880334721, 0.8412831290484478197, 0.8774814518090590099, 0.9136797745694731354, 0.9498780973298874830, 0.9860764200904986732, 1.000000000000000000 ),
 .UNSPECIFIED. ) ;
#27306=CARTESIAN_POINT ( 'NONE',  ( 4.100000000000000533, -77.49999999999998579, 0.000000000000000000 ) ) ;
#27308=DIRECTION ( 'NONE',  ( -1.000000000000000000, 0.000000000000000000, 0.000000000000000000 ) ) ;
#27311=CARTESIAN_POINT ( 'NONE',  ( 9.535425472282794246, -77.20000000000000284, -5.121398017412860604 ) ) ;
#27312=ORIENTED_EDGE ( 'NONE', *, *, #10114, .T. ) ;
#27314=CARTESIAN_POINT ( 'NONE',  ( 10.32296845096999860, -78.33546437446798905, -4.912869655601999952 ) ) ;
#27315=CARTESIAN_POINT ( 'NONE',  ( -8.796335266379976758, -79.25208333333334565, -6.760013919724066511 ) ) ;
#27327=CARTESIAN_POINT ( 'NONE',  ( -5.574784109570000368, -78.53216660084999035, -7.719595738358999704 ) ) ;
#27336=ORIENTED_EDGE ( 'NONE', *, *, #34851, .T. ) ;
#27337=CARTESIAN_POINT ( 'NONE',  ( -4.385047663734000345, -79.77863228676199014, 10.02292886995000032 ) ) ;
#27349=CARTESIAN_POINT ( 'NONE',  ( 7.000000000000000000, -81.99999999999998579, 0.000000000000000000 ) ) ;
#27352=CARTESIAN_POINT ( 'NONE',  ( 0.000000000000000000, -77.49999999999998579, 0.000000000000000000 ) ) ;
#27353=ORIENTED_EDGE ( 'NONE', *, *, #37116, .F. ) ;
#27362=CARTESIAN_POINT ( 'NONE',  ( 6.543270582036108785, -78.78770373343947142, -6.538043958785086041 ) ) ;
#27369=LINE ( 'NONE', #45700, #57927 ) ;
#27399=CARTESIAN_POINT ( 'NONE',  ( -2.898344733286999819, -79.37214830381199704, -9.457017945469999631 ) ) ;
#27402=ORIENTED_EDGE ( 'NONE', *, *, #568, .T. ) ;
#27411=CARTESIAN_POINT ( 'NONE',  ( -2.815325398627000375, -78.03378302612298967, -10.73870018959999939 ) ) ;
#27414=VERTEX_POINT ( 'NONE', #31210 ) ;
#27417=CARTESIAN_POINT ( 'NONE',  ( -4.373213035511999358, -79.47851173940198066, -8.733596771889999388 ) ) ;
#27420=DIRECTION ( 'NONE',  ( -0.7071067811865474617, -0.7071067811865474617, 1.721800171537113669E-09 ) ) ;
#27425=AXIS2_PLACEMENT_3D ( 'NONE', #10240, #50403, #51572 ) ;
#27429=CARTESIAN_POINT ( 'NONE',  ( 7.256139241522999939, -77.55778581929276072, 6.443535727668999513 ) ) ;
#27430=CARTESIAN_POINT ( 'NONE',  ( 8.982775494571313857, -79.86926930857234197, 2.207202376408675892 ) ) ;
#27434=CARTESIAN_POINT ( 'NONE',  ( 2.859599080648278946, -77.25018204720734616, -8.796768031835178192 ) ) ;
#27444=VERTEX_POINT ( 'NONE', #18550 ) ;
#27452=CARTESIAN_POINT ( 'NONE',  ( -7.648940337505000464, -77.25890875220699172, -5.852081988951999492 ) ) ;
#27460=CIRCLE ( 'NONE', #2049, 1.000000000000000000 ) ;
#27461=CARTESIAN_POINT ( 'NONE',  ( -10.44304457033000055, -78.46556299312698002, 3.377400876517000050 ) ) ;
#27465=CARTESIAN_POINT ( 'NONE',  ( 9.499157866768639380, -79.10080562451891240, 0.1004279358040388037 ) ) ;
#27482=COLOUR_RGB ( '', 0.08235294, 0.09019608, 0.10196078) ;
#27496=ORIENTED_EDGE ( 'NONE', *, *, #32747, .T. ) ;
#27499=CARTESIAN_POINT ( 'NONE',  ( 3.727203065783209368, -77.44229855731178702, 8.514839819890244854 ) ) ;
#27500=CARTESIAN_POINT ( 'NONE',  ( 8.680753609988000719, -77.67284808780799210, 6.821192461343000168 ) ) ;
#27503=CARTESIAN_POINT ( 'NONE',  ( 9.367484565636001292, -79.11943118893098870, -2.533990228858999938 ) ) ;
#27507=CARTESIAN_POINT ( 'NONE',  ( -7.054457466615000172, -80.56154281250199745, -8.769379688592000122 ) ) ;
#27508=CARTESIAN_POINT ( 'NONE',  ( 8.999546809828999017, -78.13273556822998955, -5.951127176402999375 ) ) ;
#27522=CARTESIAN_POINT ( 'NONE',  ( 7.993200843029001135, -77.78490534060698280, -4.971914600080000746 ) ) ;
#27528=CYLINDRICAL_SURFACE ( 'NONE', #41973, 11.00000000000000000 ) ;
#27532=DIRECTION ( 'NONE',  ( 0.7071067811865969777, -0.7071067811864980568, -1.305609853748994042E-09 ) ) ;
#27540=EDGE_CURVE ( 'NONE', #25253, #26404, #27917, .T. ) ;
#27549=CARTESIAN_POINT ( 'NONE',  ( -10.13785388426000011, -78.38129286498505621, -4.205702700205000255 ) ) ;
#27560=VERTEX_POINT ( 'NONE', #7513 ) ;
#27579=FACE_OUTER_BOUND ( 'NONE', #40291, .T. ) ;
#27580=CARTESIAN_POINT ( 'NONE',  ( 0.000000000000000000, -76.19999999999998863, 0.000000000000000000 ) ) ;
#27588=CONICAL_SURFACE ( 'NONE', #46468, 9.649999999948999374, 0.7853981633972997312 ) ;
#27593=EDGE_CURVE ( 'NONE', #27414, #30828, #53371, .T. ) ;
#27598=ORIENTED_EDGE ( 'NONE', *, *, #16619, .T. ) ;
#27601=VECTOR ( 'NONE', #40651, 1000.000000000000000 ) ;
#27604=CARTESIAN_POINT ( 'NONE',  ( -5.192407727267999817, -79.90950158836399453, -8.254012402074000221 ) ) ;
#27613=CARTESIAN_POINT ( 'NONE',  ( 4.837141563511999642, -77.90371847557099727, -10.06315987337999829 ) ) ;
#27616=CARTESIAN_POINT ( 'NONE',  ( -9.108272167377998940, -77.48048492307799506, -2.776672910959999907 ) ) ;
#27626=CARTESIAN_POINT ( 'NONE',  ( -0.6493855936264999462, -79.75053993242899253, 10.92090362500000111 ) ) ;
#27638=B_SPLINE_SURFACE_WITH_KNOTS ( 'NONE', 3, 3, ( 
 ( #26335, #3620, #38768, #44351, #52362, #7480, #3905, #16919, #34615, #49080, #30758, #17487, #43792, #57069, #21907, #39916, #48232, #34898, #29891, #47948, #43497, #3058, #53214, #39631, #21053, #57932, #12761, #16629, #48791, #7767, #35474, #52928, #52643, #53503, #26616 ),
 ( #12478, #12198, #30479, #57638, #48506, #8051, #13045, #31043, #8630, #44651, #30182, #25770, #3341, #44071, #46131, #31926, #10101, #23082, #32503, #27500, #5371, #50548, #17788, #54961, #8927, #40513, #49971, #54394, #13931, #22502, #45541, #397, #18374, #54677, #13340 ),
 ( #9514, #22203, #5086, #14512, #23379, #58225, #14219, #108, #45246, #45836, #688, #31336, #41389, #32216, #9807, #41096, #18670, #36659, #36368, #50258, #27790, #26916, #9222, #27207, #40214, #972, #54098, #18955, #36948, #35777, #28081, #4503, #18083, #53805, #49380 ),
 ( #36077, #44947, #13638, #31634, #49676, #4794, #22794, #40803, #10689, #33093, #42270, #23664, #51135, #20125, #46719, #15396, #55845, #37825, #15684, #47005, #37527, #33680, #52003, #24544, #6532, #38403, #51718, #20409, #28373, #1836, #19245, #46418, #11268, #2125, #29248 ) ),
 .UNSPECIFIED., .F., .F., .F.,
 ( 4, 4 ),
 ( 4, 1, 1, 1, 1, 1, 1, 1, 1, 1, 1, 1, 1, 1, 1, 1, 1, 1, 1, 1, 1, 1, 1, 1, 1, 1, 1, 1, 1, 1, 1, 1, 4 ),
 ( -0.4045438850611000059, 1.404543885061000141 ),
 ( 0.4225136409995000064, 0.4409139416538999656, 0.4593142423082999803, 0.4777145429628000262, 0.4961148436172000409, 0.5145151442715999446, 0.5329154449260999904, 0.5513157455805000051, 0.5697160462349000198, 0.5881163468892999235, 0.6065166475437999694, 0.6249169481981999841, 0.6433172488525999988, 0.6617175495070000135, 0.6801178501615000593, 0.6985181508158999630, 0.7169184514702999778, 0.7353187521247999126, 0.7537190527792000383, 0.7721193534336000530, 0.7905196540880000677, 0.8089199547425000025, 0.8273202553968999062, 0.8457205560512999210, 0.8641208567057999668, 0.8825211573601999815, 0.9009214580145999962, 0.9193217586690000109, 0.9377220593235000567, 0.9561223599778999604, 0.9745226606322999752, 0.9929229612868000210, 1.011323261940999974 ),
 .UNSPECIFIED. ) ;
#27644=FACE_OUTER_BOUND ( 'NONE', #12461, .T. ) ;
#27652=CARTESIAN_POINT ( 'NONE',  ( -1.785035796832132426, -78.70961624886150787, -9.076082582026554491 ) ) ;
#27654=CARTESIAN_POINT ( 'NONE',  ( 0.000000000000000000, -80.99999999999998579, 7.000000000000000000 ) ) ;
#27655=CARTESIAN_POINT ( 'NONE',  ( -9.090730535106020582, -80.14771101264726383, -6.193863875913084627 ) ) ;
#27663=CARTESIAN_POINT ( 'NONE',  ( 2.194848540722183827, -79.99999999999997158, 9.090985499525780611 ) ) ;
#27670=CARTESIAN_POINT ( 'NONE',  ( 7.036824827271694005, -79.54050048329402500, -6.487746313484107574 ) ) ;
#27690=ORIENTED_EDGE ( 'NONE', *, *, #42111, .F. ) ;
#27699=EDGE_LOOP ( 'NONE', ( #56022, #31980, #16942, #18286 ) ) ;
#27700=CARTESIAN_POINT ( 'NONE',  ( 10.71380177098999908, -78.18052186078398336, 0.1798162837734999797 ) ) ;
#27702=ORIENTED_EDGE ( 'NONE', *, *, #29166, .T. ) ;
#27705=CARTESIAN_POINT ( 'NONE',  ( 9.630577183392999174, -79.15378515682199634, 1.628483183780000010 ) ) ;
#27718=CARTESIAN_POINT ( 'NONE',  ( 8.993876985514928535, -79.86887379514664076, 2.161346897475597828 ) ) ;
#27720=VERTEX_POINT ( 'NONE', #22830 ) ;
#27730=CARTESIAN_POINT ( 'NONE',  ( 9.267785752250999209, -78.32436279057898787, -6.128505448192000493 ) ) ;
#27739=CARTESIAN_POINT ( 'NONE',  ( 7.685661446562000343, -76.94999999999998863, -5.583959896778000420 ) ) ;
#27741=CARTESIAN_POINT ( 'NONE',  ( -1.944889849486000077, -77.31575641046499925, -9.432423272878001086 ) ) ;
#27746=EDGE_CURVE ( 'NONE', #51020, #49432, #32833, .T. ) ;
#27752=CARTESIAN_POINT ( 'NONE',  ( 6.612939829087000732, -79.81399600109497783, 8.759739992124000452 ) ) ;
#27753=CARTESIAN_POINT ( 'NONE',  ( -6.760013919724072728, -79.17291666666666572, -8.796335266379973206 ) ) ;
#27767=CARTESIAN_POINT ( 'NONE',  ( -9.569149049473001156, -79.26527887665599792, 5.523520626929999899 ) ) ;
#27771=CARTESIAN_POINT ( 'NONE',  ( 9.249999999999998224, -79.76041666666667140, 1.210822168571084934 ) ) ;
#27772=CARTESIAN_POINT ( 'NONE',  ( -6.405151242761908392, -78.87468806584735148, 8.913016123664291968 ) ) ;
#27789=CARTESIAN_POINT ( 'NONE',  ( 8.894028069796958036, -77.37240033373954873, 2.560412268026674987 ) ) ;
#27790=CARTESIAN_POINT ( 'NONE',  ( 5.341789944771999643, -77.76496072214499122, 9.661750877468000098 ) ) ;
#27799=CARTESIAN_POINT ( 'NONE',  ( -6.999846649096999940, -79.35943504075699195, 8.407732347380999727 ) ) ;
#27812=CARTESIAN_POINT ( 'NONE',  ( -2.117690490098999678, -77.47224322018799114, 9.172054377053999730 ) ) ;
#27823=CARTESIAN_POINT ( 'NONE',  ( -0.5193979750644999172, -78.93077836576598827, -10.96331347381999954 ) ) ;
#27837=FACE_OUTER_BOUND ( 'NONE', #42694, .T. ) ;
#27857=CARTESIAN_POINT ( 'NONE',  ( 2.095844585997434173, -78.24334418708741623, -9.009563528218526685 ) ) ;
#27865=CARTESIAN_POINT ( 'NONE',  ( -0.5548610165507998904, -77.89029600155998878, -9.688283574444998436 ) ) ;
#27884=CARTESIAN_POINT ( 'NONE',  ( 5.066607476199531668, -77.20000000000000284, -9.683877171469156053 ) ) ;
#27887=CARTESIAN_POINT ( 'NONE',  ( -7.515954563004000555, -78.18872553980699536, -8.614663944174999699 ) ) ;
#27891=CARTESIAN_POINT ( 'NONE',  ( -9.738223894236998746, -79.32504842320498994, 0.5068368411314999600 ) ) ;
#27897=CARTESIAN_POINT ( 'NONE',  ( 2.991086974322999747, -77.38964371959498578, -10.75725820134999999 ) ) ;
#27901=CARTESIAN_POINT ( 'NONE',  ( 1.442464609972999856, -77.65805598037698587, -9.302176701096998457 ) ) ;
#27909=VERTEX_POINT ( 'NONE', #14474 ) ;
#27913=CARTESIAN_POINT ( 'NONE',  ( -6.000000002940000243, -81.20000000293998710, 1.734976710454000070E-08 ) ) ;
#27917=CIRCLE ( 'NONE', #18504, 2.799999999999999822 ) ;
#27930=CARTESIAN_POINT ( 'NONE',  ( 4.187011524236304183, -78.51040584207294160, -8.754585214959869077 ) ) ;
#27937=EDGE_CURVE ( 'NONE', #47434, #23068, #40151, .T. ) ;
#27939=CARTESIAN_POINT ( 'NONE',  ( 7.695212739268346702, -78.80320820975849472, -5.132832367546954266 ) ) ;
#27943=CARTESIAN_POINT ( 'NONE',  ( -9.548515496062343288, -80.14175696964518636, -5.470885215208376451 ) ) ;
#27960=CARTESIAN_POINT ( 'NONE',  ( -9.014397739498770434, -77.40433534373462976, 5.897194292687825801 ) ) ;
#27963=CARTESIAN_POINT ( 'NONE',  ( 9.694840914897000062, -79.56117174695758365, -5.145296513660000848 ) ) ;
#27970=CARTESIAN_POINT ( 'NONE',  ( 8.587978511495325762, -78.31970074046702734, -3.439774535247742904 ) ) ;
#27974=CARTESIAN_POINT ( 'NONE',  ( 9.296715471869999803, -79.12203893003398036, -2.514846541900999988 ) ) ;
#27975=VECTOR ( 'NONE', #30030, 1000.000000000000000 ) ;
#27977=CARTESIAN_POINT ( 'NONE',  ( 9.249483092228999226, -78.85084128437098627, 0.09778817195952001218 ) ) ;
#27981=CARTESIAN_POINT ( 'NONE',  ( 8.200000000000001066, -80.99999999999998579, 0.000000000000000000 ) ) ;
#27989=CARTESIAN_POINT ( 'NONE',  ( -9.676120737181999942, -77.95091993224397697, 5.663874116999999764 ) ) ;
#27994=EDGE_CURVE ( 'NONE', #11369, #17717, #6494, .T. ) ;
#27995=CARTESIAN_POINT ( 'NONE',  ( -5.726462542197000793, -79.96560161327099081, -7.912542777261000637 ) ) ;
#28001=AXIS2_PLACEMENT_3D ( 'NONE', #48873, #192, #21417 ) ;
#28004=CIRCLE ( 'NONE', #56188, 10.50000000000000000 ) ;
#28007=CARTESIAN_POINT ( 'NONE',  ( 8.976219693957377288, -79.86950217340086056, 2.233771530619390155 ) ) ;
#28012=CARTESIAN_POINT ( 'NONE',  ( 5.491552160713999875, -77.07695060022997779, 7.961786551375001686 ) ) ;
#28022=CARTESIAN_POINT ( 'NONE',  ( 8.538884422081000736, -78.42736808979898910, 7.349585687664999867 ) ) ;
#28029=CARTESIAN_POINT ( 'NONE',  ( -3.845277600207000379, -76.92115273745038451, -8.724914968965999051 ) ) ;
#28031=B_SPLINE_CURVE_WITH_KNOTS ( 'NONE', 3,
 ( #50217, #40473, #933, #9765, #49341, #27753, #41351, #18915, #40765, #14473, #5615, #26882, #23626, #41638, #44906, #4462, #22461, #67 ),
 .UNSPECIFIED., .F., .F.,
 ( 4, 2, 2, 2, 2, 2, 2, 2, 4 ),
 ( 0.000000000000000000, 0.1250000000000000000, 0.2500000000000000000, 0.3750000000000000000, 0.5000000000000000000, 0.6250000000000000000, 0.7500000000000000000, 0.8750000000000000000, 1.000000000000000000 ),
 .UNSPECIFIED. ) ;
#28035=CARTESIAN_POINT ( 'NONE',  ( -3.877711979005999954, -77.79896150565798507, -8.815699619024998768 ) ) ;
#28042=CARTESIAN_POINT ( 'NONE',  ( 7.788493169598000421, -78.80267124511898658, 7.733265204867000087 ) ) ;
#28048=ORIENTED_EDGE ( 'NONE', *, *, #3561, .F. ) ;
#28062=CARTESIAN_POINT ( 'NONE',  ( 4.038850543673305538, -79.60508927849706140, -10.20566044646936099 ) ) ;
#28065=EDGE_LOOP ( 'NONE', ( #35673, #13811, #22927 ) ) ;
#28080=CARTESIAN_POINT ( 'NONE',  ( 9.220724224615148401, -77.35639230030703573, 0.7348276087542371382 ) ) ;
#28081=CARTESIAN_POINT ( 'NONE',  ( 3.792698199283999649, -78.08305780879798874, -10.36819406884000117 ) ) ;
#28083=CARTESIAN_POINT ( 'NONE',  ( -1.959694873104000257, -77.49927292857998395, -9.504225410855001499 ) ) ;
#28089=CARTESIAN_POINT ( 'NONE',  ( -10.40934573790000073, -78.40429499344598696, 3.366502286031999969 ) ) ;
#28103=CARTESIAN_POINT ( 'NONE',  ( 8.981578277711999903, -78.35338192318698702, 2.818234580162000125 ) ) ;
#28109=FACE_OUTER_BOUND ( 'NONE', #11340, .T. ) ;
#28112=CARTESIAN_POINT ( 'NONE',  ( 4.634563706678000550, -78.64985482243899639, 9.949112313689999709 ) ) ;
#28142=DIRECTION ( 'NONE',  ( -1.000000000000000000, 0.000000000000000000, 0.000000000000000000 ) ) ;
#28144=B_SPLINE_CURVE_WITH_KNOTS ( 'NONE', 3,
 ( #8093, #12518, #17528, #48831 ),
 .UNSPECIFIED., .F., .F.,
 ( 4, 4 ),
 ( 0.000000000000000000, 0.9996434014792530132 ),
 .UNSPECIFIED. ) ;
#28147=CARTESIAN_POINT ( 'NONE',  ( 6.718422235614084137, -78.28969101729559554, -6.358450322077904282 ) ) ;
#28152=CARTESIAN_POINT ( 'NONE',  ( -8.635538383447757482, -77.57078966990042090, 3.323345330289224631 ) ) ;
#28157=CARTESIAN_POINT ( 'NONE',  ( -5.681372509047000641, -78.34507726762299740, -7.867192369580999767 ) ) ;
#28176=ORIENTED_EDGE ( 'NONE', *, *, #2361, .T. ) ;
#28180=CARTESIAN_POINT ( 'NONE',  ( 3.902330291231000281, -79.98742867705199444, -8.777487365357000471 ) ) ;
#28183=CARTESIAN_POINT ( 'NONE',  ( 7.000000000000000000, -81.10000000285099020, 0.000000000000000000 ) ) ;
#28185=CARTESIAN_POINT ( 'NONE',  ( 6.578861079155999825, -77.41820342825998580, -9.021296591805000986 ) ) ;
#28188=CARTESIAN_POINT ( 'NONE',  ( -9.395661821092000210, -77.51593683473198837, 0.5765637145115000139 ) ) ;
#28207=VECTOR ( 'NONE', #17866, 1000.000000000000114 ) ;
#28211=VERTEX_POINT ( 'NONE', #4086 ) ;
#28212=DIRECTION ( 'NONE',  ( 0.000000000000000000, 1.000000000000000000, 0.000000000000000000 ) ) ;
#28217=CARTESIAN_POINT ( 'NONE',  ( -0.1538830739163870864, -78.22616755078296080, 9.703099906196978708 ) ) ;
#28218=VECTOR ( 'NONE', #50363, 1000.000000000000000 ) ;
#28228=ADVANCED_FACE ( 'NONE', ( #32114 ), #23557, .T. ) ;
#28229=CARTESIAN_POINT ( 'NONE',  ( 6.615973074419398969, -78.78858769152571995, -6.464602604579136269 ) ) ;
#28232=CARTESIAN_POINT ( 'NONE',  ( -10.50000000000000000, -76.19999999999998863, 0.000000000000000000 ) ) ;
#28248=CARTESIAN_POINT ( 'NONE',  ( 8.206048927592433984, -77.25648637437664945, 6.978187335436623506 ) ) ;
#28249=CARTESIAN_POINT ( 'NONE',  ( -11.00000000000000000, -78.09999999999999432, 2.733298954964999989E-14 ) ) ;
#28250=EDGE_CURVE ( 'NONE', #43973, #32937, #26062, .T. ) ;
#28252=CARTESIAN_POINT ( 'NONE',  ( 4.038786804788999873, -79.50498703829204317, -10.20549938644000321 ) ) ;
#28257=CARTESIAN_POINT ( 'NONE',  ( 9.047822906991040526, -78.33349585849774144, -1.923928064677009608 ) ) ;
#28261=CARTESIAN_POINT ( 'NONE',  ( -3.921497456393000292, -77.92121002409098196, -8.915242756422999904 ) ) ;
#28269=AXIS2_PLACEMENT_3D ( 'NONE', #45301, #3956, #58281 ) ;
#28275=CARTESIAN_POINT ( 'NONE',  ( -5.572401197671056572, -77.57410848619153398, -7.480459026222967545 ) ) ;
#28279=CARTESIAN_POINT ( 'NONE',  ( 3.720647276146999971, -77.77699006546498595, 10.45956222008999781 ) ) ;
#28285=CARTESIAN_POINT ( 'NONE',  ( 5.496668217546000434, -80.18287243149549681, -8.073860231047000013 ) ) ;
#28290=ORIENTED_EDGE ( 'NONE', *, *, #28425, .F. ) ;
#28295=CARTESIAN_POINT ( 'NONE',  ( -9.318755185595000157, -77.17535770753909219, -0.9064345995222999885 ) ) ;
#28318=CARTESIAN_POINT ( 'NONE',  ( -8.527407416480999203, -78.16847128433398950, 4.476218573567000369 ) ) ;
#28331=CARTESIAN_POINT ( 'NONE',  ( -1.297526016723000053, -78.60602476478999279, -10.89864408161000142 ) ) ;
#28333=CARTESIAN_POINT ( 'NONE',  ( 4.287008109733999817, -79.80461169611500338, -8.668125945862000137 ) ) ;
#28349=CIRCLE ( 'NONE', #51937, 4.299999999999999822 ) ;
#28353=CARTESIAN_POINT ( 'NONE',  ( -8.058765910997506055, -78.50948745952305785, -7.451450251813944270 ) ) ;
#28372=CARTESIAN_POINT ( 'NONE',  ( 8.239502079663772349, -77.38765822479125234, 4.203768253517201181 ) ) ;
#28373=CARTESIAN_POINT ( 'NONE',  ( -4.789974786805000662, -78.07974131713798727, -9.946872946892002076 ) ) ;
#28377=CARTESIAN_POINT ( 'NONE',  ( -10.99980394231345926, -80.10023817985064909, 1.711188753626703361E-06 ) ) ;
#28381=CARTESIAN_POINT ( 'NONE',  ( 4.619608356761999879, -78.76949559976999637, 9.917007359391000421 ) ) ;
#28392=CIRCLE ( 'NONE', #54796, 1.199999999999999956 ) ;
#28396=CARTESIAN_POINT ( 'NONE',  ( 7.653824198668000456, -78.77973936012098477, -5.479973919995999587 ) ) ;
#28406=CARTESIAN_POINT ( 'NONE',  ( 9.981840466370998755, -78.59367011377399592, 4.563647388395000171 ) ) ;
#28422=ORIENTED_EDGE ( 'NONE', *, *, #44653, .T. ) ;
#28425=EDGE_CURVE ( 'NONE', #6475, #1066, #41601, .T. ) ;
#28426=ORIENTED_EDGE ( 'NONE', *, *, #11328, .T. ) ;
#28428=FILL_AREA_STYLE ('',( #10442 ) ) ;
#28444=CARTESIAN_POINT ( 'NONE',  ( 3.546526562939293914, -78.25635398785173891, -8.543071106479906973 ) ) ;
#28447=ORIENTED_EDGE ( 'NONE', *, *, #31708, .T. ) ;
#28448=CARTESIAN_POINT ( 'NONE',  ( -7.603718805262172253, -77.55178371867702936, 5.267967937869231676 ) ) ;
#28453=CARTESIAN_POINT ( 'NONE',  ( 1.882180247600000245, -78.62931555891299240, 9.519879562373999349 ) ) ;
#28470=CARTESIAN_POINT ( 'NONE',  ( 8.097270260564613409, -77.19999999999998863, -7.230186543639936403 ) ) ;
#28476=FACE_OUTER_BOUND ( 'NONE', #15889, .T. ) ;
#28481=ADVANCED_FACE ( 'NONE', ( #2337 ), #56637, .F. ) ;
#28483=CARTESIAN_POINT ( 'NONE',  ( 6.642950389325999794, -77.35432768747699583, -9.109179383135000307 ) ) ;
#28484=EDGE_CURVE ( 'NONE', #30832, #38602, #12872, .T. ) ;
#28492=FACE_BOUND ( 'NONE', #30755, .T. ) ;
#28496=ORIENTED_EDGE ( 'NONE', *, *, #2208, .T. ) ;
#28511=VERTEX_POINT ( 'NONE', #38327 ) ;
#28515=CARTESIAN_POINT ( 'NONE',  ( -9.248792011962317261, -79.11076594009642804, -1.210867610392123428 ) ) ;
#28516=CARTESIAN_POINT ( 'NONE',  ( 9.131180374627371421, -77.57241948081694716, -3.285631257141331307 ) ) ;
#28521=CARTESIAN_POINT ( 'NONE',  ( -1.959694873104000257, -77.35881901538978411, -9.504225410855001499 ) ) ;
#28524=AXIS2_PLACEMENT_3D ( 'NONE', #3564, #55932, #55633 ) ;
#28526=CARTESIAN_POINT ( 'NONE',  ( -5.129512087222791727, -78.67834954393102009, -7.697348747938988822 ) ) ;
#28530=CARTESIAN_POINT ( 'NONE',  ( -5.704086182078374812, -80.18177924709463866, -9.405421966457751637 ) ) ;
#28534=AXIS2_PLACEMENT_3D ( 'NONE', #49632, #19205, #41346 ) ;
#28541=LINE ( 'NONE', #15266, #45145 ) ;
#28542=CARTESIAN_POINT ( 'NONE',  ( 1.210555553064095236, -79.73586375669722770, -9.250525361423333592 ) ) ;
#28550=CARTESIAN_POINT ( 'NONE',  ( 3.303001513109999898, -78.99932466030405465, -10.46681410870000128 ) ) ;
#28556=CARTESIAN_POINT ( 'NONE',  ( 8.164293671790550988, -78.31111438883360165, -4.349583488888277394 ) ) ;
#28560=CARTESIAN_POINT ( 'NONE',  ( 0.8552902072924000176, -78.52513851832499370, -9.592793577801000282 ) ) ;
#28576=CARTESIAN_POINT ( 'NONE',  ( 0.5884124957372001141, -77.49171607516498739, 11.41734628011000119 ) ) ;
#28580=CONICAL_SURFACE ( 'NONE', #34255, 9.400000000000000355, 0.7853981633972997312 ) ;
#28584=CARTESIAN_POINT ( 'NONE',  ( 9.534323188421000239, -79.07183379231298659, -1.008198710029000189 ) ) ;
#28605=EDGE_CURVE ( 'NONE', #55607, #31248, #52468, .T. ) ;
#28610=B_SPLINE_SURFACE_WITH_KNOTS ( 'NONE', 3, 3, ( 
 ( #45549, #27508, #13939, #19253, #36668, #31641, #980, #18677, #50267, #54401, #10108, #28089, #18092, #49978, #5094, #13646, #54969, #41103, #46139, #31935, #49684, #14808, #4802, #32802, #28381, #41686, #23090, #50850, #54104, #37247, #45253, #27215, #32224, #18382, #55260, #14519, #10396, #9230, #9521, #9814, #46427, #40814, #5958, #22803, #695, #27799, #23959, #404, #54685, #14226, #36375, #45844, #5378, #23386, #1265, #32511, #41397, #18965, #5663, #23672, #36957, #50556, #42857, #56144, #56433, #15693, #6245 ),
 ( #33100, #2417, #29831, #1845, #47600, #24552, #37537, #20419, #38414, #34262, #29544, #7126, #6543, #20134, #52293, #11853, #33688, #47882, #47305, #10698, #47013, #28675, #25126, #55552, #42566, #7413, #20704, #1549, #15984, #55852, #46728, #10989, #25418, #2132, #37832, #24262, #43150, #38121, #15405, #19540, #52012, #38702, #51726, #19837, #2709, #56724, #28970, #42278, #15102, #11278, #16281, #29256, #51143, #33397, #51436, #6831, #33974, #24843, #11566, #58158, #43431, #39280, #39570, #8861, #44291, #26276, #35407 ),
 ( #20989, #35120, #44010, #49016, #40146, #21844, #39851, #35712, #57867, #25700, #57002, #2990, #53153, #31269, #3846, #53741, #48731, #52866, #16855, #34549, #17420, #30119, #3281, #12700, #17136, #30695, #43729, #8274, #21564, #57572, #7986, #8563, #53438, #52581, #44582, #12980, #30978, #26553, #4139, #13276, #49311, #38994, #16565, #48169, #30410, #12132, #7700, #21273, #57291, #34836, #25984, #12421, #48445, #3560, #4733, #41, #26853, #5019, #910, #54621, #41326, #5589, #18017, #18894, #36009, #14448, #9742 ),
 ( #54035, #27730, #5311, #46067, #32443, #28022, #23602, #25403, #43718, #4127, #16844, #52570, #43419, #3838, #57280, #12121, #26546, #26266, #53428, #21263, #34537, #44279, #21836, #3271, #56992, #44572, #52854, #39841, #3550, #17413, #35396, #57856, #12971, #12690, #30106, #30969, #49006, #16269, #48157, #12408, #40138, #17124, #57562, #8554, #53143, #21553, #22127, #52283, #39558, #34826, #34248, #11839, #30684, #29820, #47870, #7400, #16554, #2978, #20977, #38981, #7688, #39269, #30398, #5010, #9152, #31557, #49303 ) ),
 .UNSPECIFIED., .F., .F., .F.,
 ( 4, 4 ),
 ( 4, 1, 1, 1, 1, 1, 1, 1, 1, 1, 1, 1, 1, 1, 1, 1, 1, 1, 1, 1, 1, 1, 1, 1, 1, 1, 1, 1, 1, 1, 1, 1, 1, 1, 1, 1, 1, 1, 1, 1, 1, 1, 1, 1, 1, 1, 1, 1, 1, 1, 1, 1, 1, 1, 1, 1, 1, 1, 1, 1, 1, 1, 1, 1, 4 ),
 ( -0.1387574078320000237, 1.138757407831999968 ),
 ( -0.02000000000000000042, -0.003749999999999999861, 0.01250000000000000069, 0.02875000000000000125, 0.04499999999999999833, 0.06124999999999999889, 0.07749999999999999944, 0.09375000000000000000, 0.1100000000000000006, 0.1262500000000000011, 0.1424999999999999878, 0.1587500000000000022, 0.1749999999999999889, 0.1912500000000000033, 0.2074999999999999900, 0.2237500000000000044, 0.2399999999999999911, 0.2562499999999999778, 0.2725000000000000200, 0.2887500000000000067, 0.3049999999999999933, 0.3212499999999999800, 0.3375000000000000222, 0.3537500000000000089, 0.3699999999999999956, 0.3862499999999999822, 0.4025000000000000244, 0.4187500000000000111, 0.4349999999999999978, 0.4512499999999999845, 0.4675000000000000266, 0.4837500000000000133, 0.5000000000000000000, 0.5162499999999999867, 0.5324999999999999734, 0.5487499999999999600, 0.5649999999999999467, 0.5812500000000000444, 0.5975000000000000311, 0.6137500000000000178, 0.6300000000000000044, 0.6462499999999999911, 0.6624999999999999778, 0.6787499999999999645, 0.6949999999999999512, 0.7112500000000000488, 0.7275000000000000355, 0.7437500000000000222, 0.7600000000000000089, 0.7762499999999999956, 0.7924999999999999822, 0.8087499999999999689, 0.8249999999999999556, 0.8412500000000000533, 0.8575000000000000400, 0.8737500000000000266, 0.8900000000000000133, 0.9062500000000000000, 0.9224999999999999867, 0.9387499999999999734, 0.9549999999999999600, 0.9712499999999999467, 0.9875000000000000444, 1.003749999999999920, 1.020000000000000018 ),
 .UNSPECIFIED. ) ;
#28613=CARTESIAN_POINT ( 'NONE',  ( -3.564835704203999978, -77.29834088185198482, 8.912408990994999058 ) ) ;
#28618=CARTESIAN_POINT ( 'NONE',  ( -9.212293474215000444, -77.23048492307799506, -2.808383990684999887 ) ) ;
#28620=CARTESIAN_POINT ( 'NONE',  ( 1.179538764136264906, -77.83344348886518560, -11.01565543437853734 ) ) ;
#28629=CARTESIAN_POINT ( 'NONE',  ( 0.1291013223160000223, -79.36451833177198978, 10.97485077029999978 ) ) ;
#28631=CARTESIAN_POINT ( 'NONE',  ( -0.09587540347749000380, -79.70338829707398531, -9.559386592703999597 ) ) ;
#28637=DIRECTION ( 'NONE',  ( -1.000000000000000000, 0.000000000000000000, 0.000000000000000000 ) ) ;
#28648=CARTESIAN_POINT ( 'NONE',  ( 7.219097972577888100, -79.26798102650505484, 8.267553648188542326 ) ) ;
#28652=ORIENTED_EDGE ( 'NONE', *, *, #23912, .F. ) ;
#28667=ORIENTED_EDGE ( 'NONE', *, *, #39224, .T. ) ;
#28668=CARTESIAN_POINT ( 'NONE',  ( 8.786704849164062026, -77.37533117377390113, 2.890659873118438306 ) ) ;
#28670=CARTESIAN_POINT ( 'NONE',  ( 7.405962610586999340, -77.58454441596599338, -6.270759699041999369 ) ) ;
#28675=CARTESIAN_POINT ( 'NONE',  ( 11.01715842067999951, -78.74909427755598301, 0.8367281403419999375 ) ) ;
#28677=CIRCLE ( 'NONE', #55072, 1.000000000000000000 ) ;
#28681=CARTESIAN_POINT ( 'NONE',  ( -10.19334857974716790, -77.19999999999998863, 4.001455984208257988 ) ) ;
#28690=CARTESIAN_POINT ( 'NONE',  ( -6.563619111649000359, -77.64278619496199951, -6.747599474233999750 ) ) ;
#28701=CARTESIAN_POINT ( 'NONE',  ( 9.632126701410999914, -79.09933249176198444, 5.261763182588000021 ) ) ;
#28718=CYLINDRICAL_SURFACE ( 'NONE', #7954, 4.100000000000000533 ) ;
#28736=VECTOR ( 'NONE', #22253, 1000.000000000000000 ) ;
#28737=CARTESIAN_POINT ( 'NONE',  ( 7.138081588315396075, -78.29522891051385614, -5.883131579888745577 ) ) ;
#28740=ORIENTED_EDGE ( 'NONE', *, *, #41511, .F. ) ;
#28741=CARTESIAN_POINT ( 'NONE',  ( -9.136481091602316695, -77.58766093786633178, 1.444190332375185903 ) ) ;
#28744=CARTESIAN_POINT ( 'NONE',  ( -2.183112477083999803, -77.66290536852798709, 9.455407409464999802 ) ) ;
#28747=DIRECTION ( 'NONE',  ( 0.000000000000000000, -1.000000000000000000, 0.000000000000000000 ) ) ;
#28748=ADVANCED_FACE ( 'NONE', ( #44433, #3418, #26412, #31422, #17872, #4285 ), #9012, .T. ) ;
#28771=CARTESIAN_POINT ( 'NONE',  ( -7.722420941044000564, -79.94415467088899163, -5.774298730193000218 ) ) ;
#28778=CARTESIAN_POINT ( 'NONE',  ( 10.96222314295999922, -77.91600195789497718, -1.826653240149999968 ) ) ;
#28782=CARTESIAN_POINT ( 'NONE',  ( -1.000000000000000000, -81.99999999999998579, 7.000000000000000000 ) ) ;
#28813=CARTESIAN_POINT ( 'NONE',  ( 7.890274420948999001, -78.95055344661277275, -5.649267206311999523 ) ) ;
#28818=CARTESIAN_POINT ( 'NONE',  ( -3.201792520036055301, -78.69701081001878151, -8.678388619861092224 ) ) ;
#28831=CARTESIAN_POINT ( 'NONE',  ( -9.250175331044397709, -79.60562764437898409, -0.6054718526037866644 ) ) ;
#28833=DIRECTION ( 'NONE',  ( 0.000000000000000000, 0.000000000000000000, -1.000000000000000000 ) ) ;
#28837=CARTESIAN_POINT ( 'NONE',  ( -10.74517267938467491, -77.94474881793972543, 0.7745379120455484490 ) ) ;
#28839=CARTESIAN_POINT ( 'NONE',  ( 10.87588596538000019, -79.58926410129005546, -1.476184626237000863 ) ) ;
#28848=CARTESIAN_POINT ( 'NONE',  ( -9.380647509327999956, -77.80751470757499533, 2.619761060131999830 ) ) ;
#28850=CARTESIAN_POINT ( 'NONE',  ( 6.731009509123192736, -80.24817708364265911, -8.757207002688298658 ) ) ;
#28861=CARTESIAN_POINT ( 'NONE',  ( 7.366954953549999630, -79.49001771131699456, -8.234431878459000487 ) ) ;
#28863=CARTESIAN_POINT ( 'NONE',  ( -11.41214431921999939, -80.16675248214399119, 1.797791303879000102 ) ) ;
#28867=CARTESIAN_POINT ( 'NONE',  ( 3.831544248136000252, -77.96861728781497902, 10.77131813041000008 ) ) ;
#28869=ORIENTED_EDGE ( 'NONE', *, *, #6959, .F. ) ;
#28874=CARTESIAN_POINT ( 'NONE',  ( 8.193575559979001000, -79.42596350198101618, 5.316613930189999948 ) ) ;
#28893=AXIS2_PLACEMENT_3D ( 'NONE', #7900, #29459, #30322 ) ;
#28894=CARTESIAN_POINT ( 'NONE',  ( -5.684557159767995138, -77.92708333333334281, 7.396918292183145560 ) ) ;
#28916=DIRECTION ( 'NONE',  ( 0.000000000000000000, -1.000000000000000000, 0.000000000000000000 ) ) ;
#28919=CARTESIAN_POINT ( 'NONE',  ( -9.250000000000000000, -78.09999999999999432, 0.000000000000000000 ) ) ;
#28923=DIRECTION ( 'NONE',  ( 0.000000000000000000, 1.000000000000000000, 0.000000000000000000 ) ) ;
#28924=CARTESIAN_POINT ( 'NONE',  ( -6.708975540371000079, -79.20704916398798900, -6.964516712451000124 ) ) ;
#28942=CARTESIAN_POINT ( 'NONE',  ( 0.1291033597530705512, -79.32416573517009795, 10.97502397199794544 ) ) ;
#28949=AXIS2_PLACEMENT_3D ( 'NONE', #40186, #21883, #49056 ) ;
#28958=ORIENTED_EDGE ( 'NONE', *, *, #52626, .F. ) ;
#28959=CARTESIAN_POINT ( 'NONE',  ( -10.69999999997999929, -81.80000000002199556, 2.760601855093000384E-10 ) ) ;
#28960=VERTEX_POINT ( 'NONE', #57644 ) ;
#28962=CARTESIAN_POINT ( 'NONE',  ( 8.506684281324854879, -77.38222109832315709, 3.641164479901510376 ) ) ;
#28970=CARTESIAN_POINT ( 'NONE',  ( -9.569149049473001156, -79.45140313587198477, 5.523520626929999899 ) ) ;
#28972=B_SPLINE_CURVE_WITH_KNOTS ( 'NONE', 3,
 ( #44167, #21717, #39722, #50355, #50649, #9902, #491, #41190, #1349, #6044, #24052, #50938, #27311, #36751, #18471, #19629, #36462, #32023, #31730, #28470, #32601, #54489, #54770, #9318, #42071, #27884, #1640, #41480, #4893, #779, #22890, #23759, #49774 ),
 .UNSPECIFIED., .F., .F.,
 ( 4, 2, 2, 1, 1, 1, 2, 2, 1, 1, 1, 2, 2, 1, 2, 2, 2, 2, 2, 4 ),
 ( 0.000000000000000000, 0.06250000000000030531, 0.1250000000000005829, 0.1875000000000008604, 0.2187500000000009992, 0.2343750000000010825, 0.2421875000000010825, 0.2500000000000010547, 0.3125000000000012212, 0.3437500000000012768, 0.3593750000000013323, 0.3671875000000013323, 0.3750000000000013878, 0.4375000000000009992, 0.4687500000000009437, 0.5000000000000008882, 0.6250000000000006661, 0.7500000000000004441, 0.8750000000000001110, 1.000000000000000000 ),
 .UNSPECIFIED. ) ;
#28977=CARTESIAN_POINT ( 'NONE',  ( -10.16547580793340622, -77.20000000000000284, 4.069192989858231968 ) ) ;
#28983=CIRCLE ( 'NONE', #6360, 2.600000000000000089 ) ;
#28987=CARTESIAN_POINT ( 'NONE',  ( 1.442464609972999856, -77.21642875802798756, -9.302176701096998457 ) ) ;
#28999=CARTESIAN_POINT ( 'NONE',  ( 6.718030245586000149, -78.98696307443100295, -8.679405866825000260 ) ) ;
#29001=CYLINDRICAL_SURFACE ( 'NONE', #45095, 9.250000000000000000 ) ;
#29010=CARTESIAN_POINT ( 'NONE',  ( -1.210822168571079605, -78.11458333333335702, -9.250000000000000000 ) ) ;
#29012=CARTESIAN_POINT ( 'NONE',  ( 0.9331110433225999756, -78.54758795410299399, 11.22756599386000076 ) ) ;
#29036=CARTESIAN_POINT ( 'NONE',  ( 3.540722753092142572, -78.25630082268401111, -8.545476915601279089 ) ) ;
#29040=CARTESIAN_POINT ( 'NONE',  ( -9.238076119067644143, -77.59563551126068148, 0.5262792932712636595 ) ) ;
#29043=CARTESIAN_POINT ( 'NONE',  ( -7.203390125892000562, -78.82828236281598322, -6.502451851937000704 ) ) ;
#29054=LINE ( 'NONE', #47093, #32504 ) ;
#29057=CARTESIAN_POINT ( 'NONE',  ( -8.081851865186232331, -79.55868232694022879, 4.658047483831220248 ) ) ;
#29062=VERTEX_POINT ( 'NONE', #12484 ) ;
#29066=CARTESIAN_POINT ( 'NONE',  ( -3.906545279024999928, -79.30125618921398711, 8.815735697348999977 ) ) ;
#29074=CARTESIAN_POINT ( 'NONE',  ( -11.04409640815999971, -77.31072091705098615, -0.5254229673086000529 ) ) ;
#29077=CARTESIAN_POINT ( 'NONE',  ( -7.608915353569000395, -77.97071810079599175, 5.542165790529000269 ) ) ;
#29099=EDGE_LOOP ( 'NONE', ( #57541, #3837 ) ) ;
#29103=ORIENTED_EDGE ( 'NONE', *, *, #45453, .F. ) ;
#29109=CARTESIAN_POINT ( 'NONE',  ( -0.5548610165507998904, -77.87044793971165291, -9.688283574444998436 ) ) ;
#29111=CARTESIAN_POINT ( 'NONE',  ( -7.781451050798130709, -79.90091309342098214, -5.818437412919247542 ) ) ;
#29114=CARTESIAN_POINT ( 'NONE',  ( -6.936452160827999869, -78.65757999610664797, -6.128159196645447615 ) ) ;
#29116=CARTESIAN_POINT ( 'NONE',  ( 2.166634614239063377E-07, -77.01246206852036380, -9.437473063691797392 ) ) ;
#29126=DIRECTION ( 'NONE',  ( -0.7071067811865470176, -0.7071067811865470176, -3.680441518142245308E-08 ) ) ;
#29131=CARTESIAN_POINT ( 'NONE',  ( 7.744117733784010582, -77.63885439857841675, -7.580542634272604552 ) ) ;
#29133=CARTESIAN_POINT ( 'NONE',  ( -9.813193589766999736, -78.88695524297345685, -4.915816122623000162 ) ) ;
#29135=ORIENTED_EDGE ( 'NONE', *, *, #57426, .T. ) ;
#29144=CARTESIAN_POINT ( 'NONE',  ( -0.1544424224854999972, -78.20544831538099118, 9.738369639964998825 ) ) ;
#29148=VERTEX_POINT ( 'NONE', #25697 ) ;
#29153=EDGE_CURVE ( 'NONE', #5025, #9279, #20843, .T. ) ;
#29158=CARTESIAN_POINT ( 'NONE',  ( -4.551883652666999680, -77.52840078382998001, 10.48724849044000074 ) ) ;
#29162=CIRCLE ( 'NONE', #36711, 9.750000000000000000 ) ;
#29165=CARTESIAN_POINT ( 'NONE',  ( 1.841371367509999857, -80.27025261668801193, -9.592189096167999196 ) ) ;
#29166=EDGE_CURVE ( 'NONE', #31439, #32566, #55358, .T. ) ;
#29174=LINE ( 'NONE', #34172, #27975 ) ;
#29175=DIRECTION ( 'NONE',  ( 1.000000000000000000, 0.000000000000000000, 0.000000000000000000 ) ) ;
#29176=LINE ( 'NONE', #42776, #37239 ) ;
#29177=CARTESIAN_POINT ( 'NONE',  ( 7.033509982383000292, -77.03085009973318620, 6.880083864244000758 ) ) ;
#29179=CARTESIAN_POINT ( 'NONE',  ( -1.439896632895311335, -79.71458333333333712, -11.00000000000000178 ) ) ;
#29183=CARTESIAN_POINT ( 'NONE',  ( 4.888750975951074551, -77.12187499993380868, -7.978256397349015927 ) ) ;
#29187=DIRECTION ( 'NONE',  ( 0.000000000000000000, 1.000000000000000000, 0.000000000000000000 ) ) ;
#29199=CARTESIAN_POINT ( 'NONE',  ( 9.725848778082999857, -78.51658531640698868, -0.5172632330995999839 ) ) ;
#29201=CARTESIAN_POINT ( 'NONE',  ( -0.1577822530794797395, -77.82391181108907574, -11.07750337872512780 ) ) ;
#29203=DIRECTION ( 'NONE',  ( -1.000000000000000000, 0.000000000000000000, 0.000000000000000000 ) ) ;
#29206=CARTESIAN_POINT ( 'NONE',  ( 2.421389049398865900, -77.95433015483983752, 9.009788787264410459 ) ) ;
#29209=CARTESIAN_POINT ( 'NONE',  ( -9.672666136464620479, -80.06087742290506526, 5.252905469540832151 ) ) ;
#29210=CARTESIAN_POINT ( 'NONE',  ( 9.385821630279000516, -78.84439215714098736, 1.815438171114999832 ) ) ;
#29211=CARTESIAN_POINT ( 'NONE',  ( 0.000000000000000000, -80.49999999999998579, 0.000000000000000000 ) ) ;
#29220=EDGE_CURVE ( 'NONE', #5962, #52316, #37453, .T. ) ;
#29221=CARTESIAN_POINT ( 'NONE',  ( 0.000000000000000000, -77.49999999999998579, 0.000000000000000000 ) ) ;
#29244=ORIENTED_EDGE ( 'NONE', *, *, #47114, .T. ) ;
#29247=CARTESIAN_POINT ( 'NONE',  ( 4.200728562467627825, -77.26253573339837999, -8.241112584695276411 ) ) ;
#29248=CARTESIAN_POINT ( 'NONE',  ( 10.74764839381999870, -78.23878986046499051, -0.2248421733643000131 ) ) ;
#29253=FACE_OUTER_BOUND ( 'NONE', #40801, .T. ) ;
#29256=CARTESIAN_POINT ( 'NONE',  ( -3.571993175857000491, -79.59186490753599230, -10.45556112308999985 ) ) ;
#29270=CARTESIAN_POINT ( 'NONE',  ( -2.523869816676000077, -78.24671468919598283, -9.181528052588999955 ) ) ;
#29282=CARTESIAN_POINT ( 'NONE',  ( -8.058638732054999920, -78.42923420478300045, -7.451332657186999775 ) ) ;
#29292=CARTESIAN_POINT ( 'NONE',  ( -7.103610810849999346, -79.24989681241999051, -8.744578195291998313 ) ) ;
#29315=CARTESIAN_POINT ( 'NONE',  ( -1.803312564769471660, -78.20945996376244125, -9.072471366556113637 ) ) ;
#29316=CARTESIAN_POINT ( 'NONE',  ( -8.090227444665263334, -79.45847354739515822, 4.644024077103019899 ) ) ;
#29317=ORIENTED_EDGE ( 'NONE', *, *, #28605, .F. ) ;
#29324=CIRCLE ( 'NONE', #50126, 5.500000000000000000 ) ;
#29325=CARTESIAN_POINT ( 'NONE',  ( 2.260091721765999928, -78.97385677587398334, -9.437303113984999214 ) ) ;
#29338=DIRECTION ( 'NONE',  ( 0.000000000000000000, 0.7071067811866525998, -0.7071067811864425456 ) ) ;
#29341=CARTESIAN_POINT ( 'NONE',  ( -10.65969359034999897, -80.46865055360498786, 3.376454609634999660 ) ) ;
#29345=EDGE_CURVE ( 'NONE', #10810, #47434, #35445, .T. ) ;
#29350=VECTOR ( 'NONE', #34950, 1000.000000000000000 ) ;
#29351=CARTESIAN_POINT ( 'NONE',  ( -9.175873485632997983, -79.97880775341398873, -2.587226946429999952 ) ) ;
#29353=CARTESIAN_POINT ( 'NONE',  ( -0.4846980698234193974, -79.22879212854250852, 9.704134706623241513 ) ) ;
#29356=CARTESIAN_POINT ( 'NONE',  ( 11.00000000000000000, -77.44999999999998863, 0.000000000000000000 ) ) ;
#29358=CARTESIAN_POINT ( 'NONE',  ( -7.206703837310000083, -77.80299228781500176, 8.241246436175000412 ) ) ;
#29364=CARTESIAN_POINT ( 'NONE',  ( 7.559982449049000408, -76.96625235366248319, -6.032732969207000195 ) ) ;
#29366=CARTESIAN_POINT ( 'NONE',  ( 11.00000000000000000, -77.34999999999999432, 0.000000000000000000 ) ) ;
#29374=VERTEX_POINT ( 'NONE', #2280 ) ;
#29378=VERTEX_POINT ( 'NONE', #11998 ) ;
#29398=CARTESIAN_POINT ( 'NONE',  ( 2.309309650359952393, -76.99409235924242978, -9.392413018435071592 ) ) ;
#29400=CARTESIAN_POINT ( 'NONE',  ( -4.876868007374968172, -78.68090168310180843, -7.860757581031139196 ) ) ;
#29407=VECTOR ( 'NONE', #8757, 1000.000000000000000 ) ;
#29420=CARTESIAN_POINT ( 'NONE',  ( -3.788397905917849862, -77.54708607277024157, -10.15569713685381537 ) ) ;
#29431=CARTESIAN_POINT ( 'NONE',  ( -9.596198845516999754, -77.89981427748799092, -0.8161970854479000392 ) ) ;
#29438=CARTESIAN_POINT ( 'NONE',  ( -7.998217534801063344, -77.54306880728415763, -4.799733181834938023 ) ) ;
#29442=CARTESIAN_POINT ( 'NONE',  ( -7.443442755000000410, -78.12484979902399118, -8.531552098207999535 ) ) ;
#29444=VERTEX_POINT ( 'NONE', #29116 ) ;
#29448=CARTESIAN_POINT ( 'NONE',  ( 1.739862777674999972, -79.37105597504650234, 9.611119481339999382 ) ) ;
#29459=DIRECTION ( 'NONE',  ( 0.000000000000000000, -1.000000000000000000, 0.000000000000000000 ) ) ;
#29462=CARTESIAN_POINT ( 'NONE',  ( 9.620021812515000548, -76.95241263186049707, -2.063756841170000023 ) ) ;
#29471=FACE_OUTER_BOUND ( 'NONE', #38504, .T. ) ;
#29478=CARTESIAN_POINT ( 'NONE',  ( 0.000000000000000000, -81.90000000002299885, 0.000000000000000000 ) ) ;
#29483=CARTESIAN_POINT ( 'NONE',  ( -4.832441116568999995, -78.68712829118099705, 8.456193503077001239 ) ) ;
#29487=DIRECTION ( 'NONE',  ( 0.000000000000000000, 0.000000000000000000, -1.000000000000000000 ) ) ;
#29497=CARTESIAN_POINT ( 'NONE',  ( -11.00000000000000000, -77.69999999999998863, 0.000000000000000000 ) ) ;
#29498=CARTESIAN_POINT ( 'NONE',  ( -1.288745046912000092, -80.02869764566298727, 9.583962847433999954 ) ) ;
#29500=CARTESIAN_POINT ( 'NONE',  ( 1.439896632895333539, -78.73541666666665151, -10.99999999999999822 ) ) ;
#29523=CARTESIAN_POINT ( 'NONE',  ( -4.814939325413682525, -78.76622030423393994, 8.425567463547647407 ) ) ;
#29527=CARTESIAN_POINT ( 'NONE',  ( 4.100000000000000533, -75.19999999999998863, 0.000000000000000000 ) ) ;
#29531=ORIENTED_EDGE ( 'NONE', *, *, #49961, .F. ) ;
#29533=ORIENTED_EDGE ( 'NONE', *, *, #23115, .F. ) ;
#29534=CARTESIAN_POINT ( 'NONE',  ( 5.439234600025764088, -77.27515920132572091, -7.481681149270881903 ) ) ;
#29544=CARTESIAN_POINT ( 'NONE',  ( -8.689005542484000699, -78.44007837989597931, 6.824886543446999632 ) ) ;
#29551=CARTESIAN_POINT ( 'NONE',  ( 2.457916154627046712, -77.19999999999998863, 10.51642625215182036 ) ) ;
#29559=CARTESIAN_POINT ( 'NONE',  ( 6.123453098898000491, -77.96247639790598782, 7.292029784470999587 ) ) ;
#29570=CARTESIAN_POINT ( 'NONE',  ( -6.920341278396000106, -79.44055896075899170, -8.518972542050999408 ) ) ;
#29578=CARTESIAN_POINT ( 'NONE',  ( 10.71369944335147117, -77.97083333333331723, 2.879226727952105769 ) ) ;
#29579=CARTESIAN_POINT ( 'NONE',  ( 7.511900341590999730, -79.36226622975098621, -8.396444939682998765 ) ) ;
#29602=CARTESIAN_POINT ( 'NONE',  ( -1.734462217213118773, -78.21007448308577636, -9.085917012415309912 ) ) ;
#29607=CARTESIAN_POINT ( 'NONE',  ( -7.440986743656934799, -77.54937432391301400, 5.495388714296327137 ) ) ;
#29611=CARTESIAN_POINT ( 'NONE',  ( 0.8618009059429999619, -78.46222785155198665, -9.665816497589000633 ) ) ;
#29627=CARTESIAN_POINT ( 'NONE',  ( 6.112256811392500211, -79.41782375574760522, 6.968603012018727227 ) ) ;
#29628=CARTESIAN_POINT ( 'NONE',  ( -8.481311802608001216, -79.93973307352598567, 6.721462691642999587 ) ) ;
#29637=CARTESIAN_POINT ( 'NONE',  ( -9.167409920518998945, -79.41814682224598698, -2.989462504633000339 ) ) ;
#29643=CARTESIAN_POINT ( 'NONE',  ( 7.906400319760000350, -78.06002966580298619, -7.572567058774000159 ) ) ;
#29650=CARTESIAN_POINT ( 'NONE',  ( -9.467475792354999697, -77.31375831598298021, 1.978357023055999919 ) ) ;
#29652=CARTESIAN_POINT ( 'NONE',  ( -8.796335266380006956, -77.54791666666667993, 6.760013919724027431 ) ) ;
#29670=ORIENTED_EDGE ( 'NONE', *, *, #32095, .F. ) ;
#29683=CARTESIAN_POINT ( 'NONE',  ( 9.670688080733903291, -77.09852982711514358, -0.1674119159864788653 ) ) ;
#29685=CARTESIAN_POINT ( 'NONE',  ( -3.304785372409708710, -78.69605523039359696, -8.639930098831065663 ) ) ;
#29707=CARTESIAN_POINT ( 'NONE',  ( 9.684822944874866835, -78.30969691107382857, -5.379607873393639217 ) ) ;
#29715=CARTESIAN_POINT ( 'NONE',  ( 1.251117773441000169, -77.75769513184299342, 9.549236319306000809 ) ) ;
#29719=ORIENTED_EDGE ( 'NONE', *, *, #26817, .T. ) ;
#29725=CARTESIAN_POINT ( 'NONE',  ( 5.312973029106999867, -78.20546044413198672, 9.563478878364000124 ) ) ;
#29727=CARTESIAN_POINT ( 'NONE',  ( -9.428734693618999074, -79.82940494353799465, 5.424968178012999687 ) ) ;
#29730=EDGE_LOOP ( 'NONE', ( #53941, #51632, #57053 ) ) ;
#29735=CARTESIAN_POINT ( 'NONE',  ( -8.396223008680999911, -80.17283464191400810, -4.990405176070999538 ) ) ;
#29764=CARTESIAN_POINT ( 'NONE',  ( 9.618404959434000645, -78.03338022121498341, 1.531659799953999812 ) ) ;
#29773=CARTESIAN_POINT ( 'NONE',  ( 9.081835416235971792, -79.47540137645063396, -2.898796417172264217 ) ) ;
#29774=CARTESIAN_POINT ( 'NONE',  ( -0.7301085713275398126, -79.99999999999998579, -9.448919309928943022 ) ) ;
#29777=CARTESIAN_POINT ( 'NONE',  ( 9.743790892929999004, -80.00705849419799165, -1.701210078859999975 ) ) ;
#29779=CARTESIAN_POINT ( 'NONE',  ( 7.396918292183175758, -79.19791666666665719, -5.684557159767951617 ) ) ;
#29788=ORIENTED_EDGE ( 'NONE', *, *, #38802, .F. ) ;
#29793=CARTESIAN_POINT ( 'NONE',  ( -9.254388464354001087, -79.90752053325199711, 5.469807505829999528 ) ) ;
#29795=CARTESIAN_POINT ( 'NONE',  ( -2.116314338179000387, -79.81716549451699905, -9.535298106756000536 ) ) ;
#29804=CARTESIAN_POINT ( 'NONE',  ( -1.565148314788150197, -78.73779647510495749, 9.577271978113845563 ) ) ;
#29806=ADVANCED_FACE ( 'NONE', ( #43055 ), #43921, .T. ) ;
#29811=CARTESIAN_POINT ( 'NONE',  ( -7.000000000000000000, -80.99999999999998579, 0.000000000000000000 ) ) ;
#29815=CARTESIAN_POINT ( 'NONE',  ( 3.539309974270077319, -79.94384682290294108, 8.546032899262883120 ) ) ;
#29820=CARTESIAN_POINT ( 'NONE',  ( 4.145744906942999464, -79.77580109776799588, -10.47576887544000002 ) ) ;
#29821=CARTESIAN_POINT ( 'NONE',  ( 9.153609394656651688, -77.33741943966701626, -1.470339571718344285 ) ) ;
#29831=CARTESIAN_POINT ( 'NONE',  ( 10.38514225167999960, -78.21533954523499688, -3.771779243421000238 ) ) ;
#29833=DIRECTION ( 'NONE',  ( 0.000000000000000000, 0.000000000000000000, -1.000000000000000000 ) ) ;
#29836=CARTESIAN_POINT ( 'NONE',  ( -8.985908341961819090, -77.20000000000000284, 6.204576319714215416 ) ) ;
#29844=CARTESIAN_POINT ( 'NONE',  ( -9.171168281578999881, -77.62139044835899426, 2.561259179188999813 ) ) ;
#29851=CARTESIAN_POINT ( 'NONE',  ( -4.658475568430852753, -78.91666666666665719, 8.082524092276868188 ) ) ;
#29855=CARTESIAN_POINT ( 'NONE',  ( 10.74341457190999982, -79.10345070876699936, -2.245675826504000216 ) ) ;
#29865=CARTESIAN_POINT ( 'NONE',  ( -2.879226727952121312, -78.09583333333330302, 10.71369944335146052 ) ) ;
#29867=CARTESIAN_POINT ( 'NONE',  ( 6.184832724006000149, -78.41481721455799914, -9.286519468188998871 ) ) ;
#29877=VERTEX_POINT ( 'NONE', #12611 ) ;
#29890=CARTESIAN_POINT ( 'NONE',  ( -2.988019896091281158, -77.50128957587054401, 8.754269285533984757 ) ) ;
#29891=CARTESIAN_POINT ( 'NONE',  ( 10.65102452230999930, -77.58073545347198774, 2.905137941168000282 ) ) ;
#29894=CARTESIAN_POINT ( 'NONE',  ( 7.256139241522999939, -77.63793680681199305, 6.443535727668999513 ) ) ;
#29898=CARTESIAN_POINT ( 'NONE',  ( 11.10498291493000167, -80.04654471278098526, -1.830582403018000015 ) ) ;
#29908=CARTESIAN_POINT ( 'NONE',  ( 9.249548791923931645, -78.36046089431209793, 1.210758159010477009 ) ) ;
#29912=CARTESIAN_POINT ( 'NONE',  ( 0.7294602504688000311, -80.36286705758899984, 11.15791328003000160 ) ) ;
#29923=CARTESIAN_POINT ( 'NONE',  ( 1.995261538442000049, -79.66278893684399520, -9.211143000868998953 ) ) ;
#29927=CARTESIAN_POINT ( 'NONE',  ( 0.000000000000000000, -76.29999999995945359, 0.000000000000000000 ) ) ;
#29928=CARTESIAN_POINT ( 'NONE',  ( -9.611650271896834852, -77.24166666666666003, -5.539808784079895965 ) ) ;
#29930=CARTESIAN_POINT ( 'NONE',  ( -10.77935564133999868, -77.82479567302799239, -2.460411616693999992 ) ) ;
#29935=CARTESIAN_POINT ( 'NONE',  ( -8.324924863653999196, -77.16704309767348491, 4.923709561474999497 ) ) ;
#29972=CARTESIAN_POINT ( 'NONE',  ( 7.764384370167843663, -77.15074856105154311, 5.767544481182754090 ) ) ;
#29974=CARTESIAN_POINT ( 'NONE',  ( -8.997583233551933901, -78.61904547633861284, -2.178759007882292931 ) ) ;
#29976=CARTESIAN_POINT ( 'NONE',  ( -10.89601512763299240, -80.11112176916604710, -1.508143038157861993 ) ) ;
#29991=CARTESIAN_POINT ( 'NONE',  ( 10.28103400416999946, -78.08800773578599319, 3.842432268884000024 ) ) ;
#30002=CARTESIAN_POINT ( 'NONE',  ( 4.996366032364999654, -78.78798106301098869, 8.105967104710000370 ) ) ;
#30011=CARTESIAN_POINT ( 'NONE',  ( -3.661365483191000081, -79.27296990877398741, 10.30932680317000028 ) ) ;
#30013=CARTESIAN_POINT ( 'NONE',  ( 11.06914806276000185, -80.10781271246199253, -1.824675266527999939 ) ) ;
#30022=CARTESIAN_POINT ( 'NONE',  ( 9.534323188421000239, -79.37184240488002729, -1.008198710029000189 ) ) ;
#30027=EDGE_CURVE ( 'NONE', #24330, #56968, #50711, .T. ) ;
#30030=DIRECTION ( 'NONE',  ( -1.776356839400000238E-14, 1.000000000000000000, -4.909721057536999944E-14 ) ) ;
#30037=LINE ( 'NONE', #51936, #1662 ) ;
#30039=EDGE_CURVE ( 'NONE', #36505, #15394, #28983, .T. ) ;
#30048=CARTESIAN_POINT ( 'NONE',  ( 8.929983232555001038, -77.17945105385759064, -3.213320707285999500 ) ) ;
#30053=CARTESIAN_POINT ( 'NONE',  ( -9.380647509327999956, -77.74914192992498840, 2.619761060131999830 ) ) ;
#30063=CARTESIAN_POINT ( 'NONE',  ( -3.879127410312085633, -79.34166267545728601, -8.706117637024775036 ) ) ;
#30067=CARTESIAN_POINT ( 'NONE',  ( -9.399803042841998746, -79.74562488639199387, 3.078846114291999836 ) ) ;
#30069=CARTESIAN_POINT ( 'NONE',  ( -9.009247259181922374, -79.02083333333334281, -2.421167930323344653 ) ) ;
#30079=DIRECTION ( 'NONE',  ( 0.000000000000000000, 1.000000000000000000, 0.000000000000000000 ) ) ;
#30081=CYLINDRICAL_SURFACE ( 'NONE', #10133, 5.000000000000000000 ) ;
#30083=CARTESIAN_POINT ( 'NONE',  ( -9.387315177295000979, -79.68727486148499395, 2.697965643110000311 ) ) ;
#30085=ORIENTED_EDGE ( 'NONE', *, *, #51838, .T. ) ;
#30102=CARTESIAN_POINT ( 'NONE',  ( 5.335925835648241744, -79.92656333706742089, 7.555489928919846498 ) ) ;
#30106=CARTESIAN_POINT ( 'NONE',  ( -0.5331530516160000177, -79.24204636544699554, -11.25365194899999999 ) ) ;
#30107=CARTESIAN_POINT ( 'NONE',  ( 6.587734798705522365, -77.28814994202326716, -6.493410667348151755 ) ) ;
#30117=CARTESIAN_POINT ( 'NONE',  ( 10.99999999999999645, -78.36041666666666572, 1.439896632895345974 ) ) ;
#30119=CARTESIAN_POINT ( 'NONE',  ( 11.12554012740000076, -78.81297001833898719, 0.8449594846185999319 ) ) ;
#30122=DIRECTION ( 'NONE',  ( 0.000000000000000000, -1.000000000000000000, 0.000000000000000000 ) ) ;
#30134=CARTESIAN_POINT ( 'NONE',  ( -8.420145992286000691, -77.04588578325369497, 3.744741888101000171 ) ) ;
#30140=CARTESIAN_POINT ( 'NONE',  ( 4.658475568430798575, -78.83333333333330017, 8.082524092276898386 ) ) ;
#30145=CARTESIAN_POINT ( 'NONE',  ( 8.212410987726999068, -78.12433652412899221, -6.936771999183999782 ) ) ;
#30147=CARTESIAN_POINT ( 'NONE',  ( 9.506651817130499893, -80.31979166666521053, 5.480266767440791220 ) ) ;
#30149=CARTESIAN_POINT ( 'NONE',  ( -9.967566199302938301, -79.66460044437665999, 4.754512900091780736 ) ) ;
#30153=CARTESIAN_POINT ( 'NONE',  ( 7.507395534388972891, -77.29994500668442470, 5.452647970045330972 ) ) ;
#30154=CARTESIAN_POINT ( 'NONE',  ( 9.611650271896829523, -77.99166666666667425, 5.539808784079915505 ) ) ;
#30156=CARTESIAN_POINT ( 'NONE',  ( -4.515747639259999779, -79.58700506441199707, 10.32167056182999865 ) ) ;
#30181=CARTESIAN_POINT ( 'NONE',  ( -5.722401730670302555, -77.52815347229775966, 7.267916609703462427 ) ) ;
#30182=CARTESIAN_POINT ( 'NONE',  ( -10.79754810892000094, -77.38656070981998880, -2.301543980133000211 ) ) ;
#30183=DIRECTION ( 'NONE',  ( 0.000000000000000000, -1.000000000000000000, 0.000000000000000000 ) ) ;
#30185=CARTESIAN_POINT ( 'NONE',  ( 1.487026788147999934, -77.40709090636698875, -9.589549613196998834 ) ) ;
#30187=ADVANCED_FACE ( 'NONE', ( #34044 ), #57255, .T. ) ;
#30190=CARTESIAN_POINT ( 'NONE',  ( -11.09141466634999951, -79.97688649776199554, 1.909950515085000022 ) ) ;
#30201=CARTESIAN_POINT ( 'NONE',  ( -10.75000000000000000, -80.44999999999998863, 5.225043809877999334E-10 ) ) ;
#30204=CARTESIAN_POINT ( 'NONE',  ( -10.93859554520000010, -80.49215799716398578, 0.1126871859218999961 ) ) ;
#30208=CARTESIAN_POINT ( 'NONE',  ( 5.539808784079868431, -80.03333333334234112, 9.611650271896850839 ) ) ;
#30209=ORIENTED_EDGE ( 'NONE', *, *, #18299, .T. ) ;
#30215=CARTESIAN_POINT ( 'NONE',  ( 5.959432220885000575, -79.34133969600698322, 7.301460587826000825 ) ) ;
#30217=CARTESIAN_POINT ( 'NONE',  ( 0.8674776458591695327, -77.23125000000000284, -10.99972142223460736 ) ) ;
#30223=EDGE_CURVE ( 'NONE', #3255, #4702, #51642, .T. ) ;
#30224=CARTESIAN_POINT ( 'NONE',  ( 5.463250847760000362, -77.20323840584198649, 9.217959235020000364 ) ) ;
#30231=CARTESIAN_POINT ( 'NONE',  ( -9.429275737370000243, -77.21926183160998391, -1.157047565421999824 ) ) ;
#30232=CARTESIAN_POINT ( 'NONE',  ( 9.009247259181925926, -78.27083333333331439, 2.421167930323317119 ) ) ;
#30233=CARTESIAN_POINT ( 'NONE',  ( 8.796335266379966100, -77.40208333333333712, 6.760013919724084275 ) ) ;
#30245=ORIENTED_EDGE ( 'NONE', *, *, #18720, .F. ) ;
#30254=CARTESIAN_POINT ( 'NONE',  ( 2.421167930323352646, -79.64583333333334281, -9.009247259181915268 ) ) ;
#30257=DIRECTION ( 'NONE',  ( 0.000000000000000000, -1.000000000000000000, 0.000000000000000000 ) ) ;
#30263=CARTESIAN_POINT ( 'NONE',  ( -0.5065304950087446967, -77.22907666195568765, 9.658864201383851267 ) ) ;
#30265=CARTESIAN_POINT ( 'NONE',  ( -8.627689810547352067, -78.62938668033045531, -3.338956675450427181 ) ) ;
#30272=DIRECTION ( 'NONE',  ( 0.000000000000000000, -1.000000000000000000, 0.000000000000000000 ) ) ;
#30280=ADVANCED_FACE ( 'NONE', ( #46798 ), #30415, .F. ) ;
#30285=CARTESIAN_POINT ( 'NONE',  ( 10.49999999996000000, -76.19999999995870610, 1.566655805052999811E-09 ) ) ;
#30289=CARTESIAN_POINT ( 'NONE',  ( -9.497876546326999403, -77.25168256874098915, -0.2008509664869000122 ) ) ;
#30294=CARTESIAN_POINT ( 'NONE',  ( -9.070848764158998989, -77.36923613374699471, 2.805586010018000120 ) ) ;
#30302=CARTESIAN_POINT ( 'NONE',  ( 9.949629901056999515, -78.65493811345498898, 4.548920879513999260 ) ) ;
#30304=CARTESIAN_POINT ( 'NONE',  ( -11.08184087837999954, -80.35837970449398426, 1.745757554832999991 ) ) ;
#30305=VERTEX_POINT ( 'NONE', #54103 ) ;
#30322=DIRECTION ( 'NONE',  ( -1.000000000000000000, 0.000000000000000000, 0.000000000000000000 ) ) ;
#30326=CARTESIAN_POINT ( 'NONE',  ( 8.555152029244165846, -78.81910539201572874, -3.517135500673375326 ) ) ;
#30331=CARTESIAN_POINT ( 'NONE',  ( 7.999999997059999757, -81.20000000293998710, 1.734976716005999945E-08 ) ) ;
#30338=CARTESIAN_POINT ( 'NONE',  ( 8.932658457838000388, -77.29554552857699434, 2.869163408763999890 ) ) ;
#30352=CARTESIAN_POINT ( 'NONE',  ( -9.498944747049275605, -79.25084052136060109, -0.1003342093385300032 ) ) ;
#30354=CYLINDRICAL_SURFACE ( 'NONE', #38893, 11.00000000000000000 ) ;
#30358=CARTESIAN_POINT ( 'NONE',  ( 1.514375715454999938, -79.63358191161798061, 9.774571951410999660 ) ) ;
#30369=CARTESIAN_POINT ( 'NONE',  ( 3.535831105395000229, -77.07998060082339009, -10.52352073039000047 ) ) ;
#30377=CONICAL_SURFACE ( 'NONE', #25669, 10.59999999995999964, 0.7853981633972997312 ) ;
#30378=CARTESIAN_POINT ( 'NONE',  ( 8.249323304235000265, -79.91458346929098866, -5.229696851825000437 ) ) ;
#30387=CARTESIAN_POINT ( 'NONE',  ( 9.508279846913755051, -79.09345843291232825, -0.7695542747135521999 ) ) ;
#30395=CARTESIAN_POINT ( 'NONE',  ( 1.436206387574776588, -79.96308954466168473, 9.137514757049482128 ) ) ;
#30398=CARTESIAN_POINT ( 'NONE',  ( -4.515747639259999779, -80.02863228676199014, 10.32167056182999865 ) ) ;
#30399=CARTESIAN_POINT ( 'NONE',  ( 9.249995191645682624, -77.35005069067575789, 0.005711754169352296386 ) ) ;
#30407=CARTESIAN_POINT ( 'NONE',  ( -6.760013919724099374, -78.52708333333332291, 8.796335266379958995 ) ) ;
#30409=CARTESIAN_POINT ( 'NONE',  ( -4.392572548605500060, -80.45000000000000284, -9.875985572387369515 ) ) ;
#30410=CARTESIAN_POINT ( 'NONE',  ( -3.734118835908999845, -79.45909416798998848, 10.51417881607000027 ) ) ;
#30415=B_SPLINE_SURFACE_WITH_KNOTS ( 'NONE', 3, 3, ( 
 ( #55628, #25484, #57645, #3912, #47670, #43504, #43802, #11920, #29898, #2774, #7196, #8058, #57364, #21632, #25198, #39356, #48238, #53220, #44358 ),
 ( #26053, #21914, #3628, #47956, #20774, #13052, #16926, #35480, #48511, #57937, #52937, #57075, #21060, #38775, #44078, #34333, #7487, #34906, #21344 ),
 ( #3064, #12485, #25776, #3348, #39637, #56793, #34621, #16353, #52367, #30485, #8344, #39061, #53511, #17200, #16637, #7774, #52650, #43218, #17493 ),
 ( #35188, #12204, #30190, #12768, #30764, #48797, #26340, #39923, #5377, #8637, #50265, #58231, #40221, #45252, #31344, #32223, #27507, #45843, #26623 ) ),
 .UNSPECIFIED., .F., .F., .F.,
 ( 4, 4 ),
 ( 4, 1, 1, 1, 1, 1, 1, 1, 1, 1, 1, 1, 1, 1, 1, 1, 4 ),
 ( -0.4045438850611000059, 1.404543885061000141 ),
 ( -0.007432834721512999662, 0.01672387812341000202, 0.04088059096832000194, 0.06503730381324000775, 0.08919401665815999969, 0.1133507295031000034, 0.1375074423479999974, 0.1616641551929000054, 0.1858208680378000133, 0.2099775808827999968, 0.2341342937277000047, 0.2582910065726000126, 0.2824477194174999650, 0.3066044322623999729, 0.3307611451072999809, 0.3549178579523000199, 0.3790745707971999723 ),
 .UNSPECIFIED. ) ;
#30436=ADVANCED_FACE ( 'NONE', ( #8934 ), #58226, .F. ) ;
#30438=CARTESIAN_POINT ( 'NONE',  ( 9.233664981878000333, -79.66529779542098311, 5.933249305785000871 ) ) ;
#30446=CARTESIAN_POINT ( 'NONE',  ( -2.879226727952072018, -77.70416666666665151, -10.71369944335147295 ) ) ;
#30447=CARTESIAN_POINT ( 'NONE',  ( 8.267239500339000458, -78.00112293168498923, -6.983083964283999912 ) ) ;
#30449=CARTESIAN_POINT ( 'NONE',  ( 11.00000000000000000, -79.94999999999998863, 0.000000000000000000 ) ) ;
#30458=B_SPLINE_CURVE_WITH_KNOTS ( 'NONE', 3,
 ( #46906, #26447, #8170, #26172, #44470, #44191, #25593, #3737, #56901, #7877, #17609, #30592, #40034, #35012, #39169, #3174, #20878, #48623, #16458, #48062, #39464, #43613, #53045, #43323 ),
 .UNSPECIFIED., .F., .F.,
 ( 4, 2, 1, 2, 2, 2, 2, 2, 2, 2, 1, 2, 4 ),
 ( 0.000000000000000000, 0.06250000000000001388, 0.1250000000000000278, 0.1875000000000000555, 0.2500000000000000555, 0.3750000000000000000, 0.5000000000000000000, 0.6250000000000000000, 0.7500000000000000000, 0.8125000000000001110, 0.8750000000000001110, 0.9375000000000001110, 1.000000000000000000 ),
 .UNSPECIFIED. ) ;
#30465=CARTESIAN_POINT ( 'NONE',  ( -8.224854987054504463, -79.70792932115747931, 4.804646458694507238 ) ) ;
#30472=EDGE_CURVE ( 'NONE', #27909, #33815, #30037, .T. ) ;
#30478=CARTESIAN_POINT ( 'NONE',  ( -7.485639807788073696, -77.55002885482164743, 5.433928319481235114 ) ) ;
#30479=CARTESIAN_POINT ( 'NONE',  ( 10.90987126150000108, -77.13208304049749131, 1.690571823134000118 ) ) ;
#30481=CARTESIAN_POINT ( 'NONE',  ( 4.186942200393000135, -78.49065168068099752, -8.754440266352000677 ) ) ;
#30485=CARTESIAN_POINT ( 'NONE',  ( 10.52776997023000050, -80.20891172946198822, 3.979665013433000720 ) ) ;
#30497=CARTESIAN_POINT ( 'NONE',  ( -8.343537481004000611, -80.56114086983298250, 7.770819240183000076 ) ) ;
#30508=CARTESIAN_POINT ( 'NONE',  ( 10.02153394804916786, -77.66944384051467409, -4.123993692972488745 ) ) ;
#30510=CARTESIAN_POINT ( 'NONE',  ( 3.411343139177948736, -77.25000000000000000, -10.49328960906044728 ) ) ;
#30515=CARTESIAN_POINT ( 'NONE',  ( 5.539808784079907511, -77.36666666666666003, -9.611650271896827746 ) ) ;
#30521=CARTESIAN_POINT ( 'NONE',  ( -9.429275737370000243, -77.27956475728099406, -1.157047565421999824 ) ) ;
#30529=CARTESIAN_POINT ( 'NONE',  ( -7.999999997059999757, -81.20000000293998710, -1.734976707327999832E-08 ) ) ;
#30539=EDGE_CURVE ( 'NONE', #25733, #3055, #1264, .T. ) ;
#30560=CARTESIAN_POINT ( 'NONE',  ( -8.768304182600733299, -78.62583989957664699, -2.946665245982536430 ) ) ;
#30580=VERTEX_POINT ( 'NONE', #40606 ) ;
#30586=CARTESIAN_POINT ( 'NONE',  ( -9.212293474215000444, -77.41660918229499089, -2.808383990684999887 ) ) ;
#30592=CARTESIAN_POINT ( 'NONE',  ( -1.255428910056382685, -78.98621335419240097, 9.244592359588491348 ) ) ;
#30596=CARTESIAN_POINT ( 'NONE',  ( -9.062201444876000878, -78.82349223945099936, 6.128973919716999674 ) ) ;
#30598=CARTESIAN_POINT ( 'NONE',  ( -4.083745399801999909, -80.14710589224999637, 10.68783448605000075 ) ) ;
#30601=ORIENTED_EDGE ( 'NONE', *, *, #10495, .F. ) ;
#30603=DIRECTION ( 'NONE',  ( -1.000000000000000000, 0.000000000000000000, 0.000000000000000000 ) ) ;
#30604=CARTESIAN_POINT ( 'NONE',  ( -9.358268528169000788, -79.77312495323751307, -2.797054701638000296 ) ) ;
#30619=DIRECTION ( 'NONE',  ( 1.000000000000000000, 0.000000000000000000, 0.000000000000000000 ) ) ;
#30624=CARTESIAN_POINT ( 'NONE',  ( 8.796335266379966100, -77.90208333333333712, 6.760013919724084275 ) ) ;
#30643=CARTESIAN_POINT ( 'NONE',  ( -9.497892349503649356, -79.25146880129915417, -0.1753275914303987493 ) ) ;
#30645=CARTESIAN_POINT ( 'NONE',  ( 8.796335266379966100, -78.90208333333333712, 6.760013919724084275 ) ) ;
#30648=CARTESIAN_POINT ( 'NONE',  ( -0.2763518505204999864, -79.08418661348099477, 9.776846056101000215 ) ) ;
#30650=CARTESIAN_POINT ( 'NONE',  ( 2.600000000000000089, -78.49999999999998579, 0.000000000000000000 ) ) ;
#30663=EDGE_CURVE ( 'NONE', #14347, #3055, #29054, .T. ) ;
#30664=CARTESIAN_POINT ( 'NONE',  ( 6.728605944993000243, -79.45532386283399262, -7.080011783993000130 ) ) ;
#30673=CARTESIAN_POINT ( 'NONE',  ( -7.203509393524943683, -78.90833944987893744, -6.502559514027580256 ) ) ;
#30680=CARTESIAN_POINT ( 'NONE',  ( 3.538814480809993945, -79.94385127736886432, 8.546238217284953365 ) ) ;
#30684=CARTESIAN_POINT ( 'NONE',  ( 0.2682802194768000303, -79.74770874343499827, -11.26307951182000089 ) ) ;
#30695=CARTESIAN_POINT ( 'NONE',  ( 0.9241086513771999966, -78.92533943566898813, 11.11924560648999893 ) ) ;
#30719=CARTESIAN_POINT ( 'NONE',  ( -4.985523414424999800, -78.51762948478699400, -9.777963635945001286 ) ) ;
#30730=CARTESIAN_POINT ( 'NONE',  ( -9.595360835209000072, -79.28568019887099183, -5.693913425678999829 ) ) ;
#30742=AXIS2_PLACEMENT_3D ( 'NONE', #52296, #30122, #29833 ) ;
#30752=CARTESIAN_POINT ( 'NONE',  ( -6.180994592422803358, -78.16689241883609895, -6.883246697956296067 ) ) ;
#30755=EDGE_LOOP ( 'NONE', ( #12610, #17849, #244 ) ) ;
#30757=CARTESIAN_POINT ( 'NONE',  ( -6.466212988017749019, -77.53676806074847150, 6.615100391815839309 ) ) ;
#30758=CARTESIAN_POINT ( 'NONE',  ( -10.79754810892000094, -77.32625778414998763, -2.301543980133000211 ) ) ;
#30764=CARTESIAN_POINT ( 'NONE',  ( -7.179058446792000225, -80.06040882843898032, -8.667882172381000672 ) ) ;
#30793=FACE_OUTER_BOUND ( 'NONE', #45458, .T. ) ;
#30804=CARTESIAN_POINT ( 'NONE',  ( 9.100722152916000951, -77.11296757197209217, -3.274758550341999808 ) ) ;
#30821=ORIENTED_EDGE ( 'NONE', *, *, #6959, .T. ) ;
#30828=VERTEX_POINT ( 'NONE', #8946 ) ;
#30829=CARTESIAN_POINT ( 'NONE',  ( 3.792698199283999649, -78.00290701960965123, -10.36819406884000117 ) ) ;
#30832=VERTEX_POINT ( 'NONE', #32521 ) ;
#30833=DIRECTION ( 'NONE',  ( 0.000000000000000000, 0.000000000000000000, -1.000000000000000000 ) ) ;
#30837=CARTESIAN_POINT ( 'NONE',  ( -9.311105030178968178, -77.13820107031234841, -0.1312602372466275813 ) ) ;
#30843=CARTESIAN_POINT ( 'NONE',  ( -9.056035971749563984, -78.61657572224720525, -1.894306744419020250 ) ) ;
#30853=CYLINDRICAL_SURFACE ( 'NONE', #48063, 9.250000000000000000 ) ;
#30855=CARTESIAN_POINT ( 'NONE',  ( 1.439896632895334649, -79.33541666666666003, -10.99999999999999822 ) ) ;
#30866=CONICAL_SURFACE ( 'NONE', #41261, 9.649999999948999374, 0.7853981633972997312 ) ;
#30869=CARTESIAN_POINT ( 'NONE',  ( 4.939304878001000709, -78.85185680379399287, 8.013392654152999839 ) ) ;
#30883=CARTESIAN_POINT ( 'NONE',  ( -9.522411774477998136, -79.76552920275499048, 5.478866733777000952 ) ) ;
#30890=CARTESIAN_POINT ( 'NONE',  ( 6.653382217586999658, -80.06537887755254701, 7.150748904218000135 ) ) ;
#30902=CARTESIAN_POINT ( 'NONE',  ( 9.075776011423059231, -78.83460089325743070, -1.786594630451423971 ) ) ;
#30906=LINE ( 'NONE', #17345, #41724 ) ;
#30916=CARTESIAN_POINT ( 'NONE',  ( -9.549999999999998934, -79.99999999999998579, 0.000000000000000000 ) ) ;
#30923=EDGE_CURVE ( 'NONE', #7174, #23068, #16448, .T. ) ;
#30931=CARTESIAN_POINT ( 'NONE',  ( -9.666799225812999552, -79.71909680386698938, -1.488628203271999961 ) ) ;
#30943=CARTESIAN_POINT ( 'NONE',  ( -8.488829372234999227, -77.37345827014598854, 7.154399614211999214 ) ) ;
#30949=CARTESIAN_POINT ( 'NONE',  ( 9.202039358297998461, -80.10013463714798831, 2.360608321670000453 ) ) ;
#30966=CARTESIAN_POINT ( 'NONE',  ( -0.1991013119907288076, -79.97697863826387277, 9.262774322989109521 ) ) ;
#30967=FACE_OUTER_BOUND ( 'NONE', #37297, .T. ) ;
#30969=CARTESIAN_POINT ( 'NONE',  ( 3.390474011741000382, -79.27013871977898418, -10.74400392503999946 ) ) ;
#30978=CARTESIAN_POINT ( 'NONE',  ( 6.829411927397999627, -79.23435533332899183, -8.823306204757001225 ) ) ;
#30982=CARTESIAN_POINT ( 'NONE',  ( 0.000000000000000000, -81.89999999962999766, 0.000000000000000000 ) ) ;
#30988=CARTESIAN_POINT ( 'NONE',  ( 9.249483092228999226, -79.25084128437099196, 0.09778817195952001218 ) ) ;
#30995=CARTESIAN_POINT ( 'NONE',  ( 4.657000555087000393, -77.30872832793998839, -8.305583776142999142 ) ) ;
#31000=CARTESIAN_POINT ( 'NONE',  ( 8.082524092276875294, -78.79166666666665719, 4.658475568430836766 ) ) ;
#31004=EDGE_CURVE ( 'NONE', #2177, #43339, #52592, .T. ) ;
#31006=CARTESIAN_POINT ( 'NONE',  ( -10.69701368780000017, -79.92224720141999228, 1.066019776055000090 ) ) ;
#31017=CARTESIAN_POINT ( 'NONE',  ( 3.357763675545999860, -78.89238723821299004, -10.64034880800999971 ) ) ;
#31024=CARTESIAN_POINT ( 'NONE',  ( 9.469145113845355510, -79.49323344442748862, 5.723973398464534235 ) ) ;
#31028=LINE ( 'NONE', #8615, #14539 ) ;
#31037=CARTESIAN_POINT ( 'NONE',  ( -5.053239713898484808, -78.17904410541564175, -7.747788339080754483 ) ) ;
#31042=CARTESIAN_POINT ( 'NONE',  ( 2.855611011456188120, -77.45020245399071257, 8.798067008888779128 ) ) ;
#31043=CARTESIAN_POINT ( 'NONE',  ( -6.065106684382000068, -77.29113158382398296, 9.224892016835999797 ) ) ;
#31046=CARTESIAN_POINT ( 'NONE',  ( 7.890274420948999001, -79.09100735980197783, -5.649267206312000411 ) ) ;
#31052=CARTESIAN_POINT ( 'NONE',  ( -9.250000000000000000, -77.59999999999999432, 0.000000000000000000 ) ) ;
#31064=CARTESIAN_POINT ( 'NONE',  ( 8.563134967179999890, -80.25043697167899381, -7.360427151328000406 ) ) ;
#31076=CARTESIAN_POINT ( 'NONE',  ( 11.00000000000000000, -77.34999999999999432, 0.000000000000000000 ) ) ;
#31088=CARTESIAN_POINT ( 'NONE',  ( -0.5065222552852000071, -77.26962377378099234, 9.658707080791000266 ) ) ;
#31092=CARTESIAN_POINT ( 'NONE',  ( 0.000000000000000000, -76.89999999999999147, 0.000000000000000000 ) ) ;
#31118=CARTESIAN_POINT ( 'NONE',  ( -3.536681740116999872, -78.11423136717898785, 9.036735673663999435 ) ) ;
#31131=DIRECTION ( 'NONE',  ( -1.000000000000000000, 0.000000000000000000, 0.000000000000000000 ) ) ;
#31132=DIRECTION ( 'NONE',  ( 0.000000000000000000, -1.000000000000000000, 9.256484467811999056E-14 ) ) ;
#31148=EDGE_CURVE ( 'NONE', #39698, #34245, #26249, .T. ) ;
#31152=CARTESIAN_POINT ( 'NONE',  ( 8.959721679174998954, -77.67945172698098588, -3.223936051704999972 ) ) ;
#31158=EDGE_LOOP ( 'NONE', ( #19367, #34508, #39689, #13989 ) ) ;
#31165=CARTESIAN_POINT ( 'NONE',  ( 0.2605153439964000284, -79.49770874343499827, -10.93709047653000077 ) ) ;
#31167=CARTESIAN_POINT ( 'NONE',  ( 7.000000000000000000, -80.99999999999998579, 0.000000000000000000 ) ) ;
#31181=B_SPLINE_CURVE_WITH_KNOTS ( 'NONE', 3,
 ( #44957, #57942, #116, #48801, #8061, #40816, #34908, #8347, #18094, #53514, #39926, #52940, #26056, #54107, #3632, #21636, #8642, #35192 ),
 .UNSPECIFIED., .F., .F.,
 ( 4, 2, 2, 2, 2, 2, 2, 2, 4 ),
 ( 0.000000000000000000, 0.1250000000000000278, 0.2500000000000000555, 0.3750000000000001665, 0.5000000000000001110, 0.6250000000000001110, 0.7500000000000002220, 0.8750000000000001110, 1.000000000000000000 ),
 .UNSPECIFIED. ) ;
#31182=DIRECTION ( 'NONE',  ( -1.000000000000000000, 0.000000000000000000, 0.000000000000000000 ) ) ;
#31195=CARTESIAN_POINT ( 'NONE',  ( 10.99999999999999645, -77.86041666666663730, 1.439896632895345974 ) ) ;
#31204=FACE_OUTER_BOUND ( 'NONE', #36218, .T. ) ;
#31205=DIRECTION ( 'NONE',  ( 0.000000000000000000, 0.000000000000000000, -1.000000000000000000 ) ) ;
#31210=CARTESIAN_POINT ( 'NONE',  ( -5.000000000000000000, -75.19999999999998863, 0.000000000000000000 ) ) ;
#31214=EDGE_LOOP ( 'NONE', ( #19893, #51770, #56810, #43026 ) ) ;
#31222=CARTESIAN_POINT ( 'NONE',  ( -4.491587152465999822, -78.91604404360498393, -8.642068059767000321 ) ) ;
#31233=ORIENTED_EDGE ( 'NONE', *, *, #22348, .T. ) ;
#31234=CARTESIAN_POINT ( 'NONE',  ( -4.420137786970999905, -77.33677356148098170, 10.18371445122000019 ) ) ;
#31242=CARTESIAN_POINT ( 'NONE',  ( 9.630577183392999174, -79.03317930548099923, 1.628483183780000010 ) ) ;
#31244=ORIENTED_EDGE ( 'NONE', *, *, #12890, .T. ) ;
#31248=VERTEX_POINT ( 'NONE', #49624 ) ;
#31250=CARTESIAN_POINT ( 'NONE',  ( -9.627143703009355846, -78.33986286729894744, 1.221446647086100734 ) ) ;
#31254=CARTESIAN_POINT ( 'NONE',  ( -8.000000000000000000, -81.19999999999998863, 0.000000000000000000 ) ) ;
#31258=CARTESIAN_POINT ( 'NONE',  ( 8.698361121289734044, -79.87801218299412653, 3.168218995563596430 ) ) ;
#31259=CARTESIAN_POINT ( 'NONE',  ( 4.505934350724444926, -80.10858973450639553, -10.15323451728369797 ) ) ;
#31261=CARTESIAN_POINT ( 'NONE',  ( -0.5065222552852000071, -77.12916933416629206, 9.658707080791000266 ) ) ;
#31269=CARTESIAN_POINT ( 'NONE',  ( -10.30593458266999995, -78.58823118367698157, -4.275431210322000020 ) ) ;
#31296=CARTESIAN_POINT ( 'NONE',  ( 10.31626776183999894, -78.21273180413199100, -3.746764721243999841 ) ) ;
#31297=CARTESIAN_POINT ( 'NONE',  ( 0.000000000000000000, -76.19999999999998863, 0.000000000000000000 ) ) ;
#31300=CARTESIAN_POINT ( 'NONE',  ( -10.35238666240951844, -79.67168035550133709, 3.845238516216011870 ) ) ;
#31306=CARTESIAN_POINT ( 'NONE',  ( -5.539808784079886195, -77.68333333333333712, -9.611650271896841957 ) ) ;
#31308=CARTESIAN_POINT ( 'NONE',  ( 11.05620287758999964, -79.48232667919899086, -1.500659051079999973 ) ) ;
#31317=ORIENTED_EDGE ( 'NONE', *, *, #44317, .F. ) ;
#31318=VERTEX_POINT ( 'NONE', #51276 ) ;
#31322=CARTESIAN_POINT ( 'NONE',  ( 4.096584555840107278, -79.58967318748072728, 8.607303473720193665 ) ) ;
#31328=CARTESIAN_POINT ( 'NONE',  ( -6.347401566831289976, -78.16496885166350239, -6.728806251054260557 ) ) ;
#31333=EDGE_CURVE ( 'NONE', #31523, #3819, #12864, .T. ) ;
#31334=ORIENTED_EDGE ( 'NONE', *, *, #24763, .T. ) ;
#31335=CARTESIAN_POINT ( 'NONE',  ( 1.422220956165613170, -77.46272989785457241, 9.140013063714238939 ) ) ;
#31336=CARTESIAN_POINT ( 'NONE',  ( -9.050627908549000011, -77.47867334415599316, -6.322205650057999726 ) ) ;
#31339=CARTESIAN_POINT ( 'NONE',  ( 9.690463944985998168, -78.63622609373899763, -0.5153813127049999832 ) ) ;
#31344=CARTESIAN_POINT ( 'NONE',  ( -11.11771682179999843, -80.47802048182499846, 1.751409206030000165 ) ) ;
#31357=DIRECTION ( 'NONE',  ( 0.000000000000000000, 1.000000000000000000, 0.000000000000000000 ) ) ;
#31363=CARTESIAN_POINT ( 'NONE',  ( -2.879226727952121312, -80.09583333334906285, 10.71369944335146052 ) ) ;
#31372=CARTESIAN_POINT ( 'NONE',  ( 10.89775144040313215, -77.33749999999999147, -1.727831697829316893 ) ) ;
#31373=EDGE_CURVE ( 'NONE', #21042, #16896, #40504, .T. ) ;
#31374=CARTESIAN_POINT ( 'NONE',  ( 0.000000000000000000, -75.19999999999998863, 0.000000000000000000 ) ) ;
#31395=CARTESIAN_POINT ( 'NONE',  ( 2.879226727952084897, -79.45416666666667993, 10.71369944335147295 ) ) ;
#31418=B_SPLINE_SURFACE_WITH_KNOTS ( 'NONE', 3, 3, ( 
 ( #22083, #40097, #17971, #9406, #58110, #27100, #17673, #53689, #31222, #22981, #40399, #49260, #53987, #8812, #45137, #35963, #4687, #26804, #13526, #31518, #49567, #9696, #9113, #22686, #291, #18270, #36262, #54285, #13822, #31821, #582, #33574, #1729, #29144, #47190, #15579, #11169, #19431, #2023, #32690, #50740, #33278, #6722, #28261, #51612, #24730, #32982, #28848, #42743, #55740, #14985, #15870, #46899, #33856, #2306, #38298, #6426, #24441, #20303, #42455, #23846, #20021, #55143, #6134, #51894, #38004, #56320 ),
 ( #19137, #56030, #10281, #27974, #46024, #55443, #5545, #37132, #51028, #46315, #24141, #23555, #14689, #10577, #5840, #41571, #1152, #15284, #41863, #19722, #51319, #37718, #1440, #37423, #28560, #46608, #10877, #42160, #34142, #38589, #3445, #20872, #52182, #21449, #16164, #3731, #2874, #17306, #16452, #48617, #34433, #11737, #12304, #57749, #38875, #56604, #29431, #39164, #44184, #43032, #7298, #29715, #26165, #21732, #47763, #8164, #11452, #39739, #57462, #20592, #17023, #43901, #52750, #30586, #35292, #30294, #39458 ),
 ( #47483, #48333, #7872, #7009, #25874, #25300, #35007, #43318, #48056, #25011, #53040, #2593, #16739, #56895, #52463, #12021, #12587, #30002, #7587, #25586, #43608, #3168, #21158, #57173, #34720, #49494, #27327, #44463, #40331, #53618, #45656, #50084, #40629, #41205, #27029, #18202, #45066, #8743, #13747, #35590, #4014, #22617, #224, #17601, #22020, #45361, #4314, #13156, #4910, #58041, #5198, #44765, #795, #58340, #32039, #17903, #31152, #54212, #18777, #22314, #40028, #12867, #36194, #27616, #26441, #49191, #26734 ),
 ( #35892, #9628, #53923, #4618, #13456, #48905, #53322, #31452, #23200, #9338, #9043, #40921, #22909, #54508, #31747, #49792, #510, #30869, #18486, #36479, #8445, #14045, #24371, #55368, #24070, #24661, #42383, #41498, #1953, #19947, #19646, #6649, #14912, #51540, #1083, #45948, #54787, #37935, #55076, #11097, #19070, #14623, #51250, #32326, #42670, #32615, #50666, #33504, #29077, #47122, #2238, #10209, #5769, #41791, #36769, #15211, #42087, #50373, #9920, #27901, #10504, #1656, #5479, #23485, #28188, #23776, #1363 ) ),
 .UNSPECIFIED., .F., .F., .F.,
 ( 4, 4 ),
 ( 4, 1, 1, 1, 1, 1, 1, 1, 1, 1, 1, 1, 1, 1, 1, 1, 1, 1, 1, 1, 1, 1, 1, 1, 1, 1, 1, 1, 1, 1, 1, 1, 1, 1, 1, 1, 1, 1, 1, 1, 1, 1, 1, 1, 1, 1, 1, 1, 1, 1, 1, 1, 1, 1, 1, 1, 1, 1, 1, 1, 1, 1, 1, 1, 4 ),
 ( -0.1387574078320000237, 1.138757407831999968 ),
 ( -0.02000000000000000042, -0.003749999999999999861, 0.01250000000000000069, 0.02875000000000000125, 0.04499999999999999833, 0.06124999999999999889, 0.07749999999999999944, 0.09375000000000000000, 0.1100000000000000006, 0.1262500000000000011, 0.1424999999999999878, 0.1587500000000000022, 0.1749999999999999889, 0.1912500000000000033, 0.2074999999999999900, 0.2237500000000000044, 0.2399999999999999911, 0.2562499999999999778, 0.2725000000000000200, 0.2887500000000000067, 0.3049999999999999933, 0.3212499999999999800, 0.3375000000000000222, 0.3537500000000000089, 0.3699999999999999956, 0.3862499999999999822, 0.4025000000000000244, 0.4187500000000000111, 0.4349999999999999978, 0.4512499999999999845, 0.4675000000000000266, 0.4837500000000000133, 0.5000000000000000000, 0.5162499999999999867, 0.5324999999999999734, 0.5487499999999999600, 0.5649999999999999467, 0.5812500000000000444, 0.5975000000000000311, 0.6137500000000000178, 0.6300000000000000044, 0.6462499999999999911, 0.6624999999999999778, 0.6787499999999999645, 0.6949999999999999512, 0.7112500000000000488, 0.7275000000000000355, 0.7437500000000000222, 0.7600000000000000089, 0.7762499999999999956, 0.7924999999999999822, 0.8087499999999999689, 0.8249999999999999556, 0.8412500000000000533, 0.8575000000000000400, 0.8737500000000000266, 0.8900000000000000133, 0.9062500000000000000, 0.9224999999999999867, 0.9387499999999999734, 0.9549999999999999600, 0.9712499999999999467, 0.9875000000000000444, 1.003749999999999920, 1.020000000000000018 ),
 .UNSPECIFIED. ) ;
#31420=CARTESIAN_POINT ( 'NONE',  ( -7.203390125892000562, -78.76797943714498729, -6.502451851937000704 ) ) ;
#31422=FACE_BOUND ( 'NONE', #7003, .T. ) ;
#31434=AXIS2_PLACEMENT_3D ( 'NONE', #4149, #40460, #51 ) ;
#31439=VERTEX_POINT ( 'NONE', #47721 ) ;
#31452=CARTESIAN_POINT ( 'NONE',  ( -1.146763852601999867, -79.13609509508398787, -9.343239705575001608 ) ) ;
#31467=CLOSED_SHELL ( 'NONE', ( #6465, #36270, #40556, #51546, #7891, #7311, #13849, #47798, #48449, #36540, #24418, #42817, #35173, #49631, #50992, #1509, #21707, #33747, #38378, #19507, #2792, #34386, #56950, #9142, #591, #54238, #41490, #48337, #56691, #9424, #38335, #8986, #51664, #49199, #51159, #56044, #28481, #4712, #44804, #17107, #15780, #20180, #6684, #30187, #55419, #11962, #39202, #2979, #33266, #35329, #11530, #45511, #34725, #49777, #1823, #42839, #17883, #19895, #4874, #18444, #27278, #30436, #13691, #51527, #26019, #30280, #53489, #43074, #24950, #53177, #7242, #12149, #36937, #32596, #39626, #48068, #42977, #21623, #52351, #13511, #4674, #41652, #46786, #29806, #36567, #44400, #16466, #28228, #36144, #24906, #16566, #50504, #53700, #38738, #28748, #37961, #33306, #42241, #40189, #922, #35792, #40125, #26207, #52808, #10699, #9057, #52369, #13464, #42827, #47531, #36212, #4653, #39873, #3705, #44259, #21049, #24250 ) ) ;
#31482=VECTOR ( 'NONE', #53290, 1000.000000000000000 ) ;
#31485=CARTESIAN_POINT ( 'NONE',  ( 0.1338524678202104856, -78.72631179971439508, -9.249082273563699275 ) ) ;
#31502=CYLINDRICAL_SURFACE ( 'NONE', #21229, 4.100000000000000533 ) ;
#31515=CARTESIAN_POINT ( 'NONE',  ( -8.841085912879560027, -79.99999999999998579, -2.882805647535432669 ) ) ;
#31518=CARTESIAN_POINT ( 'NONE',  ( 9.292856425461000214, -78.60338192318698702, 2.915907262279999745 ) ) ;
#31523=VERTEX_POINT ( 'NONE', #25109 ) ;
#31534=CARTESIAN_POINT ( 'NONE',  ( -1.529773069620000037, -77.10717163294118848, -11.10696160730999971 ) ) ;
#31542=CARTESIAN_POINT ( 'NONE',  ( 9.534323188421000239, -78.95122794097099472, -1.008198710029000189 ) ) ;
#31554=CARTESIAN_POINT ( 'NONE',  ( 7.006148741439892191, -79.90670744298051886, 6.039518869995502470 ) ) ;
#31555=CYLINDRICAL_SURFACE ( 'NONE', #32175, 9.250000000000000000 ) ;
#31557=CARTESIAN_POINT ( 'NONE',  ( -10.85153605587000136, -80.10354523164899376, 2.386335476490000218 ) ) ;
#31558=CARTESIAN_POINT ( 'NONE',  ( 2.859706235832604193, -77.25018302167970319, -8.796733326739918368 ) ) ;
#31563=B_SPLINE_CURVE_WITH_KNOTS ( 'NONE', 3,
 ( #24475, #42489, #2059, #56070, #15614, #33609, #51652, #11203, #29179, #47226, #6757, #24767, #42779, #20336, #38331, #56355, #12055, #13194 ),
 .UNSPECIFIED., .F., .F.,
 ( 4, 2, 2, 2, 2, 2, 2, 2, 4 ),
 ( 0.000000000000000000, 0.1250000000000000000, 0.2500000000000000000, 0.3750000000000000000, 0.5000000000000000000, 0.6250000000000000000, 0.7500000000000000000, 0.8750000000000000000, 1.000000000000000000 ),
 .UNSPECIFIED. ) ;
#31593=CARTESIAN_POINT ( 'NONE',  ( 9.304500756975000897, -79.13566128010499767, -5.821536072646999571 ) ) ;
#31601=CARTESIAN_POINT ( 'NONE',  ( 11.00000000000000000, -77.94999999999998863, 0.000000000000000000 ) ) ;
#31606=CARTESIAN_POINT ( 'NONE',  ( 1.695617993698999904, -78.16967705768098540, 10.91800231797999921 ) ) ;
#31611=CARTESIAN_POINT ( 'NONE',  ( -9.250000000000000000, -79.99999999999998579, 2.662757480928999879E-14 ) ) ;
#31612=CARTESIAN_POINT ( 'NONE',  ( -5.239266479141340582, -79.61428708882451133, 9.745699944792932001 ) ) ;
#31616=ORIENTED_EDGE ( 'NONE', *, *, #4584, .F. ) ;
#31627=CARTESIAN_POINT ( 'NONE',  ( -5.117438655294176186, -78.17837365130638716, -7.705456670207614600 ) ) ;
#31632=ORIENTED_EDGE ( 'NONE', *, *, #40495, .F. ) ;
#31633=CARTESIAN_POINT ( 'NONE',  ( -0.003049617359667225382, -77.47517976812264351, 9.249906914136946767 ) ) ;
#31634=CARTESIAN_POINT ( 'NONE',  ( 9.391860901740999523, -77.28449860050398001, 5.803232400709999794 ) ) ;
#31636=CARTESIAN_POINT ( 'NONE',  ( -9.139898499914998808, -77.30632546697400187, 2.826942883852999966 ) ) ;
#31641=CARTESIAN_POINT ( 'NONE',  ( 8.291742182491999458, -78.23574086744999079, 7.136865503491999441 ) ) ;
#31654=CARTESIAN_POINT ( 'NONE',  ( 4.625011536115999355, -80.27905154712398428, -10.42155147329000009 ) ) ;
#31665=CARTESIAN_POINT ( 'NONE',  ( 10.71369944335147828, -79.92916666666667425, -2.879226727952064913 ) ) ;
#31669=CARTESIAN_POINT ( 'NONE',  ( 0.000000000000000000, -80.99999999999998579, -5.499999999999927169 ) ) ;
#31682=CARTESIAN_POINT ( 'NONE',  ( -8.631379868284000167, -78.29701580198705813, 6.779623747091000574 ) ) ;
#31694=EDGE_LOOP ( 'NONE', ( #32624, #13170, #7705, #48142 ) ) ;
#31708=EDGE_CURVE ( 'NONE', #16896, #24330, #45761, .T. ) ;
#31710=CARTESIAN_POINT ( 'NONE',  ( -3.907230163516999699, -77.80156924675998198, -8.882807090995999744 ) ) ;
#31730=CARTESIAN_POINT ( 'NONE',  ( 8.405424692078989679, -77.20000000000001705, -6.846044140412126389 ) ) ;
#31741=ORIENTED_EDGE ( 'NONE', *, *, #39701, .T. ) ;
#31743=CYLINDRICAL_SURFACE ( 'NONE', #36131, 9.250000000000000000 ) ;
#31747=CARTESIAN_POINT ( 'NONE',  ( -4.670571261811000241, -78.93712829118099705, 8.172940633331000626 ) ) ;
#31772=ORIENTED_EDGE ( 'NONE', *, *, #52223, .T. ) ;
#31783=CARTESIAN_POINT ( 'NONE',  ( 6.545892007090739817, -78.78773550716071838, -6.535419499853671432 ) ) ;
#31806=CARTESIAN_POINT ( 'NONE',  ( -4.989874071371793285, -77.36354942115313804, 9.622404567693822131 ) ) ;
#31807=DIRECTION ( 'NONE',  ( 0.000000000000000000, -1.000000000000000000, 0.000000000000000000 ) ) ;
#31821=CARTESIAN_POINT ( 'NONE',  ( -9.662137344075999223, -78.31914363189699202, 1.225886475437000023 ) ) ;
#31825=CARTESIAN_POINT ( 'NONE',  ( 11.00000000000000355, -78.83958333333332291, -1.439896632895299566 ) ) ;
#31834=CARTESIAN_POINT ( 'NONE',  ( 2.277955858752000129, -78.13434347557100068, -10.97804107101999982 ) ) ;
#31839=CARTESIAN_POINT ( 'NONE',  ( -8.199999995296000321, -81.00000000470399186, -2.775962740116999943E-08 ) ) ;
#31840=CARTESIAN_POINT ( 'NONE',  ( -0.6514213267380000172, -79.71046273805198723, 9.745581310452999801 ) ) ;
#31853=CARTESIAN_POINT ( 'NONE',  ( 9.253844781852635037, -78.97679066890853505, -2.773644284455852649 ) ) ;
#31854=CARTESIAN_POINT ( 'NONE',  ( 8.176365817920217438, -79.88921606808585807, 4.324880645766660869 ) ) ;
#31865=EDGE_CURVE ( 'NONE', #1043, #53170, #29176, .T. ) ;
#31875=CARTESIAN_POINT ( 'NONE',  ( 6.737116832614598927, -76.94999999999998863, -6.739285137172449147 ) ) ;
#31878=CARTESIAN_POINT ( 'NONE',  ( 4.710185975415000392, -77.37260406872297835, -8.400437955132002088 ) ) ;
#31886=CARTESIAN_POINT ( 'NONE',  ( -1.297526016723000053, -78.54572183911899685, -10.89864408161000142 ) ) ;
#31900=CARTESIAN_POINT ( 'NONE',  ( -10.88870934378999955, -79.29337123098800078, 1.874540603341000145 ) ) ;
#31919=CARTESIAN_POINT ( 'NONE',  ( -6.514807376190594468, -78.16298481418483846, -6.566430754354078303 ) ) ;
#31925=CARTESIAN_POINT ( 'NONE',  ( 2.297844492628001500, -77.45516506021056102, 8.961078302872612866 ) ) ;
#31926=CARTESIAN_POINT ( 'NONE',  ( 6.574300740938999077, -77.54560925314699205, -8.869200617850999890 ) ) ;
#31928=CARTESIAN_POINT ( 'NONE',  ( 5.417083560473000325, -79.06258353067298117, -8.051455326762999576 ) ) ;
#31935=CARTESIAN_POINT ( 'NONE',  ( 8.838457456548999502, -78.62903382810698361, -6.447440276951000193 ) ) ;
#31948=CARTESIAN_POINT ( 'NONE',  ( 9.372653703366999878, -78.83658701837899230, 0.8742135494153999709 ) ) ;
#31954=FACE_OUTER_BOUND ( 'NONE', #50977, .T. ) ;
#31960=CARTESIAN_POINT ( 'NONE',  ( 9.611650271896843734, -79.90833333333331723, -5.539808784079876425 ) ) ;
#31980=ORIENTED_EDGE ( 'NONE', *, *, #40478, .F. ) ;
#31988=ORIENTED_EDGE ( 'NONE', *, *, #28484, .T. ) ;
#31999=VERTEX_POINT ( 'NONE', #53068 ) ;
#32005=CARTESIAN_POINT ( 'NONE',  ( -4.475245744599999576, -78.79640326627398395, -8.610626265545000990 ) ) ;
#32023=CARTESIAN_POINT ( 'NONE',  ( 8.437633008360455378, -77.19999999999998863, -6.805276374351061364 ) ) ;
#32025=CARTESIAN_POINT ( 'NONE',  ( 0.000000000000000000, -74.64999999999999147, 0.000000000000000000 ) ) ;
#32028=DIRECTION ( 'NONE',  ( 0.000000000000000000, 1.000000000000000000, 0.000000000000000000 ) ) ;
#32029=CARTESIAN_POINT ( 'NONE',  ( 0.000000000000000000, -74.64999999999999147, 0.000000000000000000 ) ) ;
#32035=CARTESIAN_POINT ( 'NONE',  ( -9.319163437353997992, -77.78947964090998823, -6.149666482694000180 ) ) ;
#32039=CARTESIAN_POINT ( 'NONE',  ( 8.881263526186000234, -77.73629938523899341, 3.434171575746000293 ) ) ;
#32051=CARTESIAN_POINT ( 'NONE',  ( 4.025753977166000475, -79.52580109776799588, -10.17256709246999868 ) ) ;
#32053=FACE_OUTER_BOUND ( 'NONE', #10895, .T. ) ;
#32058=VERTEX_POINT ( 'NONE', #3761 ) ;
#32062=CIRCLE ( 'NONE', #52844, 9.549999999999998934 ) ;
#32073=LINE ( 'NONE', #5511, #8976 ) ;
#32077=CARTESIAN_POINT ( 'NONE',  ( 0.003320946630736449148, -78.72517372709556582, -9.249912909581682996 ) ) ;
#32083=CARTESIAN_POINT ( 'NONE',  ( 1.210716439189422733, -77.73555344446525339, -9.249687892553014379 ) ) ;
#32092=CARTESIAN_POINT ( 'NONE',  ( 8.067746785342526650, -79.99999999999998579, 4.933239913214655381 ) ) ;
#32095=EDGE_CURVE ( 'NONE', #12885, #29148, #18811, .T. ) ;
#32102=DIRECTION ( 'NONE',  ( 0.000000000000000000, -1.000000000000000000, 0.000000000000000000 ) ) ;
#32114=FACE_OUTER_BOUND ( 'NONE', #50089, .T. ) ;
#32115=CARTESIAN_POINT ( 'NONE',  ( 11.00000000000000000, -78.94999999999998863, -1.064824513673000067E-14 ) ) ;
#32128=EDGE_CURVE ( 'NONE', #14347, #44860, #20194, .T. ) ;
#32131=CARTESIAN_POINT ( 'NONE',  ( 6.653382217586999658, -79.82567319065550748, 7.150748904218000135 ) ) ;
#32137=ORIENTED_EDGE ( 'NONE', *, *, #4076, .T. ) ;
#32144=CARTESIAN_POINT ( 'NONE',  ( 6.922407739197930177, -79.90780257099709161, 6.135667632505162672 ) ) ;
#32159=EDGE_CURVE ( 'NONE', #36426, #17327, #32073, .T. ) ;
#32161=CARTESIAN_POINT ( 'NONE',  ( 10.69999999999999929, -77.19999999999998863, 0.000000000000000000 ) ) ;
#32167=CARTESIAN_POINT ( 'NONE',  ( -6.715271092063999525, -77.77053767652898841, -6.903502308617000871 ) ) ;
#32175=AXIS2_PLACEMENT_3D ( 'NONE', #57560, #7686, #39839 ) ;
#32176=CARTESIAN_POINT ( 'NONE',  ( 10.87588596538000019, -79.72971893809699395, -1.476184626237000197 ) ) ;
#32188=CARTESIAN_POINT ( 'NONE',  ( 6.124581921013000141, -78.47869295534098910, -9.196052954390001588 ) ) ;
#32195=CARTESIAN_POINT ( 'NONE',  ( -10.90777360733681789, -78.95896512884534957, -1.219956472363630917 ) ) ;
#32203=ORIENTED_EDGE ( 'NONE', *, *, #568, .F. ) ;
#32215=CARTESIAN_POINT ( 'NONE',  ( 2.655231642783967949, -77.45200555099675910, 8.860774034763510443 ) ) ;
#32216=CARTESIAN_POINT ( 'NONE',  ( -1.776188306762000124, -77.54229276148697636, -10.89629776253999971 ) ) ;
#32219=CARTESIAN_POINT ( 'NONE',  ( 1.260641617779999946, -77.75508739074000175, 9.621927669549000584 ) ) ;
#32223=CARTESIAN_POINT ( 'NONE',  ( -10.49924843836999955, -80.51978164716398112, -4.054558598941000014 ) ) ;
#32224=CARTESIAN_POINT ( 'NONE',  ( -7.484260875330000395, -78.99423443443198778, -7.979577400219000083 ) ) ;
#32237=CARTESIAN_POINT ( 'NONE',  ( -7.608915353569000395, -77.52909087844598446, 5.542165790529000269 ) ) ;
#32243=LINE ( 'NONE', #19277, #32460 ) ;
#32246=CARTESIAN_POINT ( 'NONE',  ( 10.31626776183999894, -78.09212595279097968, -3.746764721243999841 ) ) ;
#32256=CARTESIAN_POINT ( 'NONE',  ( -1.331888048429999971, -78.29475676510899973, -11.18726993471000064 ) ) ;
#32272=ORIENTED_EDGE ( 'NONE', *, *, #23041, .T. ) ;
#32282=CARTESIAN_POINT ( 'NONE',  ( 5.202079365288874158, -78.27269934739146606, -7.648514488450266491 ) ) ;
#32289=CARTESIAN_POINT ( 'NONE',  ( -9.626984307556000431, -78.19950285456599204, 1.221426423741999834 ) ) ;
#32315=CIRCLE ( 'NONE', #14419, 4.100000000000000533 ) ;
#32319=EDGE_LOOP ( 'NONE', ( #15458, #48010, #20603, #23936, #35849 ) ) ;
#32322=EDGE_CURVE ( 'NONE', #50939, #2832, #45384, .T. ) ;
#32323=CARTESIAN_POINT ( 'NONE',  ( -0.9778317140632999394, -77.36108401092899101, -11.12245703213999981 ) ) ;
#32326=CARTESIAN_POINT ( 'NONE',  ( -3.790141024232000166, -78.11283724644100346, -8.616613344227999960 ) ) ;
#32340=DIRECTION ( 'NONE',  ( 1.000000000000000000, 0.000000000000000000, 0.000000000000000000 ) ) ;
#32344=ORIENTED_EDGE ( 'NONE', *, *, #43659, .T. ) ;
#32357=CARTESIAN_POINT ( 'NONE',  ( 9.690624391480906041, -78.59567732945993157, -0.5153898459522678888 ) ) ;
#32366=CARTESIAN_POINT ( 'NONE',  ( -1.608690456112285672, -78.71114049471292162, -9.109175791259589872 ) ) ;
#32370=CARTESIAN_POINT ( 'NONE',  ( -9.274707012308825327, -80.14539018384232349, -5.914949570800462908 ) ) ;
#32378=DIRECTION ( 'NONE',  ( 0.000000000000000000, 1.000000000000000000, 1.184237892934000027E-14 ) ) ;
#32380=CARTESIAN_POINT ( 'NONE',  ( 9.250000000000000000, -79.84999999999999432, 0.000000000000000000 ) ) ;
#32383=CARTESIAN_POINT ( 'NONE',  ( 10.36873448126860886, -78.11209359995925183, -2.835127193485178054 ) ) ;
#32387=DIRECTION ( 'NONE',  ( 0.000000000000000000, 0.000000000000000000, -1.000000000000000000 ) ) ;
#32414=CARTESIAN_POINT ( 'NONE',  ( 11.21715554180000041, -77.31778620838598215, 1.538714659179999833 ) ) ;
#32418=CARTESIAN_POINT ( 'NONE',  ( -8.396223008680999911, -79.93312895501298954, -4.990405176070999538 ) ) ;
#32433=ORIENTED_EDGE ( 'NONE', *, *, #51653, .T. ) ;
#32443=CARTESIAN_POINT ( 'NONE',  ( 10.55330385607999943, -78.39927573546698625, 3.944190366796999303 ) ) ;
#32449=CARTESIAN_POINT ( 'NONE',  ( -9.502046381818999521, -77.31279324197298308, 1.985581014958000212 ) ) ;
#32450=CARTESIAN_POINT ( 'NONE',  ( -9.497876546326999403, -77.25168256874098915, -0.2008509664869000122 ) ) ;
#32454=CARTESIAN_POINT ( 'NONE',  ( -2.166619587182999851, -77.59999470175499425, 9.383974079751000730 ) ) ;
#32460=VECTOR ( 'NONE', #9838, 1000.000000000000114 ) ;
#32463=CARTESIAN_POINT ( 'NONE',  ( 9.694840914897000062, -79.70162658376399634, -5.145296513660000848 ) ) ;
#32477=CIRCLE ( 'NONE', #18383, 1.000000000000000000 ) ;
#32483=CARTESIAN_POINT ( 'NONE',  ( 10.55673762599399090, -78.67804158551905402, -3.003849123923255426 ) ) ;
#32485=ORIENTED_EDGE ( 'NONE', *, *, #27096, .T. ) ;
#32502=CARTESIAN_POINT ( 'NONE',  ( 7.455184149750110123, -77.40051399983991587, 5.475553992661359004 ) ) ;
#32503=CARTESIAN_POINT ( 'NONE',  ( 10.65102452230999930, -77.64103837914298367, 2.905137941168000282 ) ) ;
#32504=VECTOR ( 'NONE', #6333, 1000.000000000000000 ) ;
#32511=CARTESIAN_POINT ( 'NONE',  ( 9.663556473158999793, -79.64035858408298907, -5.128693071642000056 ) ) ;
#32517=CARTESIAN_POINT ( 'NONE',  ( -10.89546045048518508, -77.19999999999998863, 1.402775879548545213 ) ) ;
#32521=CARTESIAN_POINT ( 'NONE',  ( 7.000000000000000000, -80.99999999999998579, -1.199999999999970424 ) ) ;
#32536=CARTESIAN_POINT ( 'NONE',  ( -10.57157196544999955, -79.79227723196800071, 2.324769239444999691 ) ) ;
#32537=CARTESIAN_POINT ( 'NONE',  ( 0.000000000000000000, -74.64999999999999147, 0.000000000000000000 ) ) ;
#32546=CARTESIAN_POINT ( 'NONE',  ( 11.23392183412000023, -78.43521853677198408, 0.8531908288953000685 ) ) ;
#32550=VECTOR ( 'NONE', #9368, 1000.000000000000000 ) ;
#32553=CARTESIAN_POINT ( 'NONE',  ( 0.000000000000000000, -81.19999999999998863, 7.000000000000000000 ) ) ;
#32554=DIRECTION ( 'NONE',  ( 0.000000000000000000, -1.000000000000000000, 0.000000000000000000 ) ) ;
#32566=VERTEX_POINT ( 'NONE', #31052 ) ;
#32572=CARTESIAN_POINT ( 'NONE',  ( 5.263805209930564111, -78.27334790553378241, -7.606318086626214559 ) ) ;
#32577=CARTESIAN_POINT ( 'NONE',  ( -8.801507186371804181, -77.57514545457918587, 2.845283712962050071 ) ) ;
#32580=CARTESIAN_POINT ( 'NONE',  ( 7.256139241522999939, -77.57763388114098291, 6.443535727668999513 ) ) ;
#32581=EDGE_CURVE ( 'NONE', #44860, #35917, #56136, .T. ) ;
#32585=B_SPLINE_SURFACE_WITH_KNOTS ( 'NONE', 3, 3, ( 
 ( #18980, #50570, #31948, #36972, #28396, #54985, #37261, #45564, #14821, #1859, #14241, #1562, #10125, #49993, #32819, #50865, #46741, #37552, #55569, #28103, #46153, #6261, #24276, #5677, #19854, #1277, #41116, #23688, #710, #33116, #9539, #41701, #37849, #51157, #13952, #10411, #9831, #36681, #23401, #27522, #19270, #10712, #46443, #54697, #28690, #5971, #5109, #23976, #32237, #50280, #27812, #45859, #5392, #2147, #42873, #3007, #7716, #25717, #52596, #28987, #38428, #20148, #21288, #38135, #33702, #33412, #30134 ),
 ( #16001, #48183, #43743, #52027, #3296, #43165, #6558, #2430, #24566, #25431, #51450, #56446, #55869, #16579, #15419, #34276, #51741, #42583, #6847, #11002, #33988, #11290, #56158, #43446, #11580, #29270, #47028, #47896, #34564, #20433, #15707, #21003, #39009, #24857, #47318, #29559, #47614, #57017, #7138, #12147, #25139, #2722, #20718, #52311, #56739, #7428, #11867, #29844, #26292, #35423, #39295, #58174, #22153, #49329, #53755, #49033, #13292, #16870, #30995, #39868, #4449, #36024, #26869, #22450, #9174, #27157, #44305 ),
 ( #45197, #3861, #34849, #52881, #44023, #3575, #39584, #57588, #21859, #17149, #57881, #53453, #26568, #4154, #44600, #36611, #23904, #19199, #37477, #18328, #18620, #36898, #33040, #45490, #15048, #1207, #10053, #46079, #638, #45788, #28318, #19484, #37190, #55204, #55498, #14747, #54634, #32746, #49922, #925, #10636, #23614, #51086, #28035, #32167, #14170, #13884, #41627, #9467, #41051, #32454, #54911, #40755, #18905, #5324, #50206, #14463, #50794, #31878, #9756, #27741, #50499, #27452, #28618, #5603, #10340, #23331 ),
 ( #46663, #22745, #46371, #5895, #5033, #23035, #41922, #41339, #1494, #349, #36321, #54344, #20642, #51672, #29483, #37776, #7066, #34486, #6482, #52232, #29199, #42220, #25067, #43091, #38927, #34195, #11789, #11219, #24784, #56944, #16503, #2360, #52516, #51952, #15347, #47244, #33341, #29764, #1785, #6775, #12072, #25350, #6190, #2649, #2078, #51374, #15634, #30053, #42799, #42507, #10931, #47820, #20358, #20076, #24203, #56662, #43367, #38353, #24494, #7351, #2925, #33630, #46956, #19781, #56375, #20926, #15925 ) ),
 .UNSPECIFIED., .F., .F., .F.,
 ( 4, 4 ),
 ( 4, 1, 1, 1, 1, 1, 1, 1, 1, 1, 1, 1, 1, 1, 1, 1, 1, 1, 1, 1, 1, 1, 1, 1, 1, 1, 1, 1, 1, 1, 1, 1, 1, 1, 1, 1, 1, 1, 1, 1, 1, 1, 1, 1, 1, 1, 1, 1, 1, 1, 1, 1, 1, 1, 1, 1, 1, 1, 1, 1, 1, 1, 1, 1, 4 ),
 ( -0.1387574078320999993, 1.138757407831999968 ),
 ( -0.02000000000000000042, -0.003749999999999999861, 0.01250000000000000069, 0.02875000000000000125, 0.04499999999999999833, 0.06124999999999999889, 0.07749999999999999944, 0.09375000000000000000, 0.1100000000000000006, 0.1262500000000000011, 0.1424999999999999878, 0.1587500000000000022, 0.1749999999999999889, 0.1912500000000000033, 0.2074999999999999900, 0.2237500000000000044, 0.2399999999999999911, 0.2562499999999999778, 0.2725000000000000200, 0.2887500000000000067, 0.3049999999999999933, 0.3212499999999999800, 0.3375000000000000222, 0.3537500000000000089, 0.3699999999999999956, 0.3862499999999999822, 0.4025000000000000244, 0.4187500000000000111, 0.4349999999999999978, 0.4512499999999999845, 0.4675000000000000266, 0.4837500000000000133, 0.5000000000000000000, 0.5162499999999999867, 0.5324999999999999734, 0.5487499999999999600, 0.5649999999999999467, 0.5812500000000000444, 0.5975000000000000311, 0.6137500000000000178, 0.6300000000000000044, 0.6462499999999999911, 0.6624999999999999778, 0.6787499999999999645, 0.6949999999999999512, 0.7112500000000000488, 0.7275000000000000355, 0.7437500000000000222, 0.7600000000000000089, 0.7762499999999999956, 0.7924999999999999822, 0.8087499999999999689, 0.8249999999999999556, 0.8412500000000000533, 0.8575000000000000400, 0.8737500000000000266, 0.8900000000000000133, 0.9062500000000000000, 0.9224999999999999867, 0.9387499999999999734, 0.9549999999999999600, 0.9712499999999999467, 0.9875000000000000444, 1.003749999999999920, 1.020000000000000018 ),
 .UNSPECIFIED. ) ;
#32596=ADVANCED_FACE ( 'NONE', ( #41978 ), #28610, .F. ) ;
#32601=CARTESIAN_POINT ( 'NONE',  ( 7.658490574713046506, -77.20000000000000284, -7.714358540288501764 ) ) ;
#32606=CARTESIAN_POINT ( 'NONE',  ( -1.439896632895333317, -79.08541666666666003, 10.99999999999999822 ) ) ;
#32607=CARTESIAN_POINT ( 'NONE',  ( -0.4864526504254000350, -79.20815779017299008, 9.739263145490999918 ) ) ;
#32612=CARTESIAN_POINT ( 'NONE',  ( 4.447146149678999905, -77.08500682716429253, 10.06768414028999992 ) ) ;
#32614=CARTESIAN_POINT ( 'NONE',  ( 0.000000000000000000, -76.19999999999998863, -10.50000000000000000 ) ) ;
#32615=CARTESIAN_POINT ( 'NONE',  ( -8.508571376020000798, -78.05598958818299593, -4.026835934908000070 ) ) ;
#32617=CARTESIAN_POINT ( 'NONE',  ( -2.302038976840258933, -80.20520833350919077, -10.81263029561343103 ) ) ;
#32624=ORIENTED_EDGE ( 'NONE', *, *, #1131, .T. ) ;
#32628=ORIENTED_EDGE ( 'NONE', *, *, #47114, .F. ) ;
#32642=ORIENTED_EDGE ( 'NONE', *, *, #45453, .T. ) ;
#32644=CARTESIAN_POINT ( 'NONE',  ( -2.572168127912981106, -78.45355818381494828, -9.357231370006124038 ) ) ;
#32647=EDGE_CURVE ( 'NONE', #54228, #34245, #21418, .T. ) ;
#32654=CARTESIAN_POINT ( 'NONE',  ( 7.541194259660339405, -78.80083539858046038, -5.358726617299357287 ) ) ;
#32658=CARTESIAN_POINT ( 'NONE',  ( -9.180191738191043171, -80.14658889808482911, -6.059864792341575601 ) ) ;
#32674=CARTESIAN_POINT ( 'NONE',  ( 9.388046065757025715, -77.24119165340866289, 5.283002242768499279 ) ) ;
#32677=CARTESIAN_POINT ( 'NONE',  ( -9.438868967565998247, -79.39261762096144537, -5.601050722391000214 ) ) ;
#32686=CARTESIAN_POINT ( 'NONE',  ( 9.188646138531803231, -78.34088890680163786, -1.063366993189087228 ) ) ;
#32689=CARTESIAN_POINT ( 'NONE',  ( 9.499178638196321245, -79.00092112126561972, 0.1004274591880019996 ) ) ;
#32690=CARTESIAN_POINT ( 'NONE',  ( 8.270224399031000928, -78.03490534060698280, -5.144228231339999624 ) ) ;
#32703=ORIENTED_EDGE ( 'NONE', *, *, #41128, .T. ) ;
#32709=CARTESIAN_POINT ( 'NONE',  ( 8.193575559979001000, -79.18625781507998340, 5.316613930189999948 ) ) ;
#32713=EDGE_LOOP ( 'NONE', ( #3747, #40178, #56409, #1385 ) ) ;
#32720=CARTESIAN_POINT ( 'NONE',  ( 8.131718752285998164, -76.87468074736040080, -4.888939325748999920 ) ) ;
#32727=AXIS2_PLACEMENT_3D ( 'NONE', #32553, #18713, #1590 ) ;
#32741=CARTESIAN_POINT ( 'NONE',  ( 9.242241171838999847, -77.10391830622759812, 2.968601151647999536 ) ) ;
#32746=CARTESIAN_POINT ( 'NONE',  ( 9.511010664898998712, -77.96950448043199344, 1.514558053418999961 ) ) ;
#32747=EDGE_CURVE ( 'NONE', #29062, #1603, #1065, .T. ) ;
#32753=EDGE_CURVE ( 'NONE', #49740, #18403, #43287, .T. ) ;
#32756=CARTESIAN_POINT ( 'NONE',  ( 5.330173052271000245, -78.32510122146300091, 9.594439332582000546 ) ) ;
#32758=CARTESIAN_POINT ( 'NONE',  ( -0.09698300086874001025, -79.76726403785698949, -9.669821086516000364 ) ) ;
#32774=CIRCLE ( 'NONE', #8256, 4.299999999999999822 ) ;
#32775=CARTESIAN_POINT ( 'NONE',  ( -7.396918292183192634, -79.94791666666667140, 5.684557159767932077 ) ) ;
#32776=CARTESIAN_POINT ( 'NONE',  ( 10.99999999999999645, -79.45864668888548010, 1.195232468347081189 ) ) ;
#32792=EDGE_LOOP ( 'NONE', ( #30209, #44458, #37807, #49141 ) ) ;
#32793=CARTESIAN_POINT ( 'NONE',  ( 9.162130905092393363, -77.36116891436404330, 1.277012193982459687 ) ) ;
#32802=CARTESIAN_POINT ( 'NONE',  ( 7.763360352781000451, -78.74140324543799352, 7.708310604078000061 ) ) ;
#32810=CARTESIAN_POINT ( 'NONE',  ( -10.99598848309850574, -77.19999999999996021, 0.3327073738962888494 ) ) ;
#32819=CARTESIAN_POINT ( 'NONE',  ( -4.670571261811000241, -78.49550106883198453, 8.172940633331000626 ) ) ;
#32830=CARTESIAN_POINT ( 'NONE',  ( -10.69701368780000017, -79.80164135007898096, 1.066019776055000090 ) ) ;
#32833=LINE ( 'NONE', #45578, #661 ) ;
#32838=CARTESIAN_POINT ( 'NONE',  ( 5.471330588277999674, -78.01383322178197943, 9.848526282906998830 ) ) ;
#32844=CARTESIAN_POINT ( 'NONE',  ( 10.69999999999999929, -80.49999999999998579, 0.000000000000000000 ) ) ;
#32864=CARTESIAN_POINT ( 'NONE',  ( 1.818239999436394250, -78.24087318384329137, -9.069458920223979703 ) ) ;
#32869=CARTESIAN_POINT ( 'NONE',  ( -7.805592913195344096, -77.55492559948099540, 4.964263552560149506 ) ) ;
#32874=CARTESIAN_POINT ( 'NONE',  ( 9.131029190779001325, -77.49236239375397872, -3.285576857342999979 ) ) ;
#32888=CARTESIAN_POINT ( 'NONE',  ( 0.000000000000000000, -78.49999999999998579, 0.000000000000000000 ) ) ;
#32896=CARTESIAN_POINT ( 'NONE',  ( 11.06159046600000018, -78.35992084691199011, -1.510225926472999802 ) ) ;
#32897=CARTESIAN_POINT ( 'NONE',  ( 8.796335266379989193, -79.00208333333331723, 6.760013919724051412 ) ) ;
#32900=CARTESIAN_POINT ( 'NONE',  ( 4.903292266777000030, -79.99716956313798732, -8.177287202055998350 ) ) ;
#32906=CARTESIAN_POINT ( 'NONE',  ( -10.62852719317000094, -77.21828546760299616, 3.420469065344999837 ) ) ;
#32914=CARTESIAN_POINT ( 'NONE',  ( 9.499157866768639380, -79.10080562451891240, 0.1004279358040388037 ) ) ;
#32937=VERTEX_POINT ( 'NONE', #1829 ) ;
#32939=CARTESIAN_POINT ( 'NONE',  ( 6.240635229950907359, -78.16931989252493906, 7.431574511284630979 ) ) ;
#32945=CARTESIAN_POINT ( 'NONE',  ( 1.487026788147999934, -77.38724284451876656, -9.589549613196998834 ) ) ;
#32949=CARTESIAN_POINT ( 'NONE',  ( -6.370113089561758812, -78.66462273621775125, -6.707093103444599969 ) ) ;
#32954=CARTESIAN_POINT ( 'NONE',  ( -5.652729497046634854, -80.18219462805302555, -9.436345438157960785 ) ) ;
#32962=DIRECTION ( 'NONE',  ( 0.000000000000000000, -1.000000000000000000, 0.000000000000000000 ) ) ;
#32972=CARTESIAN_POINT ( 'NONE',  ( -10.81678667190517906, -77.45531774696169691, -0.6574978399008775121 ) ) ;
#32978=CARTESIAN_POINT ( 'NONE',  ( 9.192561553568495469, -78.34118095183893615, -1.028967211150572547 ) ) ;
#32981=CARTESIAN_POINT ( 'NONE',  ( 0.000000000000000000, -81.99999999999998579, 0.000000000000000000 ) ) ;
#32982=CARTESIAN_POINT ( 'NONE',  ( -9.704555048820999730, -77.83593853670399199, -0.8254132364208000006 ) ) ;
#32994=CARTESIAN_POINT ( 'NONE',  ( -8.959657150203256037, -77.52237568801258760, -2.594892310216006859 ) ) ;
#32998=CARTESIAN_POINT ( 'NONE',  ( -1.559871468835000163, -77.23492311450797843, -11.32549190513999982 ) ) ;
#33004=CARTESIAN_POINT ( 'NONE',  ( 3.269429986698999979, -79.73829300546499610, 9.203886808668999109 ) ) ;
#33007=CARTESIAN_POINT ( 'NONE',  ( -4.799999999787999627, -74.99999999978798826, -2.226280155659000170E-09 ) ) ;
#33008=CIRCLE ( 'NONE', #45307, 4.100000000000000533 ) ;
#33018=B_SPLINE_CURVE_WITH_KNOTS ( 'NONE', 3,
 ( #51760, #24589, #34871, #20740, #57327, #11887, #39317, #29865, #12168, #16890, #6577, #43763, #47919, #20167, #30154, #29578, #38739, #47339 ),
 .UNSPECIFIED., .F., .F.,
 ( 4, 2, 2, 2, 2, 2, 2, 2, 4 ),
 ( 0.000000000000000000, 0.1250000000000000278, 0.2500000000000000000, 0.3750000000000001110, 0.5000000000000001110, 0.6250000000000001110, 0.7500000000000002220, 0.8750000000000001110, 1.000000000000000000 ),
 .UNSPECIFIED. ) ;
#33025=CARTESIAN_POINT ( 'NONE',  ( 0.000000000000000000, -80.35000000001998899, 0.000000000000000000 ) ) ;
#33040=CARTESIAN_POINT ( 'NONE',  ( 6.930806504809000401, -78.39586191736599119, -6.687086896242999678 ) ) ;
#33042=CARTESIAN_POINT ( 'NONE',  ( 7.545211986414574135, -77.01380208334457222, 5.799587084941282278 ) ) ;
#33051=CARTESIAN_POINT ( 'NONE',  ( 7.218984044805000444, -79.30833362310698931, 8.267423174273998754 ) ) ;
#33052=CARTESIAN_POINT ( 'NONE',  ( -10.81039872835957816, -80.08464542082350590, 2.129203739267044426 ) ) ;
#33053=CARTESIAN_POINT ( 'NONE',  ( 9.559470275639000647, -79.32991171449499745, 0.08713422356856999340 ) ) ;
#33055=DIRECTION ( 'NONE',  ( 0.7071067811865470176, -0.7071067811865470176, 3.680441518142245308E-08 ) ) ;
#33071=CARTESIAN_POINT ( 'NONE',  ( -1.297546493877329565, -78.56567216818805832, -10.89881608063975804 ) ) ;
#33092=CARTESIAN_POINT ( 'NONE',  ( 7.482597622593881503, -77.40011871758873951, 5.438000268058704734 ) ) ;
#33093=CARTESIAN_POINT ( 'NONE',  ( -10.84202097104999929, -77.47535685249599169, 2.082001701158999740 ) ) ;
#33100=CARTESIAN_POINT ( 'NONE',  ( 8.267239500339000458, -78.18724719090198505, -6.983083964283999912 ) ) ;
#33105=CARTESIAN_POINT ( 'NONE',  ( -10.39360022642970804, -77.19999999999998863, 3.478205997298121854 ) ) ;
#33116=CARTESIAN_POINT ( 'NONE',  ( -9.338489578732000140, -78.06914363189699202, 1.184823571421999899 ) ) ;
#33127=CARTESIAN_POINT ( 'NONE',  ( -3.673218652927999539, -79.21170190909299436, 10.34270183798999909 ) ) ;
#33139=DIRECTION ( 'NONE',  ( 1.000000000000000000, 0.000000000000000000, 0.000000000000000000 ) ) ;
#33153=DIRECTION ( 'NONE',  ( 0.000000000000000000, 1.000000000000000000, 0.000000000000000000 ) ) ;
#33157=CYLINDRICAL_SURFACE ( 'NONE', #21617, 9.250000000000000000 ) ;
#33160=CARTESIAN_POINT ( 'NONE',  ( 6.321504634335313177, -78.28489978996086052, -6.754501521448134760 ) ) ;
#33169=CARTESIAN_POINT ( 'NONE',  ( 4.746041175454999816, -77.43551473549599962, -8.464384343845999581 ) ) ;
#33170=DIRECTION ( 'NONE',  ( 0.000000000000000000, 1.000000000000000000, 0.000000000000000000 ) ) ;
#33178=CARTESIAN_POINT ( 'NONE',  ( -10.77593383617251277, -80.24166666668229198, -2.296997422106781706 ) ) ;
#33183=CARTESIAN_POINT ( 'NONE',  ( -9.248871138250700952, -79.58998423164975122, 1.210936878181855691 ) ) ;
#33184=CARTESIAN_POINT ( 'NONE',  ( 0.000000000000000000, -80.49999999999998579, 0.000000000000000000 ) ) ;
#33187=CARTESIAN_POINT ( 'NONE',  ( -9.611650271896834852, -78.24166666666666003, -5.539808784079895965 ) ) ;
#33190=CARTESIAN_POINT ( 'NONE',  ( -4.628649168153988747, -77.18975860091060781, -8.076984658556984442 ) ) ;
#33191=CARTESIAN_POINT ( 'NONE',  ( -3.507257632973999950, -79.86191712038298363, 8.865074537405000399 ) ) ;
#33192=AXIS2_PLACEMENT_3D ( 'NONE', #27580, #33170, #1332 ) ;
#33199=CARTESIAN_POINT ( 'NONE',  ( 11.17006500217999942, -77.44000681347299064, 1.528262659639999965 ) ) ;
#33222=VERTEX_POINT ( 'NONE', #29527 ) ;
#33224=ORIENTED_EDGE ( 'NONE', *, *, #54901, .F. ) ;
#33233=CARTESIAN_POINT ( 'NONE',  ( -1.210723843908615871, -79.21478203666787010, -9.248604757515597186 ) ) ;
#33239=CARTESIAN_POINT ( 'NONE',  ( 6.240531904507999883, -78.06941474361464373, 7.431451467605000083 ) ) ;
#33244=CARTESIAN_POINT ( 'NONE',  ( -6.733423791686919735, -78.66015289143886946, -6.348039707728767134 ) ) ;
#33252=DIRECTION ( 'NONE',  ( 0.000000000000000000, 0.7071067811866525998, -0.7071067811864425456 ) ) ;
#33258=CARTESIAN_POINT ( 'NONE',  ( 4.907702572637520078, -79.99999999999997158, 7.984394256099379916 ) ) ;
#33266=ADVANCED_FACE ( 'NONE', ( #33673 ), #52276, .F. ) ;
#33267=CARTESIAN_POINT ( 'NONE',  ( 5.663577320046584873, -77.78160512761387224, 9.213540343163701962 ) ) ;
#33268=CARTESIAN_POINT ( 'NONE',  ( 9.981840466370998755, -78.63412405397946259, 4.563647388395000171 ) ) ;
#33273=CARTESIAN_POINT ( 'NONE',  ( 8.342888411232321388, -78.31448426059630208, -3.994830225491370790 ) ) ;
#33278=CARTESIAN_POINT ( 'NONE',  ( 2.878019135186999922, -77.97805768234898949, -9.304660206797001010 ) ) ;
#33281=CARTESIAN_POINT ( 'NONE',  ( 1.437851432728850520, -80.22213541715329654, -10.97786456746221084 ) ) ;
#33289=CARTESIAN_POINT ( 'NONE',  ( -3.697742159549999741, -79.20909416798998848, 10.41175280961999938 ) ) ;
#33292=CARTESIAN_POINT ( 'NONE',  ( 10.80657406421999944, -79.95794665545098212, 4.085057409123999506 ) ) ;
#33296=CARTESIAN_POINT ( 'NONE',  ( 10.89779338388999896, -77.89524787048398480, 3.455448588212000072 ) ) ;
#33303=CARTESIAN_POINT ( 'NONE',  ( -5.726462542197000793, -80.08545445672149299, -7.912542777261000637 ) ) ;
#33304=ORIENTED_EDGE ( 'NONE', *, *, #7844, .F. ) ;
#33306=ADVANCED_FACE ( 'NONE', ( #2969 ), #34528, .F. ) ;
#33334=CARTESIAN_POINT ( 'NONE',  ( 2.613075649634000186, -77.24612214791498843, 9.236390685206998796 ) ) ;
#33335=DIRECTION ( 'NONE',  ( 0.000000000000000000, -1.000000000000000000, 0.000000000000000000 ) ) ;
#33341=CARTESIAN_POINT ( 'NONE',  ( 8.475813183550998886, -78.06180405034399428, 4.797946079729999092 ) ) ;
#33343=CARTESIAN_POINT ( 'NONE',  ( 8.250583882568891525, -77.00729166667787240, 4.756314485391412994 ) ) ;
#33354=CARTESIAN_POINT ( 'NONE',  ( 8.584472847271999996, -79.43113511353598710, 4.452153601206999767 ) ) ;
#33357=ORIENTED_EDGE ( 'NONE', *, *, #50535, .F. ) ;
#33367=PRODUCT_DEFINITION_SHAPE ( 'NONE', 'NONE',  #518 ) ;
#33370=CARTESIAN_POINT ( 'NONE',  ( -10.79343819383525016, -79.46462750683407705, -1.992363124314718181 ) ) ;
#33383=CARTESIAN_POINT ( 'NONE',  ( 0.000000000000000000, -74.64999999999999147, 0.000000000000000000 ) ) ;
#33386=VERTEX_POINT ( 'NONE', #31254 ) ;
#33388=ORIENTED_EDGE ( 'NONE', *, *, #26459, .T. ) ;
#33389=CARTESIAN_POINT ( 'NONE',  ( 7.465779029155634738, -77.40036112842625471, 5.461091003694943602 ) ) ;
#33397=CARTESIAN_POINT ( 'NONE',  ( 4.065750953757999220, -79.64804961620099277, -10.27363435345999854 ) ) ;
#33412=CARTESIAN_POINT ( 'NONE',  ( -8.866000417715000026, -77.05536039296339368, 2.742227037787000388 ) ) ;
#33424=CARTESIAN_POINT ( 'NONE',  ( 6.083963560182000130, -78.48130069644298601, -9.135064530700001129 ) ) ;
#33431=FACE_OUTER_BOUND ( 'NONE', #34948, .T. ) ;
#33436=CARTESIAN_POINT ( 'NONE',  ( 10.55330385607999943, -77.95764851311697896, 3.944190366796999303 ) ) ;
#33438=CARTESIAN_POINT ( 'NONE',  ( -11.00000000000000000, -79.69999999999998863, 0.000000000000000000 ) ) ;
#33452=CARTESIAN_POINT ( 'NONE',  ( 9.499693205731109202, -80.00008708754018016, -1.997583897032410100E-06 ) ) ;
#33459=CARTESIAN_POINT ( 'NONE',  ( 4.687722617765969879, -78.26731946421421071, -7.992545327129488619 ) ) ;
#33463=CARTESIAN_POINT ( 'NONE',  ( -9.250000000000000000, -77.59999999999999432, 0.000000000000000000 ) ) ;
#33467=CARTESIAN_POINT ( 'NONE',  ( -9.446433787353997857, -78.28822960936498987, -2.221620594898999990 ) ) ;
#33481=CARTESIAN_POINT ( 'NONE',  ( 0.000000000000000000, -81.79999999999998295, -10.70000000000298179 ) ) ;
#33485=CARTESIAN_POINT ( 'NONE',  ( -5.539808784079887083, -78.28333333333333144, -9.611650271896841957 ) ) ;
#33493=CARTESIAN_POINT ( 'NONE',  ( 9.314328882329000692, -79.06204449888298313, -2.038033000261999739 ) ) ;
#33497=CIRCLE ( 'NONE', #24062, 10.69999999999999929 ) ;
#33500=CARTESIAN_POINT ( 'NONE',  ( -4.728196578006000017, -77.46027578382999934, -9.874152122658001574 ) ) ;
#33504=CARTESIAN_POINT ( 'NONE',  ( -9.066428667704000688, -77.99914192992498840, 2.532008238717000204 ) ) ;
#33507=DIRECTION ( 'NONE',  ( -1.000000000000000000, 0.000000000000000000, 0.000000000000000000 ) ) ;
#33513=ORIENTED_EDGE ( 'NONE', *, *, #55235, .T. ) ;
#33535=CYLINDRICAL_SURFACE ( 'NONE', #27425, 10.69999999999999929 ) ;
#33537=CARTESIAN_POINT ( 'NONE',  ( 9.690463944985998168, -78.49577218054876937, -0.5153813127049999832 ) ) ;
#33539=CARTESIAN_POINT ( 'NONE',  ( -1.876049203459514203, -79.95935840993698207, -9.533404770284985119 ) ) ;
#33540=CARTESIAN_POINT ( 'NONE',  ( 5.212769757709797780, -77.02020172621061533, -8.147222165250761705 ) ) ;
#33542=CARTESIAN_POINT ( 'NONE',  ( -7.252642920492362144, -78.65334380994336527, -5.741174788834818798 ) ) ;
#33545=CARTESIAN_POINT ( 'NONE',  ( -7.720906625823901415, -80.16344810211410277, -7.835007712627920284 ) ) ;
#33558=EDGE_CURVE ( 'NONE', #409, #31439, #34688, .T. ) ;
#33561=CARTESIAN_POINT ( 'NONE',  ( 8.660058625535635102, -77.64905087922392113, -6.518498288151249653 ) ) ;
#33562=CARTESIAN_POINT ( 'NONE',  ( 8.140362823347702559, -78.29063355552166570, -7.514683589434230093 ) ) ;
#33563=CARTESIAN_POINT ( 'NONE',  ( -3.548303639236000340, -79.44880232962658795, -10.38621961377000247 ) ) ;
#33565=ORIENTED_EDGE ( 'NONE', *, *, #49269, .T. ) ;
#33570=CARTESIAN_POINT ( 'NONE',  ( 8.916672120480782837, -78.32869008935927013, -2.465681892806660169 ) ) ;
#33574=CARTESIAN_POINT ( 'NONE',  ( -6.496683922195000349, -78.26229597363898449, 7.256224481198000120 ) ) ;
#33582=ORIENTED_EDGE ( 'NONE', *, *, #22117, .F. ) ;
#33587=VECTOR ( 'NONE', #23251, 1000.000000000000000 ) ;
#33590=CARTESIAN_POINT ( 'NONE',  ( 5.551777116439001070, -77.39115562571699058, 9.867624315061000573 ) ) ;
#33593=ORIENTED_EDGE ( 'NONE', *, *, #55900, .F. ) ;
#33596=CARTESIAN_POINT ( 'NONE',  ( 1.739862777674999972, -79.49090881849700452, 9.611119481339999382 ) ) ;
#33603=EDGE_CURVE ( 'NONE', #20388, #11813, #28677, .T. ) ;
#33607=CARTESIAN_POINT ( 'NONE',  ( 2.887802510467000427, -76.96689670991779053, 9.218216609984001053 ) ) ;
#33609=CARTESIAN_POINT ( 'NONE',  ( -6.760013919724058518, -79.67291666666666572, -8.796335266379987416 ) ) ;
#33623=EDGE_CURVE ( 'NONE', #24388, #51092, #40341, .T. ) ;
#33624=CARTESIAN_POINT ( 'NONE',  ( 7.587587806099000076, -77.02559020532309830, -6.054761558390000076 ) ) ;
#33630=CARTESIAN_POINT ( 'NONE',  ( -5.177883096403999907, -77.35120832211899256, -8.249196342081999589 ) ) ;
#33637=CARTESIAN_POINT ( 'NONE',  ( -4.658421459997613923, -78.01682404241935842, 8.082575534271919437 ) ) ;
#33642=CARTESIAN_POINT ( 'NONE',  ( -10.99162204853783109, -80.09707396476217411, 0.4707213547353387151 ) ) ;
#33643=FACE_OUTER_BOUND ( 'NONE', #35019, .T. ) ;
#33649=CARTESIAN_POINT ( 'NONE',  ( 1.199999999999999956, -80.99999999999998579, -7.000000000000000000 ) ) ;
#33659=FACE_OUTER_BOUND ( 'NONE', #25825, .T. ) ;
#33673=FACE_OUTER_BOUND ( 'NONE', #46564, .T. ) ;
#33679=CARTESIAN_POINT ( 'NONE',  ( 7.482987909259383841, -77.40011310578455550, 5.437463058363716684 ) ) ;
#33680=CARTESIAN_POINT ( 'NONE',  ( 1.160587285869999929, -77.85707335648099559, 10.97894289003999901 ) ) ;
#33688=CARTESIAN_POINT ( 'NONE',  ( -1.306188688584000168, -78.60863250589198969, -10.97140668998000024 ) ) ;
#33702=CARTESIAN_POINT ( 'NONE',  ( -9.395661821092000210, -77.07430961238269163, 0.5765637145115000139 ) ) ;
#33714=CARTESIAN_POINT ( 'NONE',  ( 4.038786804788999873, -79.52483602375698979, -10.20549938643999965 ) ) ;
#33715=AXIS2_PLACEMENT_3D ( 'NONE', #36175, #54192, #31131 ) ;
#33723=CARTESIAN_POINT ( 'NONE',  ( -7.000000000000000000, -80.99999999999998579, 0.000000000000000000 ) ) ;
#33725=CARTESIAN_POINT ( 'NONE',  ( -9.009247259181924150, -78.02083333333332860, -2.421167930323337991 ) ) ;
#33726=CARTESIAN_POINT ( 'NONE',  ( 10.24618685648000138, -78.46331089110499590, 4.684505231889000143 ) ) ;
#33742=CARTESIAN_POINT ( 'NONE',  ( 3.089230661516983556, -79.90117923447624548, -9.040938033382255767 ) ) ;
#33747=ADVANCED_FACE ( 'NONE', ( #27579 ), #16406, .F. ) ;
#33752=CARTESIAN_POINT ( 'NONE',  ( -8.796452690798227891, -77.57500652429015986, 2.860862753174310491 ) ) ;
#33755=CARTESIAN_POINT ( 'NONE',  ( 9.512131559252001267, -78.00399131807598962, -1.920953556448999899 ) ) ;
#33770=CARTESIAN_POINT ( 'NONE',  ( 5.442928436726999664, -80.32760589224999137, 9.767578386100000287 ) ) ;
#33778=CARTESIAN_POINT ( 'NONE',  ( -0.09167600787266001749, -79.76881872134099183, 9.642089308184999652 ) ) ;
#33779=CARTESIAN_POINT ( 'NONE',  ( 2.600000000000000089, -77.49999999999998579, 0.000000000000000000 ) ) ;
#33786=CARTESIAN_POINT ( 'NONE',  ( 10.75070227408000001, -78.04375343946199450, -1.791407170491000178 ) ) ;
#33798=EDGE_CURVE ( 'NONE', #57837, #5962, #47007, .T. ) ;
#33801=CARTESIAN_POINT ( 'NONE',  ( 0.000000000000000000, -75.19999999999998863, 0.000000000000000000 ) ) ;
#33815=VERTEX_POINT ( 'NONE', #13570 ) ;
#33820=AXIS2_PLACEMENT_3D ( 'NONE', #43432, #3847, #57293 ) ;
#33825=CARTESIAN_POINT ( 'NONE',  ( 9.208765611215513402, -77.12463919408332913, 2.957848825889281219 ) ) ;
#33828=CARTESIAN_POINT ( 'NONE',  ( -3.523190925713206578, -78.69400124385185791, -8.552690850126060340 ) ) ;
#33831=CARTESIAN_POINT ( 'NONE',  ( -10.87293685240500984, -80.11224519801238841, -1.667451285520860305 ) ) ;
#33847=CARTESIAN_POINT ( 'NONE',  ( -9.745349999783975647, -77.98553474052145873, -4.591900818727150835 ) ) ;
#33849=CARTESIAN_POINT ( 'NONE',  ( 6.083963560182001018, -78.52175463664858057, -9.135064530700001129 ) ) ;
#33856=CARTESIAN_POINT ( 'NONE',  ( 7.282635111839001141, -77.63697173280098696, 6.467064367534000269 ) ) ;
#33862=DIRECTION ( 'NONE',  ( 0.000000000000000000, 1.000000000000000000, 0.000000000000000000 ) ) ;
#33866=CARTESIAN_POINT ( 'NONE',  ( 8.926269970182000080, -78.50678530967299196, -6.511497375149000177 ) ) ;
#33870=CARTESIAN_POINT ( 'NONE',  ( -10.99954758021000067, -77.53789446037799848, 2.683689935402000071 ) ) ;
#33874=CIRCLE ( 'NONE', #27260, 1.000000000000000000 ) ;
#33878=CARTESIAN_POINT ( 'NONE',  ( 3.366547962069000199, -79.78316274281900178, -9.168809063548000182 ) ) ;
#33889=CARTESIAN_POINT ( 'NONE',  ( -8.912837724143001239, -77.08455291172688817, 3.724768546731999752 ) ) ;
#33890=EDGE_CURVE ( 'NONE', #42976, #35609, #27369, .T. ) ;
#33895=CARTESIAN_POINT ( 'NONE',  ( -9.250000000000000000, -77.99999999999998579, 0.000000000000000000 ) ) ;
#33918=ORIENTED_EDGE ( 'NONE', *, *, #54164, .T. ) ;
#33920=CARTESIAN_POINT ( 'NONE',  ( 9.438973017186889081, -79.48883391750764815, -1.335242394275343081 ) ) ;
#33925=CARTESIAN_POINT ( 'NONE',  ( 1.480558193255000043, -79.50583043005198647, 9.556295997439999468 ) ) ;
#33927=CARTESIAN_POINT ( 'NONE',  ( -2.879226727952072018, -78.70416666666666572, -10.71369944335147295 ) ) ;
#33936=B_SPLINE_CURVE_WITH_KNOTS ( 'NONE', 3,
 ( #16348, #34328, #52363, #25479 ),
 .UNSPECIFIED., .F., .F.,
 ( 4, 4 ),
 ( 0.000000000000000000, 1.000000000000000000 ),
 .UNSPECIFIED. ) ;
#33938=DIRECTION ( 'NONE',  ( 1.000000000000000000, 0.000000000000000000, 0.000000000000000000 ) ) ;
#33944=CARTESIAN_POINT ( 'NONE',  ( 8.944729675425000082, -79.49243891193700051, 3.923329690209000908 ) ) ;
#33953=CARTESIAN_POINT ( 'NONE',  ( -9.157651701204139627, -78.82306796249194747, 3.211112441314760257 ) ) ;
#33964=ORIENTED_EDGE ( 'NONE', *, *, #2345, .T. ) ;
#33965=CARTESIAN_POINT ( 'NONE',  ( 5.783621287653671672, -77.27891537691782275, -7.219593957272368634 ) ) ;
#33974=CARTESIAN_POINT ( 'NONE',  ( 10.94849663375999960, -79.73232667919899086, -1.486040076422999956 ) ) ;
#33988=CARTESIAN_POINT ( 'NONE',  ( 9.508660861234000450, -78.38883383484099454, -0.5057122284909000287 ) ) ;
#34001=CARTESIAN_POINT ( 'NONE',  ( 10.85730540529999999, -79.13154306309999697, 1.607151491820999922 ) ) ;
#34007=EDGE_CURVE ( 'NONE', #32937, #13151, #3028, .T. ) ;
#34010=CARTESIAN_POINT ( 'NONE',  ( -8.082524092276891281, -78.04166666666668561, -4.658475568430815450 ) ) ;
#34012=CARTESIAN_POINT ( 'NONE',  ( 9.550909342165001092, -78.88469620609498634, -5.975706243058000133 ) ) ;
#34022=VERTEX_POINT ( 'NONE', #32161 ) ;
#34031=CARTESIAN_POINT ( 'NONE',  ( 2.365362167656198888, -79.35465741588306798, 9.023513813972275699 ) ) ;
#34035=CARTESIAN_POINT ( 'NONE',  ( -5.567379522523680180, -77.52644555432438267, 7.387118996003618321 ) ) ;
#34040=CARTESIAN_POINT ( 'NONE',  ( -7.707166124622999881, -77.32181941897998456, -5.896629607976000109 ) ) ;
#34044=FACE_OUTER_BOUND ( 'NONE', #7947, .T. ) ;
#34055=CARTESIAN_POINT ( 'NONE',  ( 9.015520653554002450, -80.22846898612900191, 6.426785087202000035 ) ) ;
#34060=ORIENTED_EDGE ( 'NONE', *, *, #14479, .T. ) ;
#34065=CARTESIAN_POINT ( 'NONE',  ( -7.482909773998999370, -79.44736948050399405, -6.081476139641999623 ) ) ;
#34066=LINE ( 'NONE', #33779, #21520 ) ;
#34067=CARTESIAN_POINT ( 'NONE',  ( -6.863219652448105279, -79.28723744505849425, 6.877600145842833967 ) ) ;
#34074=CARTESIAN_POINT ( 'NONE',  ( 0.9750215749860999814, -78.00291024847199139, -10.90431470505999911 ) ) ;
#34079=CARTESIAN_POINT ( 'NONE',  ( 5.212684961665999595, -76.94014298669428342, -8.147089634514999901 ) ) ;
#34085=VECTOR ( 'NONE', #54802, 1000.000000000000000 ) ;
#34104=DIRECTION ( 'NONE',  ( -1.000000000000000000, 0.000000000000000000, 0.000000000000000000 ) ) ;
#34110=CARTESIAN_POINT ( 'NONE',  ( -6.269511089439802731, -78.66582854956671156, -6.801662962640114607 ) ) ;
#34129=CARTESIAN_POINT ( 'NONE',  ( -0.9755963328057704054, -77.83258753084055570, 10.79518899496484430 ) ) ;
#34142=CARTESIAN_POINT ( 'NONE',  ( -9.375068251199000002, -78.41144320180897864, -2.204836785425999590 ) ) ;
#34150=ORIENTED_EDGE ( 'NONE', *, *, #55315, .F. ) ;
#34151=CARTESIAN_POINT ( 'NONE',  ( -2.919153588227000107, -78.76730753078498992, 10.54354582977000021 ) ) ;
#34157=CARTESIAN_POINT ( 'NONE',  ( 10.92669092472000081, -78.30827334234999171, 0.1833893325657000029 ) ) ;
#34164=CARTESIAN_POINT ( 'NONE',  ( 9.202039358297998461, -80.40014324972001702, 2.360608321670000453 ) ) ;
#34172=CARTESIAN_POINT ( 'NONE',  ( 11.00000000000000000, -77.94999999999998863, 0.000000000000000000 ) ) ;
#34186=CARTESIAN_POINT ( 'NONE',  ( -9.549999999953000085, -76.40000000004698677, 5.125988344190999543E-10 ) ) ;
#34195=CARTESIAN_POINT ( 'NONE',  ( -2.581517684854000017, -78.37446617076199118, -9.391243908516001326 ) ) ;
#34197=DIRECTION ( 'NONE',  ( 1.000000000000000000, 0.000000000000000000, 0.000000000000000000 ) ) ;
#34205=CARTESIAN_POINT ( 'NONE',  ( 8.787724721424778451, -79.46806983379561018, -3.732128204872922961 ) ) ;
#34206=CARTESIAN_POINT ( 'NONE',  ( 0.009747935475830782001, -79.99999999999998579, -9.487720945728824518 ) ) ;
#34209=CARTESIAN_POINT ( 'NONE',  ( -9.237809349072998444, -79.23357724651299350, -3.213393753055000079 ) ) ;
#34228=CARTESIAN_POINT ( 'NONE',  ( 5.496668217546000434, -79.88211081103300160, -8.073860231047000013 ) ) ;
#34237=CARTESIAN_POINT ( 'NONE',  ( 7.890405061430818101, -79.05045859552323861, -5.649360742093826104 ) ) ;
#34244=CARTESIAN_POINT ( 'NONE',  ( -0.7262319456430645914, -79.98135051806083595, 9.221384681847585085 ) ) ;
#34245=VERTEX_POINT ( 'NONE', #45783 ) ;
#34248=CARTESIAN_POINT ( 'NONE',  ( -7.103610810849999346, -79.69152403476999780, -8.744578195291998313 ) ) ;
#34249=CARTESIAN_POINT ( 'NONE',  ( 5.439453896751886397, -77.27516157131327645, -7.481521277697023464 ) ) ;
#34255=AXIS2_PLACEMENT_3D ( 'NONE', #17358, #4370, #31205 ) ;
#34256=DIRECTION ( 'NONE',  ( -1.000000000000000000, 0.000000000000000000, 0.000000000000000000 ) ) ;
#34262=CARTESIAN_POINT ( 'NONE',  ( -5.793600105730999594, -78.41198602556298169, 9.408086495002001115 ) ) ;
#34268=CARTESIAN_POINT ( 'NONE',  ( -6.266080380867400379, -77.20000000000001705, 8.932657602619032744 ) ) ;
#34276=CARTESIAN_POINT ( 'NONE',  ( -1.535759092668000036, -78.53095298048599204, 9.397436897434999992 ) ) ;
#34282=CARTESIAN_POINT ( 'NONE',  ( -5.684557159767995138, -78.92708333333335702, 7.396918292183145560 ) ) ;
#34289=CARTESIAN_POINT ( 'NONE',  ( -7.022507694776999543, -79.30009718909599314, 8.434951230355999030 ) ) ;
#34291=CARTESIAN_POINT ( 'NONE',  ( 5.465577009020043953, -80.34583333333198141, 9.484549217282665978 ) ) ;
#34297=DIRECTION ( 'NONE',  ( 1.000000000000000000, 0.000000000000000000, 0.000000000000000000 ) ) ;
#34301=CARTESIAN_POINT ( 'NONE',  ( 3.260743090391000187, -79.53082035574698239, 10.78408470153000032 ) ) ;
#34302=B_SPLINE_CURVE_WITH_KNOTS ( 'NONE', 3,
 ( #39945, #19486, #427, #2080, #56377, #20078, #1788, #28620, #29201, #37479, #42510, #55502, #47246, #42222, #19784, #6778, #25070, #10933 ),
 .UNSPECIFIED., .F., .F.,
 ( 4, 2, 2, 2, 2, 2, 2, 2, 4 ),
 ( 0.000000000000000000, 0.1250000000000000000, 0.2500000000000000000, 0.3750000000000000000, 0.5000000000000000000, 0.6250000000000000000, 0.7500000000000000000, 0.8750000000000000000, 1.000000000000000000 ),
 .UNSPECIFIED. ) ;
#34311=ORIENTED_EDGE ( 'NONE', *, *, #14207, .T. ) ;
#34320=CARTESIAN_POINT ( 'NONE',  ( -3.149542236319641475, -78.19745273510419281, -8.697855718134043457 ) ) ;
#34321=CARTESIAN_POINT ( 'NONE',  ( 7.348709943010458545, -79.30274935012705839, 5.745885650500440534 ) ) ;
#34325=CARTESIAN_POINT ( 'NONE',  ( -3.175871872419103070, -77.50302735801024312, 8.687844134873774493 ) ) ;
#34328=CARTESIAN_POINT ( 'NONE',  ( 10.86862532138017912, -78.33584017775066854, -1.957230818804968520 ) ) ;
#34329=CARTESIAN_POINT ( 'NONE',  ( -8.592320330817999618, -78.29168487677797827, 4.510292750937000328 ) ) ;
#34333=CARTESIAN_POINT ( 'NONE',  ( -10.49924843836999955, -80.39917579582198925, -4.054558598941000014 ) ) ;
#34343=CARTESIAN_POINT ( 'NONE',  ( 1.211018816713875124, -79.46477661281171834, 9.190900382934870549 ) ) ;
#34344=CARTESIAN_POINT ( 'NONE',  ( -10.78747482502000032, -79.91111849808099521, 2.492395449116000083 ) ) ;
#34355=CARTESIAN_POINT ( 'NONE',  ( -9.601393729781001696, -79.88570935437299170, 0.8896799134053999802 ) ) ;
#34360=CARTESIAN_POINT ( 'NONE',  ( 1.439896632895334649, -77.33541666666666003, -10.99999999999999822 ) ) ;
#34362=CARTESIAN_POINT ( 'NONE',  ( 9.237438452994998883, -77.51063887770899896, -6.076007254799000279 ) ) ;
#34386=ADVANCED_FACE ( 'NONE', ( #14742 ), #10426, .F. ) ;
#34393=CARTESIAN_POINT ( 'NONE',  ( 1.199999995295999877, -81.00000000470399186, 7.000000027760000521 ) ) ;
#34399=DIRECTION ( 'NONE',  ( 0.000000000000000000, -1.000000000000000000, 0.000000000000000000 ) ) ;
#34404=CARTESIAN_POINT ( 'NONE',  ( 2.633009914059649681, -77.20296729498775790, 9.306851964919491849 ) ) ;
#34424=CARTESIAN_POINT ( 'NONE',  ( 8.318585563179999198, -78.11610009011799605, 7.159970128962999780 ) ) ;
#34433=CARTESIAN_POINT ( 'NONE',  ( 5.883202309618000392, -78.07035725226099032, -7.625033806424000637 ) ) ;
#34438=ORIENTED_EDGE ( 'NONE', *, *, #36087, .T. ) ;
#34439=CARTESIAN_POINT ( 'NONE',  ( 9.611650271896824194, -78.90833333333333144, -5.539808784079917281 ) ) ;
#34442=CARTESIAN_POINT ( 'NONE',  ( -10.10513987668000091, -78.40210692446099472, -4.192131248929999998 ) ) ;
#34444=CARTESIAN_POINT ( 'NONE',  ( -1.678309891182000024, -80.29203597816000126, -10.90631216329999909 ) ) ;
#34454=CARTESIAN_POINT ( 'NONE',  ( -2.217000330786000450, -79.52338147675502000, 9.512392227823999846 ) ) ;
#34455=EDGE_LOOP ( 'NONE', ( #26044, #55307, #11121, #44363 ) ) ;
#34462=DIRECTION ( 'NONE',  ( 1.000000000000000000, 0.000000000000000000, 0.000000000000000000 ) ) ;
#34464=EDGE_CURVE ( 'NONE', #51092, #41582, #34675, .T. ) ;
#34467=CARTESIAN_POINT ( 'NONE',  ( 9.249909156602798888, -78.84782921127370514, -0.2699301895770213067 ) ) ;
#34480=CARTESIAN_POINT ( 'NONE',  ( 7.531584214675000055, -77.32165489554499516, 5.594615735256000200 ) ) ;
#34484=VECTOR ( 'NONE', #44520, 1000.000000000000114 ) ;
#34486=CARTESIAN_POINT ( 'NONE',  ( 5.110488341091000031, -78.60185680379399287, 8.291116005822999568 ) ) ;
#34495=CARTESIAN_POINT ( 'NONE',  ( -9.324131985855107274, -79.26576877103842378, -1.871943872962896105 ) ) ;
#34496=CARTESIAN_POINT ( 'NONE',  ( -6.215025413931507536, -80.00000000000000000, -7.018981048385420252 ) ) ;
#34499=CARTESIAN_POINT ( 'NONE',  ( 9.459667290369997872, -80.04440615245599133, 2.889698063178000265 ) ) ;
#34501=CARTESIAN_POINT ( 'NONE',  ( 9.611650271896847286, -78.80833333333333712, -5.539808784079878201 ) ) ;
#34508=ORIENTED_EDGE ( 'NONE', *, *, #27593, .F. ) ;
#34515=CARTESIAN_POINT ( 'NONE',  ( -2.217000330786000450, -79.10276701284199419, 9.512392227823999846 ) ) ;
#34523=CARTESIAN_POINT ( 'NONE',  ( -8.796335266380014062, -77.64791666666667425, 6.760013919724027431 ) ) ;
#34524=LINE ( 'NONE', #16834, #6290 ) ;
#34528=CYLINDRICAL_SURFACE ( 'NONE', #50369, 1.000000000000000000 ) ;
#34529=EDGE_CURVE ( 'NONE', #10810, #58355, #26815, .T. ) ;
#34537=CARTESIAN_POINT ( 'NONE',  ( 10.83613785003000096, -78.84875340478899375, -3.083350589994000135 ) ) ;
#34538=CARTESIAN_POINT ( 'NONE',  ( 4.461117935985351224, -77.26506148592295631, -8.103638615493796493 ) ) ;
#34545=CARTESIAN_POINT ( 'NONE',  ( -5.539808784079933268, -78.51666666666667993, 9.611650271896811759 ) ) ;
#34549=CARTESIAN_POINT ( 'NONE',  ( 9.014082483815000657, -78.75678530967299196, -6.575554473347999362 ) ) ;
#34558=DIRECTION ( 'NONE',  ( 0.000000000000000000, -1.000000000000000000, 0.000000000000000000 ) ) ;
#34564=CARTESIAN_POINT ( 'NONE',  ( -9.269208960685000775, -78.16144320180897864, -2.179940704506999616 ) ) ;
#34575=CARTESIAN_POINT ( 'NONE',  ( -10.13785388426000011, -78.40114185044998862, -4.205702700205000255 ) ) ;
#34589=CARTESIAN_POINT ( 'NONE',  ( -3.642272407944000090, -79.27798916675298813, -10.66127506782999923 ) ) ;
#34609=CARTESIAN_POINT ( 'NONE',  ( -1.020496043806678133, -78.21636009095580278, -9.194640008617911420 ) ) ;
#34613=ORIENTED_EDGE ( 'NONE', *, *, #13444, .T. ) ;
#34614=CARTESIAN_POINT ( 'NONE',  ( -1.980088454537020981, -77.49218653272571089, 9.036431384186325744 ) ) ;
#34615=CARTESIAN_POINT ( 'NONE',  ( -9.177034484502000211, -77.26263836681899022, 6.137278520473000043 ) ) ;
#34618=CARTESIAN_POINT ( 'NONE',  ( -6.766389538252999714, -77.89375126897199664, -6.956053621355001049 ) ) ;
#34621=CARTESIAN_POINT ( 'NONE',  ( 3.942135768300999654, -80.08362823344599235, -10.54187931140000067 ) ) ;
#34631=CARTESIAN_POINT ( 'NONE',  ( 1.210855936474563910, -78.46461170675218000, 9.190418661073644913 ) ) ;
#34638=CARTESIAN_POINT ( 'NONE',  ( -5.539808784079931492, -80.11666666668466519, 9.611650271896815312 ) ) ;
#34644=CARTESIAN_POINT ( 'NONE',  ( 2.940699877186000233, -79.37056235426499029, 8.954246345182999889 ) ) ;
#34645=DIRECTION ( 'NONE',  ( -7.074008051008000492E-10, -1.000000000000000000, -4.749370611643999689E-10 ) ) ;
#34648=DIRECTION ( 'NONE',  ( 0.000000000000000000, -0.7071067811866525998, -0.7071067811864425456 ) ) ;
#34652=CARTESIAN_POINT ( 'NONE',  ( -10.52498723879999964, -77.28216120838598613, 3.387147871870999971 ) ) ;
#34657=CARTESIAN_POINT ( 'NONE',  ( -0.5065222552852000071, -77.14901792243969680, 9.658707080791000266 ) ) ;
#34675=B_SPLINE_CURVE_WITH_KNOTS ( 'NONE', 3,
 ( #25217, #43237, #24932, #2508, #2794, #37632, #55650, #33190, #46819, #26076 ),
 .UNSPECIFIED., .F., .F.,
 ( 4, 2, 2, 2, 4 ),
 ( 0.000000000000000000, 0.2500000000000000000, 0.5000000000000000000, 0.7500000000000000000, 1.000000000000000000 ),
 .UNSPECIFIED. ) ;
#34680=ORIENTED_EDGE ( 'NONE', *, *, #2312, .F. ) ;
#34681=CARTESIAN_POINT ( 'NONE',  ( -9.250000000000000000, -79.49999999999998579, 1.813240672189999963E-14 ) ) ;
#34683=EDGE_CURVE ( 'NONE', #44715, #43667, #32243, .T. ) ;
#34688=LINE ( 'NONE', #48018, #31482 ) ;
#34692=CARTESIAN_POINT ( 'NONE',  ( 9.100870196628985553, -77.07242046014692960, -3.274811821655061017 ) ) ;
#34695=CARTESIAN_POINT ( 'NONE',  ( -8.513832829815155989, -78.63200474943408835, -3.619427496593546678 ) ) ;
#34697=CARTESIAN_POINT ( 'NONE',  ( -10.95040223189505468, -80.10793889166065185, -1.053133452593003838 ) ) ;
#34700=CARTESIAN_POINT ( 'NONE',  ( -5.799999999999999822, -80.99999999999998579, 0.000000000000000000 ) ) ;
#34720=CARTESIAN_POINT ( 'NONE',  ( 0.8456326333846000409, -78.58901425910798366, -9.484475825334998333 ) ) ;
#34725=ADVANCED_FACE ( 'NONE', ( #49707, #28109 ), #50286, .F. ) ;
#34731=CARTESIAN_POINT ( 'NONE',  ( 10.28297802758999957, -78.09309102680099102, -3.734674224488999883 ) ) ;
#34733=CARTESIAN_POINT ( 'NONE',  ( 10.59805651207999944, -80.08569813701798523, 4.006234447635000251 ) ) ;
#34761=CARTESIAN_POINT ( 'NONE',  ( 5.492755632425520673, -77.13749999994708162, -7.555491190735147633 ) ) ;
#34763=CARTESIAN_POINT ( 'NONE',  ( 5.539808784079867543, -77.93333333333333712, 9.611650271896852615 ) ) ;
#34765=CARTESIAN_POINT ( 'NONE',  ( 1.748323643227931434, -79.96240695551148292, 10.92574688943145844 ) ) ;
#34786=CARTESIAN_POINT ( 'NONE',  ( -3.141535938717197496, -79.15175190257748739, 8.986458492157693101 ) ) ;
#34791=CARTESIAN_POINT ( 'NONE',  ( -9.582886764941999758, -79.13235384747198964, 1.297353921085000028 ) ) ;
#34803=CARTESIAN_POINT ( 'NONE',  ( 7.985065670160999218, -77.74030535679999332, 7.712612023391999472 ) ) ;
#34804=DIRECTION ( 'NONE',  ( 0.000000000000000000, 1.000000000000000000, 0.000000000000000000 ) ) ;
#34808=CARTESIAN_POINT ( 'NONE',  ( 1.739862777674999972, -79.07029435458399291, 9.611119481339999382 ) ) ;
#34815=CARTESIAN_POINT ( 'NONE',  ( 5.417173251955453850, -79.02203476639424196, -8.051588635942257710 ) ) ;
#34823=CARTESIAN_POINT ( 'NONE',  ( -0.7835675759065233725, -79.98183763911107746, 9.216734333713379357 ) ) ;
#34825=EDGE_LOOP ( 'NONE', ( #12039, #41446, #2027 ) ) ;
#34826=CARTESIAN_POINT ( 'NONE',  ( -9.688835989853998854, -79.66343168043698597, -5.749381838710999837 ) ) ;
#34827=CARTESIAN_POINT ( 'NONE',  ( 8.684857183346831988, -77.32189494946037200, -3.221164999357318592 ) ) ;
#34836=CARTESIAN_POINT ( 'NONE',  ( -9.595360835209000072, -79.59955593965399601, -5.693913425678999829 ) ) ;
#34842=CARTESIAN_POINT ( 'NONE',  ( -3.820214278402727093, -77.19999999999998863, 10.15434263821451566 ) ) ;
#34849=CARTESIAN_POINT ( 'NONE',  ( 9.589208240076997569, -78.96433849994599541, 0.8944121949827000817 ) ) ;
#34851=EDGE_CURVE ( 'NONE', #54228, #29062, #49449, .T. ) ;
#34852=FACE_OUTER_BOUND ( 'NONE', #31214, .T. ) ;
#34863=CARTESIAN_POINT ( 'NONE',  ( 7.788493169598000421, -78.68206539377699471, 7.733265204867000087 ) ) ;
#34870=CARTESIAN_POINT ( 'NONE',  ( 5.452652381452083752, -77.32493831431021647, 7.507522693077579135 ) ) ;
#34871=CARTESIAN_POINT ( 'NONE',  ( -10.71369944335148361, -78.17916666666667425, 2.879226727952040044 ) ) ;
#34873=CARTESIAN_POINT ( 'NONE',  ( -10.30593458266999995, -78.27435544289399161, -4.275431210322000020 ) ) ;
#34886=ORIENTED_EDGE ( 'NONE', *, *, #21888, .F. ) ;
#34897=CARTESIAN_POINT ( 'NONE',  ( -5.437822718421641888, -77.52503815049138325, 7.482785194970384524 ) ) ;
#34898=CARTESIAN_POINT ( 'NONE',  ( 10.94195044575999987, -77.54892574480697931, -1.468969119710000104 ) ) ;
#34901=CARTESIAN_POINT ( 'NONE',  ( 8.444976262095000408, -78.12114190200398411, 4.780490068936999570 ) ) ;
#34906=CARTESIAN_POINT ( 'NONE',  ( -3.493617039247999934, -80.46877773805297807, -10.33892454317000187 ) ) ;
#34908=CARTESIAN_POINT ( 'NONE',  ( 4.658475568430830549, -78.66666666666665719, -8.082524092276877070 ) ) ;
#34928=CARTESIAN_POINT ( 'NONE',  ( 6.249458598087999306, -79.83812488639198079, 7.054820424332000073 ) ) ;
#34942=CARTESIAN_POINT ( 'NONE',  ( 7.559982449049000408, -76.90594942799179989, -6.032732969207000195 ) ) ;
#34946=CARTESIAN_POINT ( 'NONE',  ( 4.299999999999999822, -81.99999999999998579, 0.000000000000000000 ) ) ;
#34948=EDGE_LOOP ( 'NONE', ( #4775, #14147, #22272, #1238 ) ) ;
#34950=DIRECTION ( 'NONE',  ( -3.675129103447999014E-09, -0.9999999999999997780, 2.168720876821999677E-08 ) ) ;
#34960=AXIS2_PLACEMENT_3D ( 'NONE', #24425, #38860, #28833 ) ;
#34965=ORIENTED_EDGE ( 'NONE', *, *, #37116, .T. ) ;
#34997=CARTESIAN_POINT ( 'NONE',  ( -5.539808784079887083, -79.78333333333333144, -9.611650271896841957 ) ) ;
#35007=CARTESIAN_POINT ( 'NONE',  ( 2.217690073412000196, -79.10064318342999456, -9.260249588150999855 ) ) ;
#35012=CARTESIAN_POINT ( 'NONE',  ( 2.365578933032910669, -78.95508126976140773, 9.023057518257136422 ) ) ;
#35019=EDGE_LOOP ( 'NONE', ( #46925, #13465, #13328, #38615, #21323, #43049, #38465, #14138, #36488 ) ) ;
#35022=ORIENTED_EDGE ( 'NONE', *, *, #54521, .T. ) ;
#35037=CARTESIAN_POINT ( 'NONE',  ( 8.545990964147081925, -78.81890182048778115, -3.539321513413446585 ) ) ;
#35042=LINE ( 'NONE', #8486, #292 ) ;
#35043=CARTESIAN_POINT ( 'NONE',  ( -10.71369944335148183, -78.07916666666665151, 2.879226727952040932 ) ) ;
#35045=CARTESIAN_POINT ( 'NONE',  ( -6.272971974831354380, -80.02293377770999427, 9.114735501174534349 ) ) ;
#35049=CARTESIAN_POINT ( 'NONE',  ( -6.176117940694000552, -77.38832598960298981, 7.205939610817000407 ) ) ;
#35063=CARTESIAN_POINT ( 'NONE',  ( -2.546082409442600447, -79.14654788605089664, 9.173657452411669411 ) ) ;
#35066=CARTESIAN_POINT ( 'NONE',  ( -10.71369944335148183, -79.07916666666666572, 2.879226727952040932 ) ) ;
#35069=CARTESIAN_POINT ( 'NONE',  ( 1.673403667841999898, -79.34562022128699255, -9.636531604483000280 ) ) ;
#35073=DIRECTION ( 'NONE',  ( -0.3090169943748909409, 0.000000000000000000, 0.9510565162951718499 ) ) ;
#35075=DIRECTION ( 'NONE',  ( 0.000000000000000000, 1.000000000000000000, 0.000000000000000000 ) ) ;
#35090=CARTESIAN_POINT ( 'NONE',  ( 9.647254834573999460, -80.00735905321899111, -1.526580663425000095 ) ) ;
#35098=LINE ( 'NONE', #57552, #4678 ) ;
#35105=CARTESIAN_POINT ( 'NONE',  ( 1.403051294136565819, -79.96338502862796815, 9.142673906005519768 ) ) ;
#35108=CARTESIAN_POINT ( 'NONE',  ( 4.209725253073815843, -77.26262135689660226, -8.236522718530926213 ) ) ;
#35111=CONICAL_SURFACE ( 'NONE', #4973, 5.249999999862000166, 0.7853981633972997312 ) ;
#35120=CARTESIAN_POINT ( 'NONE',  ( 9.178372771442999678, -78.26048704979598369, -6.069379357596000446 ) ) ;
#35132=VECTOR ( 'NONE', #22672, 1000.000000000000000 ) ;
#35145=CARTESIAN_POINT ( 'NONE',  ( -4.399243655502999673, -79.83797013842199419, 10.05537673064999815 ) ) ;
#35149=CARTESIAN_POINT ( 'NONE',  ( 9.415891442473027340, -79.15074836997709440, 0.09954902595250748887 ) ) ;
#35153=DIRECTION ( 'NONE',  ( 0.000000000000000000, -1.000000000000000000, 0.000000000000000000 ) ) ;
#35154=CARTESIAN_POINT ( 'NONE',  ( 10.38514225167999960, -78.02921528601798684, -3.771779243421000238 ) ) ;
#35157=VECTOR ( 'NONE', #33335, 1000.000000000000000 ) ;
#35167=B_SPLINE_CURVE_WITH_KNOTS ( 'NONE', 3,
 ( #33463, #55327, #29040, #46497, #20197, #55621, #55036, #42632, #6899, #24907, #51210, #10762, #50914, #28741, #19905, #42345, #37898, #24619, #15757, #51501, #11058, #47080, #1327, #32577, #42925, #56209, #19029, #33752, #14584, #50624, #28152, #46204, #5728, #23738, #41752, #32869, #19321, #10462, #28448, #6021, #24031, #48505, #25769, #2479, #30478, #20483, #29607, #8050, #43495, #56784, #12760, #52927, #39630, #7479, #20767, #26046, #44070, #11913, #3057, #16052, #38479, #48231, #12197, #39054, #12477, #57636, #30757, #53213, #7766, #56497, #25477, #30181, #38766, #34035, #3340, #17192, #21335, #25189, #3619, #34897, #52074, #52642, #21052, #21625, #35181, #39347, #57355, #48790, #16918, #43209, #11632, #26334, #43791, #8335, #47663, #7189, #2768, #16346, #34325, #52361, #29890, #47947, #57068, #16628, #34614, #53502, #18081, #44650, #45540, #40802, #687, #39915, #35473, #36076, #44350, #9221, #18669, #5085, #21906, #18373, #22202, #4205, #9806, #54676, #13637, #31633, #8629, #13044, #54097, #49379, #13338, #44946, #3903, #31335, #396, #8926, #49675, #27206, #45245, #54393, #4793, #57931, #22793, #26615, #40213, #17486, #36658, #36367, #23081, #14218, #13930, #31925, #58224, #17787, #32215, #49970, #35776, #9513, #50257, #53804, #41095, #31042, #49079, #27499, #26915, #4502, #22501, #40512, #14799, #46417, #15095, #15683, #15395, #32502, #33389, #55844, #10688, #46130, #33092, #33679, #55544, #45835, #24254, #51134, #971, #51426, #42269, #5654, #37824, #55252, #10982, #28372, #5370, #28962, #51717, #56134, #5947, #1541, #1256, #23951, #28668, #41968, #19533, #23663, #19831, #47004, #27789, #19244, #37237, #23378, #6238, #50840, #6531, #41675, #41388, #24543, #18954, #32793, #42557, #10387, #37526, #46718, #1835, #2124, #20124, #28080, #38113, #36947, #54960, #14511, #50547, #10100, #20408, #38402, #7401, #30399, #47871, #39270, #21554, #29821, #25404, #34827, #48158, #56423, #12409, #3272, #57281, #56993, #2980, #52571, #43420, #7689, #20978, #15973, #56713, #16270, #11267, #38982, #43141, #16555, #43719, #16845, #57563, #30107, #12122, #44001, #52855, #25974, #33965, #52284, #24832, #52002, #48435, #25690, #7977, #11556, #34249, #29534, #3551, #6822, #11840, #34538, #47591, #21264, #7117, #39559, #17125, #35108, #42848, #25117, #29247, #47295, #2407, #2700, #20694, #38693, #53429, #23016, #40737, #44573, #40441, #22724, #48722, #35703, #27434, #13862, #31558, #49007, #49304, #328, #18010, #53144, #18306, #12692, #21837, #36299 ),
 .UNSPECIFIED., .F., .F.,
 ( 4, 2, 2, 1, 1, 1, 1, 1, 2, 2, 2, 2, 2, 1, 1, 1, 2, 2, 2, 2, 2, 2, 2, 1, 1, 1, 1, 1, 2, 2, 2, 2, 1, 1, 2, 2, 2, 1, 1, 1, 1, 2, 2, 2, 2, 2, 1, 1, 1, 1, 2, 2, 2, 2, 2, 1, 1, 1, 1, 2, 2, 2, 2, 2, 2, 2, 2, 1, 1, 1, 1, 2, 2, 2, 2, 1, 1, 1, 1, 1, 2, 2, 2, 2, 2, 1, 1, 2, 2, 2, 2, 2, 1, 1, 2, 2, 2, 2, 1, 1, 1, 1, 2, 2, 2, 2, 2, 2, 2, 1, 1, 1, 1, 1, 2, 2, 1, 1, 1, 1, 1, 1, 2, 2, 2, 2, 2, 1, 1, 1, 1, 2, 2, 2, 2, 1, 1, 2, 2, 2, 2, 1, 1, 2, 2, 2, 2, 1, 1, 1, 1, 2, 2, 2, 2, 2, 2, 2, 1, 1, 1, 1, 2, 2, 2, 2, 1, 2, 2, 2, 2, 1, 1, 1, 1, 1, 2, 2, 2, 2, 2, 1, 1, 1, 1, 2, 2, 2, 2, 2, 1, 1, 1, 1, 1, 2, 2, 2, 2, 2, 4 ),
 ( 0.000000000000000000, 0.01562500000005664219, 0.02343750000008496329, 0.02734375000009912904, 0.02929687500010621365, 0.03027343750010977330, 0.03076171875011152884, 0.03100585937511241008, 0.03112792968761284029, 0.03125000000011327050, 0.04687500000016913554, 0.05468750000019706459, 0.05859375000021103258, 0.06054687500021796454, 0.06152343750022142704, 0.06201171875022322422, 0.06225585937522412627, 0.06250000000022502833, 0.07812500000022287727, 0.09375000000022072622, 0.1093750000002185613, 0.1171875000002174511, 0.1210937500002169098, 0.1230468750002166461, 0.1240234375002165074, 0.1245117187502164519, 0.1247558593752164380, 0.1248779296877164380, 0.1249389648439664241, 0.1250000000002164102, 0.1328125000002231826, 0.1367187500002266520, 0.1386718750002283451, 0.1396484375002291778, 0.1401367187502295941, 0.1406250000002300105, 0.1484375000002361999, 0.1523437500002392531, 0.1542968750002407519, 0.1552734375002415568, 0.1557617187502419454, 0.1560058593752421396, 0.1562500000002423062, 0.1718750000002544354, 0.1796875000002605416, 0.1835937500002635669, 0.1855468750002650935, 0.1865234375002658429, 0.1870117187502662315, 0.1872558593752664258, 0.1873779296877665090, 0.1875000000002665923, 0.2031250000002769174, 0.2109375000002820522, 0.2148437500002845779, 0.2167968750002858824, 0.2177734375002865208, 0.2182617187502868539, 0.2185058593752870482, 0.2186279296877871314, 0.2187500000002871869, 0.2343750000002968459, 0.2421875000003016754, 0.2460937500003040623, 0.2500000000003064216, 0.2656250000003159140, 0.2734375000003206879, 0.2773437500003230749, 0.2792968750003242406, 0.2802734375003248513, 0.2807617187503251843, 0.2810058593753253509, 0.2812500000003255174, 0.2968750000003349543, 0.3046875000003396727, 0.3085937500003420042, 0.3105468750003432254, 0.3115234375003438361, 0.3120117187503441136, 0.3122558593753442802, 0.3123779296878443357, 0.3125000000003443357, 0.3281250000003541056, 0.3359375000003589351, 0.3398437500003613221, 0.3417968750003624878, 0.3427734375003629874, 0.3432617187503632650, 0.3437500000003635425, 0.3515625000003680389, 0.3554687500003703149, 0.3574218750003714251, 0.3583984375003719802, 0.3588867187503722578, 0.3591308593753724243, 0.3593750000003725908, 0.3671875000003768097, 0.3710937500003789191, 0.3730468750003799183, 0.3740234375003804179, 0.3745117187503806400, 0.3747558593753807510, 0.3748779296878808065, 0.3750000000003808620, 0.4062500000003944067, 0.4375000000004078959, 0.4687500000004214407, 0.4843750000004282685, 0.4921875000004316547, 0.4960937500004333200, 0.4980468750004342082, 0.4990234375004343748, 0.4995117187504344303, 0.4997558593754346523, 0.4998779296879345968, 0.5000000000004345413, 0.5156250000004241052, 0.5234375000004188871, 0.5273437500004162226, 0.5292968750004148903, 0.5302734375004141132, 0.5307617187504137801, 0.5310058593754136691, 0.5312500000004135581, 0.5468750000004045653, 0.5546875000004000134, 0.5585937500003976819, 0.5605468750003965717, 0.5615234375003960166, 0.5620117187503956835, 0.5622558593753955725, 0.5623779296878954614, 0.5625000000003953504, 0.5781250000003820277, 0.5859375000003753664, 0.5898437500003721468, 0.5917968750003703704, 0.5927734375003694822, 0.5937500000003685940, 0.6015625000003618217, 0.6054687500003584910, 0.6074218750003568257, 0.6083984375003558265, 0.6088867187503553824, 0.6093750000003549383, 0.6171875000003481659, 0.6210937500003448353, 0.6230468750003431699, 0.6240234375003422818, 0.6245117187503418377, 0.6247558593753416156, 0.6248779296878415046, 0.6250000000003412826, 0.6562500000003149703, 0.6875000000002885470, 0.7187500000002622347, 0.7343750000002490230, 0.7421875000002423617, 0.7460937500002389200, 0.7480468750002372547, 0.7490234375002363665, 0.7495117187502359224, 0.7497558593752357003, 0.7500000000002354783, 0.7656250000002193801, 0.7734375000002113865, 0.7773437500002073897, 0.7792968750002053913, 0.7812500000002032818, 0.7968750000001869616, 0.8046875000001787459, 0.8085937500001746381, 0.8105468750001726397, 0.8115234375001716405, 0.8120117187501710854, 0.8122558593751708633, 0.8123779296876707523, 0.8125000000001706413, 0.8281250000001512124, 0.8359375000001415534, 0.8398437500001367795, 0.8417968750001343370, 0.8427734375001331157, 0.8432617187501324496, 0.8435058593751321165, 0.8436279296876320055, 0.8437500000001318945, 0.8593750000001109113, 0.8671875000001003642, 0.8710937500000951461, 0.8730468750000924816, 0.8740234375000911493, 0.8745117187500904832, 0.8747558593750902611, 0.8748779296875901501, 0.8749389648438401501, 0.8750000000000900391, 0.9062500000000676126, 0.9375000000000450751, 0.9687500000000226485, 1.000000000000000000 ),
 .UNSPECIFIED. ) ;
#35169=CARTESIAN_POINT ( 'NONE',  ( 8.597946777922295780, -79.53556089611873858, 4.122091896699570768 ) ) ;
#35173=ADVANCED_FACE ( 'NONE', ( #1947 ), #42951, .T. ) ;
#35174=AXIS2_PLACEMENT_3D ( 'NONE', #12374, #17090, #53391 ) ;
#35177=CARTESIAN_POINT ( 'NONE',  ( -6.528096133866698736, -78.16282450551233296, -6.553206690438871718 ) ) ;
#35181=CARTESIAN_POINT ( 'NONE',  ( -4.564206451014241495, -77.51613632694960643, 8.045838294816407554 ) ) ;
#35184=CARTESIAN_POINT ( 'NONE',  ( 8.444976262095000408, -78.18144482767498005, 4.780490068936999570 ) ) ;
#35188=CARTESIAN_POINT ( 'NONE',  ( -8.254612054926999676, -79.93512533242399343, 6.886499823760000361 ) ) ;
#35192=CARTESIAN_POINT ( 'NONE',  ( -9.250000000000000000, -78.49999999999998579, 0.000000000000000000 ) ) ;
#35213=CARTESIAN_POINT ( 'NONE',  ( 8.183515395032999962, -79.31211703774899036, 4.675091623977000843 ) ) ;
#35215=CARTESIAN_POINT ( 'NONE',  ( -0.001775305735512080086, -77.22499999999998010, -11.03387446371952940 ) ) ;
#35225=CARTESIAN_POINT ( 'NONE',  ( 9.208615812369000508, -77.04458045456699722, 2.957800710608999850 ) ) ;
#35246=CARTESIAN_POINT ( 'NONE',  ( -9.254388464354001087, -79.90752053325199711, 5.469807505829999528 ) ) ;
#35252=CARTESIAN_POINT ( 'NONE',  ( -10.84202097104999929, -77.33490313763715562, 2.082001701158999740 ) ) ;
#35258=DIRECTION ( 'NONE',  ( -1.000000000000000000, 0.000000000000000000, 0.000000000000000000 ) ) ;
#35277=FACE_OUTER_BOUND ( 'NONE', #20957, .T. ) ;
#35289=CARTESIAN_POINT ( 'NONE',  ( 7.685661446562000343, -76.94999999999998863, -5.583959896778000420 ) ) ;
#35292=CARTESIAN_POINT ( 'NONE',  ( -9.612747958823000261, -77.38818535316599423, 0.5898851805584999219 ) ) ;
#35303=CARTESIAN_POINT ( 'NONE',  ( 7.195688986358000250, -79.18869284577598933, 8.240744890341000328 ) ) ;
#35305=CARTESIAN_POINT ( 'NONE',  ( -1.882622766709999951, -79.91865347566299249, -11.17249270816999918 ) ) ;
#35310=EDGE_LOOP ( 'NONE', ( #42769, #45233, #24464, #9067, #5207, #45661 ) ) ;
#35312=CARTESIAN_POINT ( 'NONE',  ( 6.728605944993000243, -79.93548824452055612, -7.080011783993000130 ) ) ;
#35328=CARTESIAN_POINT ( 'NONE',  ( 9.195972239629917055, -78.84146734569272041, -1.008436867448839758 ) ) ;
#35329=ADVANCED_FACE ( 'NONE', ( #42082 ), #51422, .F. ) ;
#35338=CARTESIAN_POINT ( 'NONE',  ( 10.80348683896753137, -79.86729337777099147, 2.390241153868426505 ) ) ;
#35362=CARTESIAN_POINT ( 'NONE',  ( 7.050245828045000884, -80.01787806992999208, 6.779143932755000712 ) ) ;
#35378=CARTESIAN_POINT ( 'NONE',  ( 9.226480760116999136, -78.94040372155198781, -2.263195259622999611 ) ) ;
#35382=DIRECTION ( 'NONE',  ( 0.000000000000000000, -1.000000000000000000, 0.000000000000000000 ) ) ;
#35385=CARTESIAN_POINT ( 'NONE',  ( 0.8618151749125838590, -78.48198201294394494, -9.665976535993026530 ) ) ;
#35396=CARTESIAN_POINT ( 'NONE',  ( -11.19646453606000058, -79.12967694811598562, -1.252244488204000028 ) ) ;
#35405=AXIS2_PLACEMENT_3D ( 'NONE', #12098, #34804, #16820 ) ;
#35407=CARTESIAN_POINT ( 'NONE',  ( -10.76843015134999959, -79.98515786819298512, 1.073136842994000029 ) ) ;
#35419=CARTESIAN_POINT ( 'NONE',  ( -9.254388464354001087, -79.90752053325199711, 5.469807505829999528 ) ) ;
#35423=CARTESIAN_POINT ( 'NONE',  ( -5.250896469870999006, -77.56454279010098674, 7.943454065752000304 ) ) ;
#35435=CARTESIAN_POINT ( 'NONE',  ( -10.57157196544999955, -79.91288308330898360, 2.324769239444999691 ) ) ;
#35436=CARTESIAN_POINT ( 'NONE',  ( -2.831617975195505288, -80.38489583333210931, 10.53328982651339629 ) ) ;
#35445=B_SPLINE_CURVE_WITH_KNOTS ( 'NONE', 3,
 ( #55410, #1697, #5236, #14956, #46285, #10847, #24412, #6106, #42131, #42428, #19691, #9962, #41248, #51584, #32954, #15552, #28530, #37978, #50999, #46579, #1997, #23241, #10250, #19991, #6397, #37691, #23527, #41835, #15257, #37100, #33545, #55710, #41539, #54829, #56002, #27655, #1121, #45697, #836, #18818, #32658, #36810, #14370, #32370, #50412, #27943, #45991, #19109, #55116, #14660, #50709, #11423, #48310, #39434, #3425, #56867, #16137, #56577, #16715, #52438, #43292, #33831, #24702, #11142, #29976, #20845, #43581, #47162, #2848, #11713, #34697, #7849, #48029, #7561 ),
 .UNSPECIFIED., .F., .F.,
 ( 4, 2, 2, 2, 2, 2, 2, 1, 1, 1, 1, 2, 2, 2, 2, 2, 1, 1, 1, 2, 2, 2, 2, 2, 1, 1, 1, 2, 2, 2, 2, 2, 1, 1, 1, 1, 2, 2, 1, 2, 2, 1, 1, 1, 2, 4 ),
 ( 0.000000000000000000, 0.04346818531367174082, 0.08693637062734348164, 0.1086704632841794249, 0.1195375096125975006, 0.1249710327768065871, 0.1253106279745698770, 0.1256502231723332086, 0.1263294135678600105, 0.1276877943589138642, 0.1304045559410215438, 0.1738727412547442785, 0.2173409265684669855, 0.2390750192253283946, 0.2499420655537591407, 0.2506212559492860814, 0.2513004463448130776, 0.2526588271358671256, 0.2553755887179749995, 0.2608091118821907473, 0.3477454825096416569, 0.3694795751665044259, 0.3749130983307200626, 0.3755922887262470033, 0.3762714791217740551, 0.3776298599128280475, 0.3803466214949359214, 0.3912136678233673059, 0.4346818531370924554, 0.4781500384508176604, 0.4998841311076802629, 0.5005633215032072592, 0.5012425118987341444, 0.5026008926897881368, 0.5053176542718960107, 0.5107511774361116474, 0.5216182237645430320, 0.6085545943919933309, 0.6194216407204246044, 0.6248551638846403522, 0.6255343542801672374, 0.6262135446756940116, 0.6275719254667480040, 0.6302886870488556559, 0.6520227797057175367, 0.6954909650194412984 ),
 .UNSPECIFIED. ) ;
#35446=CARTESIAN_POINT ( 'NONE',  ( -7.730500772889000061, -79.67897315952798465, 8.045567737375000306 ) ) ;
#35450=AXIS2_PLACEMENT_3D ( 'NONE', #31374, #49417, #40251 ) ;
#35468=CARTESIAN_POINT ( 'NONE',  ( -5.132841502757762520, -78.17821230117139919, -7.695201808387375664 ) ) ;
#35473=CARTESIAN_POINT ( 'NONE',  ( -1.453085306447361003, -77.48762070070470998, 9.135110569084051946 ) ) ;
#35474=CARTESIAN_POINT ( 'NONE',  ( 3.792698199283999649, -77.96245195745699164, -10.36819406884000117 ) ) ;
#35476=CARTESIAN_POINT ( 'NONE',  ( 4.746041175454999816, -77.49581766116699555, -8.464384343845999581 ) ) ;
#35480=CARTESIAN_POINT ( 'NONE',  ( 8.693423296916000353, -80.06508647311397908, -7.148151291522000683 ) ) ;
#35496=CARTESIAN_POINT ( 'NONE',  ( -11.04620438670000127, -80.55603373794698996, 0.1137957503148000066 ) ) ;
#35501=AXIS2_PLACEMENT_3D ( 'NONE', #43651, #47808, #12063 ) ;
#35508=CARTESIAN_POINT ( 'NONE',  ( 9.118072387854001093, -79.75045691161798800, -2.384738962471999901 ) ) ;
#35527=LINE ( 'NONE', #40264, #28736 ) ;
#35539=( LENGTH_UNIT ( ) NAMED_UNIT ( * ) SI_UNIT ( .MILLI., .METRE. ) );
#35559=CARTESIAN_POINT ( 'NONE',  ( 1.882180247600000245, -78.56901263324199647, 9.519879562373999349 ) ) ;
#35565=CARTESIAN_POINT ( 'NONE',  ( -9.250000000000000000, -78.59999999999999432, 0.000000000000000000 ) ) ;
#35570=FACE_OUTER_BOUND ( 'NONE', #27699, .T. ) ;
#35585=ORIENTED_EDGE ( 'NONE', *, *, #28250, .T. ) ;
#35590=CARTESIAN_POINT ( 'NONE',  ( 8.085542028362999289, -78.16265682217398592, -5.029352477166999513 ) ) ;
#35597=CARTESIAN_POINT ( 'NONE',  ( 6.760013919724043419, -78.87708333333334565, -8.796335266379996298 ) ) ;
#35605=LINE ( 'NONE', #27913, #34085 ) ;
#35609=VERTEX_POINT ( 'NONE', #25086 ) ;
#35618=CARTESIAN_POINT ( 'NONE',  ( 9.249824691843906876, -79.33960135255351531, -1.210482662510009799 ) ) ;
#35631=DIRECTION ( 'NONE',  ( 0.7071067811864970576, -0.7071067811865969777, 3.680441427362984728E-08 ) ) ;
#35636=FACE_OUTER_BOUND ( 'NONE', #24894, .T. ) ;
#35667=AXIS2_PLACEMENT_3D ( 'NONE', #40889, #10184, #23169 ) ;
#35668=CARTESIAN_POINT ( 'NONE',  ( 0.000000000000000000, -80.99999999999998579, -7.000000000000000000 ) ) ;
#35673=ORIENTED_EDGE ( 'NONE', *, *, #48516, .T. ) ;
#35684=CARTESIAN_POINT ( 'NONE',  ( -9.687172913667000174, -79.78005044541399116, -1.248753675804000096 ) ) ;
#35693=CARTESIAN_POINT ( 'NONE',  ( 9.512289053070713152, -78.08404840513796330, -1.920985361971307537 ) ) ;
#35699=CARTESIAN_POINT ( 'NONE',  ( 5.420624143929649641, -79.92565254368837202, 7.494935276742532793 ) ) ;
#35702=CARTESIAN_POINT ( 'NONE',  ( 9.126884531295068825, -76.97371192633831072, -3.132086699607132374 ) ) ;
#35703=CARTESIAN_POINT ( 'NONE',  ( 2.860640696257633842, -77.25019150838288340, -8.796429361950103498 ) ) ;
#35712=CARTESIAN_POINT ( 'NONE',  ( 1.712298698931000063, -78.41967705768098540, 11.02540857285000087 ) ) ;
#35722=AXIS2_PLACEMENT_3D ( 'NONE', #25940, #8514, #4392 ) ;
#35723=FACE_OUTER_BOUND ( 'NONE', #54734, .T. ) ;
#35736=CARTESIAN_POINT ( 'NONE',  ( -7.022507694776999543, -79.36040011476698908, 8.434951230355999030 ) ) ;
#35743=CARTESIAN_POINT ( 'NONE',  ( 7.483407197968000801, -77.19999999999998863, -5.437013583705000208 ) ) ;
#35746=EDGE_CURVE ( 'NONE', #29444, #1603, #24761, .T. ) ;
#35747=CARTESIAN_POINT ( 'NONE',  ( 0.2656919276500000482, -79.36995726186898992, -11.15441650005999996 ) ) ;
#35764=CARTESIAN_POINT ( 'NONE',  ( 1.870325714029711817, -79.60930526082691472, 9.346613135352017210 ) ) ;
#35765=ORIENTED_EDGE ( 'NONE', *, *, #26606, .T. ) ;
#35768=VECTOR ( 'NONE', #12624, 1000.000000000000000 ) ;
#35774=ORIENTED_EDGE ( 'NONE', *, *, #5199, .T. ) ;
#35776=CARTESIAN_POINT ( 'NONE',  ( 2.773106347243120329, -77.45094825236556346, 8.824487850178316606 ) ) ;
#35777=CARTESIAN_POINT ( 'NONE',  ( -0.5413127449341000874, -78.05124810013299452, -11.02683867434999954 ) ) ;
#35778=CARTESIAN_POINT ( 'NONE',  ( 5.091895231007000255, -78.72149758112600182, 8.260951054388000259 ) ) ;
#35792=ADVANCED_FACE ( 'NONE', ( #18278 ), #17978, .F. ) ;
#35801=CARTESIAN_POINT ( 'NONE',  ( -9.611650271896857944, -80.15833333335581301, 5.539808784079855997 ) ) ;
#35805=DIRECTION ( 'NONE',  ( 0.000000000000000000, 1.000000000000000000, 0.000000000000000000 ) ) ;
#35807=CARTESIAN_POINT ( 'NONE',  ( -1.819771783575000024, -80.13035146897098571, -9.247423239423000041 ) ) ;
#35808=CIRCLE ( 'NONE', #47150, 5.000000000000000000 ) ;
#35817=DIRECTION ( 'NONE',  ( -1.000000000000000000, 0.000000000000000000, 0.000000000000000000 ) ) ;
#35844=CARTESIAN_POINT ( 'NONE',  ( 7.117135278674999732, -80.17052195727752917, 8.718833803912000135 ) ) ;
#35849=ORIENTED_EDGE ( 'NONE', *, *, #18652, .F. ) ;
#35850=CARTESIAN_POINT ( 'NONE',  ( -5.876696946709999203, -77.43033226363316146, -9.346046374399000101 ) ) ;
#35872=EDGE_CURVE ( 'NONE', #5115, #36325, #21715, .T. ) ;
#35873=DIRECTION ( 'NONE',  ( 0.000000000000000000, -1.000000000000000000, 0.000000000000000000 ) ) ;
#35883=B_SPLINE_CURVE_WITH_KNOTS ( 'NONE', 3,
 ( #13375, #52673, #12227, #35215, #30217, #48826, #30510, #39664, #48264, #44687, #3375, #48539, #22237, #3938, #7799, #31372, #13079, #31076 ),
 .UNSPECIFIED., .F., .F.,
 ( 4, 2, 2, 2, 2, 2, 2, 2, 4 ),
 ( 0.000000000000000000, 0.1250000000000000555, 0.2500000000000001110, 0.3750000000000001665, 0.5000000000000001110, 0.6250000000000001110, 0.7500000000000001110, 0.8750000000000000000, 1.000000000000000000 ),
 .UNSPECIFIED. ) ;
#35888=CARTESIAN_POINT ( 'NONE',  ( 9.473958333542425336, -76.97604166667584025, -0.9915651795498008347 ) ) ;
#35891=AXIS2_PLACEMENT_3D ( 'NONE', #52041, #6864, #52327 ) ;
#35892=CARTESIAN_POINT ( 'NONE',  ( 8.297164401012999235, -79.30663806985799624, 4.009864491784999707 ) ) ;
#35902=EDGE_LOOP ( 'NONE', ( #18985, #14861, #29244, #32703, #27702, #54237, #16620, #18291, #37291, #24599, #38312 ) ) ;
#35913=ORIENTED_EDGE ( 'NONE', *, *, #18169, .T. ) ;
#35917=VERTEX_POINT ( 'NONE', #33481 ) ;
#35921=EDGE_CURVE ( 'NONE', #42976, #3055, #38249, .T. ) ;
#35927=CARTESIAN_POINT ( 'NONE',  ( 7.699327770571627205, -78.80327297366488892, -5.126656867452202171 ) ) ;
#35941=CARTESIAN_POINT ( 'NONE',  ( 0.000000000000000000, -77.04999999999999716, -9.400000000000000355 ) ) ;
#35948=DIRECTION ( 'NONE',  ( 1.000000000000000000, 0.000000000000000000, 0.000000000000000000 ) ) ;
#35958=AXIS2_PLACEMENT_3D ( 'NONE', #13099, #45001, #40861 ) ;
#35963=CARTESIAN_POINT ( 'NONE',  ( -1.570837462060999945, -78.71707723970298787, 9.612084340777000691 ) ) ;
#35964=CARTESIAN_POINT ( 'NONE',  ( 0.000000000000000000, -74.64999999999999147, 0.000000000000000000 ) ) ;
#35970=DIRECTION ( 'NONE',  ( -1.000000000000000000, 0.000000000000000000, 0.000000000000000000 ) ) ;
#35984=CARTESIAN_POINT ( 'NONE',  ( 6.653382217586999658, -79.64551742153697944, 7.150748904218000135 ) ) ;
#35996=CARTESIAN_POINT ( 'NONE',  ( -3.907230163516999699, -77.84202411058264204, -8.882807090995999744 ) ) ;
#35997=CARTESIAN_POINT ( 'NONE',  ( 7.620730594883017517, -79.89843349061651168, 5.254643287462647194 ) ) ;
#35998=CARTESIAN_POINT ( 'NONE',  ( 5.407125718259508496, -80.28489556119939152, 9.703328807378895249 ) ) ;
#36009=CARTESIAN_POINT ( 'NONE',  ( -10.03539896543000154, -80.02094125464398644, 4.876675511606999969 ) ) ;
#36024=CARTESIAN_POINT ( 'NONE',  ( -5.062255795481000575, -77.22345684055298420, -8.064983548927001422 ) ) ;
#36031=CARTESIAN_POINT ( 'NONE',  ( -7.000000000000000000, -81.10000000285099020, 0.000000000000000000 ) ) ;
#36036=CARTESIAN_POINT ( 'NONE',  ( 10.74341457190999982, -79.16375363443799529, -2.245675826504000216 ) ) ;
#36044=CARTESIAN_POINT ( 'NONE',  ( 9.249645746724414863, -77.24371006452764732, -0.7293945652191456963 ) ) ;
#36049=CARTESIAN_POINT ( 'NONE',  ( 4.711402524194999941, -78.58337134055398110, 10.11406376844000121 ) ) ;
#36070=CARTESIAN_POINT ( 'NONE',  ( -3.495466746200742492, -78.19430050195801130, -8.564046205178371451 ) ) ;
#36076=CARTESIAN_POINT ( 'NONE',  ( -1.451214355047547366, -77.48760472878844041, 9.135408314824262632 ) ) ;
#36077=CARTESIAN_POINT ( 'NONE',  ( 10.42639159904000046, -77.22087918317399158, -2.617796444239999687 ) ) ;
#36079=CARTESIAN_POINT ( 'NONE',  ( 8.240135455977000589, -78.09617334028799007, -5.125512367919999868 ) ) ;
#36080=VECTOR ( 'NONE', #9906, 1000.000000000000000 ) ;
#36085=CONICAL_SURFACE ( 'NONE', #26624, 2.699999999213000379, 0.7853981633972997312 ) ;
#36086=DIRECTION ( 'NONE',  ( 1.000000000000000000, 0.000000000000000000, 0.000000000000000000 ) ) ;
#36087=EDGE_CURVE ( 'NONE', #15959, #50939, #52884, .T. ) ;
#36101=CARTESIAN_POINT ( 'NONE',  ( -8.648182244747999903, -80.06748455509199403, 6.853707971299000334 ) ) ;
#36115=CARTESIAN_POINT ( 'NONE',  ( 10.75000000000000000, -77.19999999999998863, -6.141891925717000695E-13 ) ) ;
#36125=CARTESIAN_POINT ( 'NONE',  ( -0.8405563561534999950, -77.00853010409947785, -9.635375415708001157 ) ) ;
#36128=CARTESIAN_POINT ( 'NONE',  ( 8.318585563179999198, -78.15655403032357640, 7.159970128962999780 ) ) ;
#36131=AXIS2_PLACEMENT_3D ( 'NONE', #21728, #49787, #45357 ) ;
#36144=ADVANCED_FACE ( 'NONE', ( #25210 ), #23166, .F. ) ;
#36151=CARTESIAN_POINT ( 'NONE',  ( -1.996894868142000012, -77.23947401164122084, 10.85801781015000067 ) ) ;
#36158=CARTESIAN_POINT ( 'NONE',  ( -2.183112477083999803, -77.60260244285699116, 9.455407409464999802 ) ) ;
#36175=CARTESIAN_POINT ( 'NONE',  ( 0.000000000000000000, -81.19999999999998863, -7.000000000000000000 ) ) ;
#36194=CARTESIAN_POINT ( 'NONE',  ( -7.562571750566999818, -77.50890875220699172, -5.786002763631000079 ) ) ;
#36211=EDGE_LOOP ( 'NONE', ( #33224, #7669, #8837, #53157 ) ) ;
#36212=ADVANCED_FACE ( 'NONE', ( #994 ), #32585, .F. ) ;
#36218=EDGE_LOOP ( 'NONE', ( #31317, #25528, #28426, #10760, #27135 ) ) ;
#36227=CARTESIAN_POINT ( 'NONE',  ( 7.705485901114815128, -78.80336997934396948, -5.117403104356717414 ) ) ;
#36228=CARTESIAN_POINT ( 'NONE',  ( 1.000000000000000000, -81.19999999999998863, -7.000000000000000000 ) ) ;
#36229=CARTESIAN_POINT ( 'NONE',  ( -9.008922265110777872, -77.62093321339025920, -2.421082990426596027 ) ) ;
#36241=VECTOR ( 'NONE', #27420, 1000.000000000000114 ) ;
#36250=CARTESIAN_POINT ( 'NONE',  ( 10.75000000000000000, -77.19999999999998863, -6.141891925717000695E-13 ) ) ;
#36261=DIRECTION ( 'NONE',  ( 0.000000000000000000, 1.000000000000000000, 0.000000000000000000 ) ) ;
#36262=CARTESIAN_POINT ( 'NONE',  ( -5.702118101738999911, -78.40441511928399621, -7.895919506952999711 ) ) ;
#36266=CARTESIAN_POINT ( 'NONE',  ( 11.00000000000000000, -78.84999999999999432, 0.000000000000000000 ) ) ;
#36270=ADVANCED_FACE ( 'NONE', ( #26214 ), #18458, .F. ) ;
#36274=LINE ( 'NONE', #54298, #25575 ) ;
#36276=CARTESIAN_POINT ( 'NONE',  ( 10.62615472113999893, -77.21722575893699059, -3.576548769619000367 ) ) ;
#36284=CARTESIAN_POINT ( 'NONE',  ( 5.411006671257999834, -79.09812462199599281, 8.131518144102999557 ) ) ;
#36294=CARTESIAN_POINT ( 'NONE',  ( 1.260641617779999946, -77.61463347755076825, 9.621927669549000584 ) ) ;
#36295=CARTESIAN_POINT ( 'NONE',  ( 8.904755119730189961, -79.87193893653522991, 2.506716701817723436 ) ) ;
#36299=CARTESIAN_POINT ( 'NONE',  ( -2.858407197967999913, -77.19999999999998863, -8.797272775729998884 ) ) ;
#36306=CARTESIAN_POINT ( 'NONE',  ( -7.229432123817375100, -80.45000000000000284, -8.035240866824315376 ) ) ;
#36315=DIRECTION ( 'NONE',  ( 0.000000000000000000, 1.000000000000000000, 0.000000000000000000 ) ) ;
#36317=CARTESIAN_POINT ( 'NONE',  ( 3.648104590558693072, -76.95000000000000284, -8.803297125097907738 ) ) ;
#36321=CARTESIAN_POINT ( 'NONE',  ( -9.055195227533998192, -78.80082360769699790, -3.586521308946000186 ) ) ;
#36325=VERTEX_POINT ( 'NONE', #25924 ) ;
#36328=CARTESIAN_POINT ( 'NONE',  ( -10.44304457033000055, -78.40526006745598409, 3.377400876517000050 ) ) ;
#36340=CARTESIAN_POINT ( 'NONE',  ( 3.325053339351000226, -78.95626297899599422, -10.53669369097999997 ) ) ;
#36344=CARTESIAN_POINT ( 'NONE',  ( 2.421167930323313566, -79.85416666666665719, 9.009247259181924150 ) ) ;
#36345=CARTESIAN_POINT ( 'NONE',  ( 5.155010784763280896, -79.53646688885500282, 9.790528303537312738 ) ) ;
#36354=CARTESIAN_POINT ( 'NONE',  ( 10.91276041655392959, -80.28723958337666033, -1.427624777354248975 ) ) ;
#36360=CARTESIAN_POINT ( 'NONE',  ( -5.840324968496969582, -78.17066989859858950, -7.173046464363928010 ) ) ;
#36367=CARTESIAN_POINT ( 'NONE',  ( 2.115181327729357630, -77.45675243142653699, 9.004852716841607929 ) ) ;
#36368=CARTESIAN_POINT ( 'NONE',  ( 10.65102452230999930, -77.70134130481397960, 2.905137941168000282 ) ) ;
#36370=CARTESIAN_POINT ( 'NONE',  ( -9.022250383429000209, -78.92046438502799788, -3.573472734901999903 ) ) ;
#36375=CARTESIAN_POINT ( 'NONE',  ( -6.898009915208000109, -79.49989681241999051, -8.491482529321999095 ) ) ;
#36398=B_SPLINE_CURVE_WITH_KNOTS ( 'NONE', 3,
 ( #15050, #56090, #37778, #33343, #33042, #51674, #2363, #18404, #51089, #10638, #54423, #15636, #24205, #20360, #46665, #13959, #15928, #47544 ),
 .UNSPECIFIED., .F., .F.,
 ( 4, 2, 2, 2, 2, 2, 2, 2, 4 ),
 ( 0.000000000000000000, 0.1250000000000000833, 0.2500000000000001665, 0.3750000000000002220, 0.5000000000000002220, 0.6250000000000002220, 0.7500000000000001110, 0.8750000000000001110, 1.000000000000000000 ),
 .UNSPECIFIED. ) ;
#36400=CARTESIAN_POINT ( 'NONE',  ( 11.00000000000000000, -79.94999999999998863, 0.000000000000000000 ) ) ;
#36413=CARTESIAN_POINT ( 'NONE',  ( 5.491552160713999875, -77.21740503984499071, 7.961786551375001686 ) ) ;
#36416=CARTESIAN_POINT ( 'NONE',  ( -5.755176823513999729, -78.26892344765445841, 9.345691860246999383 ) ) ;
#36425=VERTEX_POINT ( 'NONE', #26791 ) ;
#36426=VERTEX_POINT ( 'NONE', #7637 ) ;
#36437=EDGE_CURVE ( 'NONE', #36505, #15394, #9989, .T. ) ;
#36443=CARTESIAN_POINT ( 'NONE',  ( -5.159044788988000008, -77.28994032243799950, -8.219183903844999861 ) ) ;
#36450=AXIS2_PLACEMENT_3D ( 'NONE', #13433, #35873, #27308 ) ;
#36462=CARTESIAN_POINT ( 'NONE',  ( 8.503076353544873456, -77.20000000000000284, -6.721226585468835779 ) ) ;
#36466=CARTESIAN_POINT ( 'NONE',  ( 10.71369944335147828, -79.42916666666667425, -2.879226727952064913 ) ) ;
#36468=CARTESIAN_POINT ( 'NONE',  ( 8.655581700850000004, -79.61727500578398065, 4.491190667650000634 ) ) ;
#36476=CARTESIAN_POINT ( 'NONE',  ( 9.825879204080999685, -77.53244226292098062, 5.302575144543999919 ) ) ;
#36479=CARTESIAN_POINT ( 'NONE',  ( 8.981578277711999903, -78.79500914553598534, 2.818234580162000125 ) ) ;
#36488=ORIENTED_EDGE ( 'NONE', *, *, #19466, .T. ) ;
#36505=VERTEX_POINT ( 'NONE', #49850 ) ;
#36516=CARTESIAN_POINT ( 'NONE',  ( 0.008117082130627714665, -78.72521557527629454, -9.249909508878625175 ) ) ;
#36521=CARTESIAN_POINT ( 'NONE',  ( 9.190623734250525700, -77.83975365453363793, -1.210915399504562950 ) ) ;
#36523=AXIS2_PLACEMENT_3D ( 'NONE', #39480, #58067, #48355 ) ;
#36529=CARTESIAN_POINT ( 'NONE',  ( 6.916454804249409172, -79.99999999999998579, 6.378165265317452537 ) ) ;
#36536=CARTESIAN_POINT ( 'NONE',  ( 11.00000000000000000, -78.34999999999999432, 0.000000000000000000 ) ) ;
#36540=ADVANCED_FACE ( 'NONE', ( #279 ), #44869, .F. ) ;
#36557=CARTESIAN_POINT ( 'NONE',  ( 4.222580443737000699, -79.11071469600697981, 8.944559048890999620 ) ) ;
#36566=EDGE_LOOP ( 'NONE', ( #9250, #52265, #32433, #8768, #38764 ) ) ;
#36567=ADVANCED_FACE ( 'NONE', ( #19126 ), #13806, .T. ) ;
#36568=CARTESIAN_POINT ( 'NONE',  ( -4.763107053801999946, -77.14659090128088792, -9.977925823576001108 ) ) ;
#36572=CARTESIAN_POINT ( 'NONE',  ( -0.5483576180056000116, -79.51098439765999615, -9.751923335751000010 ) ) ;
#36579=ORIENTED_EDGE ( 'NONE', *, *, #12177, .T. ) ;
#36585=CARTESIAN_POINT ( 'NONE',  ( 9.244022517729193922, -79.85467752281239484, 0.4841345082002578848 ) ) ;
#36589=CARTESIAN_POINT ( 'NONE',  ( 7.685661446562000343, -76.94999999999998863, -5.583959896778000420 ) ) ;
#36602=ORIENTED_EDGE ( 'NONE', *, *, #7583, .F. ) ;
#36611=CARTESIAN_POINT ( 'NONE',  ( -1.553298277364999924, -78.59482872126899622, 9.504760619105999453 ) ) ;
#36612=AXIS2_PLACEMENT_3D ( 'NONE', #32537, #1573, #50583 ) ;
#36622=CARTESIAN_POINT ( 'NONE',  ( -0.6514878906251000412, -79.87018070975999251, 10.95625855609000077 ) ) ;
#36623=FACE_BOUND ( 'NONE', #8758, .T. ) ;
#36634=CARTESIAN_POINT ( 'NONE',  ( 4.065750953757999220, -79.46192535698398274, -10.27363435345999854 ) ) ;
#36638=LINE ( 'NONE', #9783, #47196 ) ;
#36639=CARTESIAN_POINT ( 'NONE',  ( -10.44320937922884518, -78.42521039652507397, 3.377454177612398745 ) ) ;
#36642=ORIENTED_EDGE ( 'NONE', *, *, #34851, .F. ) ;
#36645=ORIENTED_EDGE ( 'NONE', *, *, #35872, .F. ) ;
#36658=CARTESIAN_POINT ( 'NONE',  ( 2.071969569050668536, -77.45712744981192088, 9.014943109846830893 ) ) ;
#36659=CARTESIAN_POINT ( 'NONE',  ( 10.94195044575999987, -77.66953159614799063, -1.468969119710000104 ) ) ;
#36668=CARTESIAN_POINT ( 'NONE',  ( 10.24785796630000156, -78.20764851311697896, 3.830033060943999867 ) ) ;
#36681=CARTESIAN_POINT ( 'NONE',  ( 9.296222075829000175, -77.84175299886499033, 1.480354560350000126 ) ) ;
#36691=CARTESIAN_POINT ( 'NONE',  ( -6.405050160242000246, -78.73413188543698027, 8.912875463421000788 ) ) ;
#36701=EDGE_CURVE ( 'NONE', #26900, #36425, #13449, .T. ) ;
#36705=CARTESIAN_POINT ( 'NONE',  ( 2.309272084855999996, -76.97433654539688064, -9.392260232199999948 ) ) ;
#36711=AXIS2_PLACEMENT_3D ( 'NONE', #14736, #5312, #19474 ) ;
#36723=CARTESIAN_POINT ( 'NONE',  ( 0.000000000000000000, -80.99999999999998579, 7.000000000000000000 ) ) ;
#36726=CARTESIAN_POINT ( 'NONE',  ( 5.478502669466799091, -78.27562318616411119, -7.453347129908455493 ) ) ;
#36734=CARTESIAN_POINT ( 'NONE',  ( -9.157500079073999544, -78.68270794975798310, 3.211059275314999795 ) ) ;
#36751=CARTESIAN_POINT ( 'NONE',  ( 9.231148410301667440, -77.20000000000000284, -5.678455705185387004 ) ) ;
#36753=CARTESIAN_POINT ( 'NONE',  ( -8.796335266379976758, -78.25208333333333144, -6.760013919724066511 ) ) ;
#36755=CARTESIAN_POINT ( 'NONE',  ( -5.088691759813757095E-08, -76.94999999999998863, -9.499908983443795307 ) ) ;
#36757=CARTESIAN_POINT ( 'NONE',  ( -6.888064133618999385, -79.26660310668899001, 6.902496683615999551 ) ) ;
#36764=CARTESIAN_POINT ( 'NONE',  ( 8.063504857351000865, -77.93227818423599729, -7.723038145240000318 ) ) ;
#36769=CARTESIAN_POINT ( 'NONE',  ( 8.779834778627000347, -77.80017512602198337, 3.394951511978999914 ) ) ;
#36780=CARTESIAN_POINT ( 'NONE',  ( 10.84079038992999955, -79.61007816076597976, -1.471421101766999806 ) ) ;
#36790=CIRCLE ( 'NONE', #11363, 5.500000000000000000 ) ;
#36793=CARTESIAN_POINT ( 'NONE',  ( -7.000000000000000000, -81.19999999999998863, 0.000000000000000000 ) ) ;
#36796=ORIENTED_EDGE ( 'NONE', *, *, #53848, .F. ) ;
#36798=CARTESIAN_POINT ( 'NONE',  ( 9.583569705204123323, -78.11247223426698838, 1.526112543548083345 ) ) ;
#36799=DIRECTION ( 'NONE',  ( 0.000000000000000000, -1.000000000000000000, 0.000000000000000000 ) ) ;
#36800=DIRECTION ( 'NONE',  ( 0.000000000000000000, 1.000000000000000000, 0.000000000000000000 ) ) ;
#36805=CARTESIAN_POINT ( 'NONE',  ( 6.549831546891490497, -78.78778326711085356, -6.531473034326317872 ) ) ;
#36810=CARTESIAN_POINT ( 'NONE',  ( -9.189182874619413965, -80.14647585629263915, -6.046231220059206102 ) ) ;
#36826=CIRCLE ( 'NONE', #14191, 1.200000000000000622 ) ;
#36834=ORIENTED_EDGE ( 'NONE', *, *, #50771, .F. ) ;
#36844=CARTESIAN_POINT ( 'NONE',  ( 9.890776657308000708, -79.52153893684399577, 0.09015406917691999589 ) ) ;
#36856=CARTESIAN_POINT ( 'NONE',  ( 10.73068991439000186, -77.28110149971999476, -3.611733201485999967 ) ) ;
#36861=CARTESIAN_POINT ( 'NONE',  ( 3.366547962069000199, -79.66330989936849960, -9.168809063548000182 ) ) ;
#36869=EDGE_CURVE ( 'NONE', #51020, #17089, #41590, .T. ) ;
#36874=CARTESIAN_POINT ( 'NONE',  ( 9.250000000000000000, -79.84999999999999432, 0.000000000000000000 ) ) ;
#36889=ORIENTED_EDGE ( 'NONE', *, *, #46148, .F. ) ;
#36891=EDGE_CURVE ( 'NONE', #48925, #29378, #3158, .T. ) ;
#36898=CARTESIAN_POINT ( 'NONE',  ( 8.831426253027000683, -78.42428574649498785, -3.841760052678000026 ) ) ;
#36904=CARTESIAN_POINT ( 'NONE',  ( 7.396628201097954936, -77.90225191519014913, 5.684307536487873236 ) ) ;
#36907=CARTESIAN_POINT ( 'NONE',  ( -9.438868967565998247, -79.53307245776798595, -5.601050722391000214 ) ) ;
#36917=CARTESIAN_POINT ( 'NONE',  ( -9.250000000000000000, -77.49999999999998579, -1.203901273580999948E-14 ) ) ;
#36926=CARTESIAN_POINT ( 'NONE',  ( 10.74358412115683770, -79.18370396350707097, -2.245711267065026551 ) ) ;
#36929=ORIENTED_EDGE ( 'NONE', *, *, #28605, .T. ) ;
#36937=ADVANCED_FACE ( 'NONE', ( #53029 ), #575, .F. ) ;
#36945=CARTESIAN_POINT ( 'NONE',  ( 10.53001524630587404, -77.97857283748489010, -2.879224655733970017 ) ) ;
#36947=CARTESIAN_POINT ( 'NONE',  ( 9.240164464789534904, -77.35383050921583958, 0.4429433074386741609 ) ) ;
#36948=CARTESIAN_POINT ( 'NONE',  ( -4.789974786805000662, -78.01943839146699133, -9.946872946892002076 ) ) ;
#36957=CARTESIAN_POINT ( 'NONE',  ( 3.166366903731000271, -79.78082035574699660, 10.47195928638999973 ) ) ;
#36962=CARTESIAN_POINT ( 'NONE',  ( -11.00000000000000000, -77.19999999999998863, 5.688460190305999883E-13 ) ) ;
#36972=CARTESIAN_POINT ( 'NONE',  ( 9.086766343481999186, -78.80816318924999564, -2.458053382951000287 ) ) ;
#36975=CYLINDRICAL_SURFACE ( 'NONE', #7337, 11.00000000000000000 ) ;
#36981=CARTESIAN_POINT ( 'NONE',  ( -4.277738290159001089, -78.90268601143299065, -10.10766895494000117 ) ) ;
#36990=CARTESIAN_POINT ( 'NONE',  ( 9.101894997447999458, -78.37903382810698361, -6.639611571546000235 ) ) ;
#36995=LINE ( 'NONE', #37287, #38389 ) ;
#37004=CARTESIAN_POINT ( 'NONE',  ( -11.00000000000000000, -79.19999999999998863, 0.000000000000000000 ) ) ;
#37012=CARTESIAN_POINT ( 'NONE',  ( -3.321932689531000182, -80.44999999999998863, -10.22385755016999909 ) ) ;
#37018=CARTESIAN_POINT ( 'NONE',  ( 5.660329970366285046, -78.27756882288660734, -7.317403316748722020 ) ) ;
#37023=CARTESIAN_POINT ( 'NONE',  ( -6.000000000000000000, -81.19999999999998863, 0.000000000000000000 ) ) ;
#37026=CARTESIAN_POINT ( 'NONE',  ( 7.890274420948999001, -78.97040150846099493, -5.649267206312000411 ) ) ;
#37044=CARTESIAN_POINT ( 'NONE',  ( -10.71369944335147117, -78.22083333333330302, -2.879226727952084453 ) ) ;
#37047=CARTESIAN_POINT ( 'NONE',  ( 9.639239310942999239, -79.09126715714099021, 1.474640406829000217 ) ) ;
#37055=CARTESIAN_POINT ( 'NONE',  ( 8.142057126146999835, -77.86840244345297890, -7.798273688473000398 ) ) ;
#37094=EDGE_CURVE ( 'NONE', #11445, #47767, #53494, .T. ) ;
#37096=CARTESIAN_POINT ( 'NONE',  ( 7.931954819903705101, -78.80706091626400678, -4.759922961224686055 ) ) ;
#37100=CARTESIAN_POINT ( 'NONE',  ( -7.656495383265241372, -80.16412063804881427, -7.897723017437628279 ) ) ;
#37116=EDGE_CURVE ( 'NONE', #23736, #4408, #17246, .T. ) ;
#37118=CARTESIAN_POINT ( 'NONE',  ( -9.098371730874241337, -77.49610366954293283, -5.890886578694863651 ) ) ;
#37122=CARTESIAN_POINT ( 'NONE',  ( 10.55657102546000203, -78.57793934531359525, -3.003801718854000047 ) ) ;
#37123=DIRECTION ( 'NONE',  ( 1.000000000000000000, 0.000000000000000000, 0.000000000000000000 ) ) ;
#37132=CARTESIAN_POINT ( 'NONE',  ( -1.173259754689000234, -79.00834361351799373, -9.559114633834001395 ) ) ;
#37148=CARTESIAN_POINT ( 'NONE',  ( -10.25776238537000040, -77.96041360879199544, -4.245464761278999966 ) ) ;
#37154=CARTESIAN_POINT ( 'NONE',  ( 1.841371367509999857, -80.03054692978699336, -9.592189096167999196 ) ) ;
#37166=CARTESIAN_POINT ( 'NONE',  ( 0.9999999970599000587, -81.20000000293998710, 7.000000017349999659 ) ) ;
#37168=AXIS2_PLACEMENT_3D ( 'NONE', #38304, #55148, #50448 ) ;
#37169=CARTESIAN_POINT ( 'NONE',  ( -9.233182284105000193, -77.12377164566318299, -0.8981109299819999281 ) ) ;
#37170=EDGE_CURVE ( 'NONE', #52834, #32058, #42223, .T. ) ;
#37185=CARTESIAN_POINT ( 'NONE',  ( 7.502868599214999712, -77.08946594610628722, -5.987157122012000343 ) ) ;
#37190=CARTESIAN_POINT ( 'NONE',  ( -3.509962959857999554, -78.11162362607598197, 8.968465308258000590 ) ) ;
#37195=CYLINDRICAL_SURFACE ( 'NONE', #28534, 9.549999999999998934 ) ;
#37197=CARTESIAN_POINT ( 'NONE',  ( 9.250030457523495286, -77.86058932347035011, 1.210900974741199621 ) ) ;
#37199=CARTESIAN_POINT ( 'NONE',  ( -7.508490145779999736, -79.05550243411299505, -8.005410190140000992 ) ) ;
#37237=CARTESIAN_POINT ( 'NONE',  ( 9.045497074381291469, -77.36695256801532139, 1.937463959486106946 ) ) ;
#37238=LINE ( 'NONE', #42849, #15006 ) ;
#37239=VECTOR ( 'NONE', #25329, 1000.000000000000000 ) ;
#37242=CARTESIAN_POINT ( 'NONE',  ( -2.183112477083999803, -77.78351121986898420, 9.455407409464999802 ) ) ;
#37247=CARTESIAN_POINT ( 'NONE',  ( -10.62234821842000088, -78.90995737143398969, 2.617925641156000349 ) ) ;
#37261=CARTESIAN_POINT ( 'NONE',  ( 2.192362874646999860, -78.72289170186299145, -9.154492618432000128 ) ) ;
#37270=CARTESIAN_POINT ( 'NONE',  ( 10.55657102546000026, -78.53748540510798648, -3.003801718854000047 ) ) ;
#37282=CARTESIAN_POINT ( 'NONE',  ( 1.728979404161999911, -78.04192557611499126, 11.13281482770999986 ) ) ;
#37284=DIRECTION ( 'NONE',  ( 1.000000000000000000, 0.000000000000000000, 0.000000000000000000 ) ) ;
#37287=CARTESIAN_POINT ( 'NONE',  ( 0.000000000000000000, -77.04999999999999716, -9.400000000000000355 ) ) ;
#37289=DIRECTION ( 'NONE',  ( 0.000000000000000000, -1.000000000000000000, 0.000000000000000000 ) ) ;
#37291=ORIENTED_EDGE ( 'NONE', *, *, #5679, .F. ) ;
#37293=( NAMED_UNIT ( * ) SI_UNIT ( $, .STERADIAN. ) SOLID_ANGLE_UNIT ( ) );
#37295=CARTESIAN_POINT ( 'NONE',  ( 0.000000000000000000, -81.79999999999998295, -4.100000000000000533 ) ) ;
#37296=ORIENTED_EDGE ( 'NONE', *, *, #52241, .T. ) ;
#37297=EDGE_LOOP ( 'NONE', ( #36645, #9139, #11858, #22465 ) ) ;
#37301=ORIENTED_EDGE ( 'NONE', *, *, #51094, .F. ) ;
#37307=CARTESIAN_POINT ( 'NONE',  ( 6.544128014875892241, -78.28754515060697372, -6.537337346629323420 ) ) ;
#37317=CARTESIAN_POINT ( 'NONE',  ( -9.626984307556000431, -78.25980578023599321, 1.221426423741999834 ) ) ;
#37321=B_SPLINE_SURFACE_WITH_KNOTS ( 'NONE', 3, 3, ( 
 ( #44846, #21238, #48694, #30369, #13543, #48411, #12945, #43691, #7, #7948, #31234, #30943, #44545, #17986, #48130, #49276, #3246, #4099, #57252, #52826, #16819, #34803, #28279, #46038, #50165, #19152, #1165, #37148, #5562, #27411, #50753, #9709, #45151, #14415, #27700 ),
 ( #23572, #41586, #31534, #4987, #55160, #36276, #14706, #10298, #5854, #45445, #27113, #23860, #18284, #41876, #1453, #37440, #18579, #55456, #9129, #49582, #22994, #54868, #4703, #41005, #40713, #27989, #54300, #13837, #596, #45742, #31834, #49877, #9421, #10011, #18864 ),
 ( #41295, #36568, #14128, #23285, #878, #36856, #32414, #50459, #33590, #24455, #6441, #20035, #33870, #51628, #1744, #2609, #24743, #46621, #42758, #56619, #55757, #51911, #42469, #51045, #2322, #20318, #20604, #11471, #29442, #2036, #38023, #38604, #16178, #56046, #34157 ),
 ( #15595, #19738, #32998, #10890, #10592, #47497, #11182, #7024, #25027, #28576, #29158, #47207, #38314, #24159, #43047, #56335, #37733, #42176, #15301, #15887, #33296, #51333, #28867, #46913, #55356, #37341, #50652, #37630, #27887, #24055, #14029, #18474, #27314, #32896, #9613 ) ),
 .UNSPECIFIED., .F., .F., .F.,
 ( 4, 4 ),
 ( 4, 1, 1, 1, 1, 1, 1, 1, 1, 1, 1, 1, 1, 1, 1, 1, 1, 1, 1, 1, 1, 1, 1, 1, 1, 1, 1, 1, 1, 1, 1, 1, 4 ),
 ( -0.1387574078320000237, 1.138757407831999968 ),
 ( 0.3340109127995999905, 0.3552311533231000129, 0.3764513938467000109, 0.3976716343701999778, 0.4188918748937999759, 0.4401121154172999983, 0.4613323559408000207, 0.4825525964644000187, 0.5037728369878999857, 0.5249930775114999282, 0.5462133180349999506, 0.5674335585586000041, 0.5886537990821000266, 0.6098740396056000490, 0.6310942801291999915, 0.6523145206527000139, 0.6735347611762999565, 0.6947550016997999789, 0.7159752422233999214, 0.7371954827468999438, 0.7584157232704000773, 0.7796359637940000198, 0.8008562043175000422, 0.8220764448410999847, 0.8432966853646000072, 0.8645169258881999497, 0.8857371664116999721, 0.9069574069351999945, 0.9281776474588000481, 0.9493978879823000705, 0.9706181285059000130, 0.9918383690294000354, 1.013058609553000089 ),
 .UNSPECIFIED. ) ;
#37341=CARTESIAN_POINT ( 'NONE',  ( -9.866499134202999954, -78.07867141381099430, 5.775311262588999739 ) ) ;
#37349=CARTESIAN_POINT ( 'NONE',  ( -10.99144026735999979, -77.69704419146098928, -2.508820398717999556 ) ) ;
#37354=CARTESIAN_POINT ( 'NONE',  ( 7.588757936995927963E-07, -80.21583927563050054, -10.98470495943546688 ) ) ;
#37356=LINE ( 'NONE', #20240, #48724 ) ;
#37368=AXIS2_PLACEMENT_3D ( 'NONE', #8501, #43368, #26496 ) ;
#37381=CARTESIAN_POINT ( 'NONE',  ( -9.161389328174658786, -77.37563928610997266, -3.065743153103684726 ) ) ;
#37384=CARTESIAN_POINT ( 'NONE',  ( 9.583411031200000707, -78.01256708535665041, 1.526087275887999750 ) ) ;
#37388=CARTESIAN_POINT ( 'NONE',  ( -5.105871269591521155, -78.67859004320752092, -7.713068480137897254 ) ) ;
#37400=CARTESIAN_POINT ( 'NONE',  ( -9.549999999999998934, -80.99999999999998579, 0.000000000000000000 ) ) ;
#37411=CARTESIAN_POINT ( 'NONE',  ( -9.254388464354001087, -79.80752053325198858, 5.469807505829999528 ) ) ;
#37419=CARTESIAN_POINT ( 'NONE',  ( 8.743304200629554046, -78.32361866804367878, -3.019380310087202535 ) ) ;
#37422=CARTESIAN_POINT ( 'NONE',  ( 9.332529440374916163, -78.90131187205814456, 0.09866230578322067457 ) ) ;
#37423=CARTESIAN_POINT ( 'NONE',  ( 4.155310858692000231, -78.55356234745399036, -8.688302574878001394 ) ) ;
#37435=CARTESIAN_POINT ( 'NONE',  ( 2.500028546529174278, -77.64653440364209303, -8.986588875504750717 ) ) ;
#37440=CARTESIAN_POINT ( 'NONE',  ( -4.644564950407000126, -77.58407284559099537, -10.20464596076999975 ) ) ;
#37445=CARTESIAN_POINT ( 'NONE',  ( 1.739862777674999972, -79.19090020592499002, 9.611119481339999382 ) ) ;
#37453=CIRCLE ( 'NONE', #41211, 9.750000000000000000 ) ;
#37457=CARTESIAN_POINT ( 'NONE',  ( -1.817250558667000027, -77.00611544385418483, 9.487466121941999120 ) ) ;
#37477=CARTESIAN_POINT ( 'NONE',  ( 7.600999290758999827, -78.50955723388199203, 5.914221820906000460 ) ) ;
#37479=CARTESIAN_POINT ( 'NONE',  ( -2.769480662737825671, -77.80484845553691287, -10.72687993797706341 ) ) ;
#37485=CARTESIAN_POINT ( 'NONE',  ( -9.250231375314745819, -78.08973357792895342, 1.210876817583024678 ) ) ;
#37488=CARTESIAN_POINT ( 'NONE',  ( 3.303001513109999898, -79.13977949711097892, -10.46681410869999951 ) ) ;
#37490=CARTESIAN_POINT ( 'NONE',  ( -4.038530367108999819, -79.98972034371799111, 8.407770091669000578 ) ) ;
#37493=VERTEX_POINT ( 'NONE', #3730 ) ;
#37509=CARTESIAN_POINT ( 'NONE',  ( 2.550540064461633616, -78.59376452252105594, -10.67532501814229207 ) ) ;
#37526=CARTESIAN_POINT ( 'NONE',  ( 9.203835967791539119, -77.35804978725602155, 0.9230458045160537806 ) ) ;
#37527=CARTESIAN_POINT ( 'NONE',  ( 5.341789944771999643, -77.82526364781499240, 9.661750877468000098 ) ) ;
#37537=CARTESIAN_POINT ( 'NONE',  ( 5.365758882164000099, -78.32770896256499782, 9.658494679878000255 ) ) ;
#37538=LINE ( 'NONE', #38122, #23466 ) ;
#37542=VERTEX_POINT ( 'NONE', #55367 ) ;
#37552=CARTESIAN_POINT ( 'NONE',  ( 4.939304878001000709, -78.41022958144498034, 8.013392654152999839 ) ) ;
#37563=DIRECTION ( 'NONE',  ( 7.038562604822999888E-12, 1.000000000000000000, -4.198155382477000102E-10 ) ) ;
#37566=CARTESIAN_POINT ( 'NONE',  ( 3.176617583302000281, -79.66117957841500186, 10.50586082162000068 ) ) ;
#37578=CARTESIAN_POINT ( 'NONE',  ( 0.000000000000000000, -81.99999999999998579, 0.000000000000000000 ) ) ;
#37579=DIRECTION ( 'NONE',  ( 0.000000000000000000, 0.7071067811866525998, -0.7071067811864425456 ) ) ;
#37586=SURFACE_STYLE_USAGE ( .BOTH. , #19586 ) ;
#37594=CARTESIAN_POINT ( 'NONE',  ( 0.000000000000000000, -81.79999999999998295, 0.000000000000000000 ) ) ;
#37597=AXIS2_PLACEMENT_3D ( 'NONE', #46929, #6455, #38040 ) ;
#37601=CARTESIAN_POINT ( 'NONE',  ( 5.170697374967133442, -78.27237039058387325, -7.669726363621671261 ) ) ;
#37603=ORIENTED_EDGE ( 'NONE', *, *, #46254, .T. ) ;
#37610=CARTESIAN_POINT ( 'NONE',  ( 9.703485699160999900, -77.52078622288298959, 0.1143444355825999903 ) ) ;
#37619=CARTESIAN_POINT ( 'NONE',  ( -3.321932689531000182, -80.44999999999998863, -10.22385755016999909 ) ) ;
#37623=VECTOR ( 'NONE', #7792, 1000.000000000000000 ) ;
#37630=CARTESIAN_POINT ( 'NONE',  ( -10.56350348457000088, -78.15204083114099376, -4.372004352851999620 ) ) ;
#37631=CARTESIAN_POINT ( 'NONE',  ( 10.71369944335147828, -78.97083333333333144, 2.879226727952054254 ) ) ;
#37632=CARTESIAN_POINT ( 'NONE',  ( -6.876280931137317864, -77.17439650227632342, -6.298142934911103552 ) ) ;
#37634=CARTESIAN_POINT ( 'NONE',  ( -9.492978868049998908, -79.94958509515598166, 0.8796340255361999594 ) ) ;
#37642=CARTESIAN_POINT ( 'NONE',  ( 7.337378888528000687, -77.56100197158698961, 8.415941797739000307 ) ) ;
#37656=EDGE_LOOP ( 'NONE', ( #33582, #57694, #17775, #32628 ) ) ;
#37657=VERTEX_POINT ( 'NONE', #32614 ) ;
#37681=CARTESIAN_POINT ( 'NONE',  ( -0.1538805260929127228, -78.12626240187222493, 9.702939253146000809 ) ) ;
#37687=CARTESIAN_POINT ( 'NONE',  ( -5.072857026477922915, -78.67892529861725848, -7.734870698971506364 ) ) ;
#37691=CARTESIAN_POINT ( 'NONE',  ( -7.593646480162997925, -80.16477289014299856, -7.958079035431402382 ) ) ;
#37707=CARTESIAN_POINT ( 'NONE',  ( 7.662045806512479906, -78.13848195020216281, -7.571676706850216654 ) ) ;
#37708=CARTESIAN_POINT ( 'NONE',  ( 10.26300017817222177, -78.31922858884991001, -4.172146172881584292 ) ) ;
#37709=CARTESIAN_POINT ( 'NONE',  ( -7.022507694777002207, -79.28024820363059177, 8.434951230355999030 ) ) ;
#37714=CARTESIAN_POINT ( 'NONE',  ( 8.654766271459692462, -78.32129049133318688, -3.269801377774523399 ) ) ;
#37715=DIRECTION ( 'NONE',  ( 0.000000000000000000, 1.000000000000000000, 0.000000000000000000 ) ) ;
#37718=CARTESIAN_POINT ( 'NONE',  ( 8.831426253027000683, -78.61041000571199788, -3.841760052678000026 ) ) ;
#37722=CARTESIAN_POINT ( 'NONE',  ( 0.000000000000000000, -80.99999999999998579, 0.000000000000000000 ) ) ;
#37730=CARTESIAN_POINT ( 'NONE',  ( -8.473216720655999623, -79.62385733274298616, 7.068873142094000528 ) ) ;
#37733=CARTESIAN_POINT ( 'NONE',  ( 0.3871641813082000172, -77.74850903582299111, -11.42594107635000178 ) ) ;
#37741=CARTESIAN_POINT ( 'NONE',  ( -8.448510849392999233, -79.34862110636998977, 4.901364000006999788 ) ) ;
#37746=ORIENTED_EDGE ( 'NONE', *, *, #32159, .F. ) ;
#37754=CARTESIAN_POINT ( 'NONE',  ( 8.206391254555001069, -76.92626680923629579, -4.933833811651999746 ) ) ;
#37771=CARTESIAN_POINT ( 'NONE',  ( -0.8342061549693000622, -77.01113784520168792, -9.562582470975000248 ) ) ;
#37776=CARTESIAN_POINT ( 'NONE',  ( -1.570837462060999945, -78.65870446205198618, 9.612084340777000691 ) ) ;
#37778=CARTESIAN_POINT ( 'NONE',  ( 9.209295718512867879, -76.99427083334457222, 2.475804447281278353 ) ) ;
#37786=CARTESIAN_POINT ( 'NONE',  ( -9.505686244346000180, -79.44879539476998787, 5.486888517706000279 ) ) ;
#37787=CARTESIAN_POINT ( 'NONE',  ( -10.47809169991074896, -80.07556136232952326, 3.347707656643508223 ) ) ;
#37805=CARTESIAN_POINT ( 'NONE',  ( -9.505836260145096972, -79.40844279816811024, 5.486975110082571661 ) ) ;
#37807=ORIENTED_EDGE ( 'NONE', *, *, #1288, .F. ) ;
#37824=CARTESIAN_POINT ( 'NONE',  ( 8.229772620175682007, -77.38784508169860032, 4.222788055672235252 ) ) ;
#37825=CARTESIAN_POINT ( 'NONE',  ( 10.94195044575999987, -77.72983452181898656, -1.468969119710000104 ) ) ;
#37832=CARTESIAN_POINT ( 'NONE',  ( -0.5228656313312000092, -79.11429488387997822, -11.03650783440000005 ) ) ;
#37842=CARTESIAN_POINT ( 'NONE',  ( 0.000000000000000000, -77.19999999999998863, 0.000000000000000000 ) ) ;
#37849=CARTESIAN_POINT ( 'NONE',  ( -3.430696936678000242, -77.98387214451000204, 8.765929102848000198 ) ) ;
#37854=ORIENTED_EDGE ( 'NONE', *, *, #5679, .T. ) ;
#37859=CARTESIAN_POINT ( 'NONE',  ( 10.87588596538000019, -79.54881016108498670, -1.476184626237000197 ) ) ;
#37870=CARTESIAN_POINT ( 'NONE',  ( 8.429898053969001381, -77.87337145011899509, -7.120476661986999467 ) ) ;
#37879=CARTESIAN_POINT ( 'NONE',  ( -11.00000000000000000, -79.59999999999999432, 0.000000000000000000 ) ) ;
#37885=ORIENTED_EDGE ( 'NONE', *, *, #13316, .F. ) ;
#37893=CARTESIAN_POINT ( 'NONE',  ( 6.576607919464698249, -78.28793833107616251, -6.504691508555049850 ) ) ;
#37898=CARTESIAN_POINT ( 'NONE',  ( -8.920832483808519342, -77.57870377730691303, 2.448822063241335112 ) ) ;
#37901=CARTESIAN_POINT ( 'NONE',  ( 5.417083560473000325, -78.94197767933198406, -8.051455326762999576 ) ) ;
#37916=CARTESIAN_POINT ( 'NONE',  ( 9.499693205731109202, -80.00008708754018016, -1.997583897032410100E-06 ) ) ;
#37922=CARTESIAN_POINT ( 'NONE',  ( 11.00000000000000355, -78.96041666666668846, 1.439896632895290018 ) ) ;
#37924=CARTESIAN_POINT ( 'NONE',  ( 4.848544560051999852, -80.06104530392099150, -8.085983706936000104 ) ) ;
#37931=CARTESIAN_POINT ( 'NONE',  ( 10.78300809584000142, -77.53919858637399898, -2.444354666989000169 ) ) ;
#37935=CARTESIAN_POINT ( 'NONE',  ( 9.296222075829000175, -78.28338022121498341, 1.480354560350000126 ) ) ;
#37944=CIRCLE ( 'NONE', #16246, 1.000000000000000000 ) ;
#37961=ADVANCED_FACE ( 'NONE', ( #33431 ), #16019, .F. ) ;
#37969=CARTESIAN_POINT ( 'NONE',  ( -9.446433787353997857, -78.26838154751725085, -2.221620594898999990 ) ) ;
#37976=CARTESIAN_POINT ( 'NONE',  ( -6.510594146543013494, -78.66291057767605821, -6.570709974646258722 ) ) ;
#37978=CARTESIAN_POINT ( 'NONE',  ( -6.042415835457781270, -80.17903136551073828, -9.199162289450645957 ) ) ;
#37992=CARTESIAN_POINT ( 'NONE',  ( -8.205098860340234168, -77.89376641471295670, 7.080053407133187982 ) ) ;
#37995=CARTESIAN_POINT ( 'NONE',  ( -4.277738290159001089, -78.94313995163858522, -10.10766895494000117 ) ) ;
#37997=ORIENTED_EDGE ( 'NONE', *, *, #55680, .T. ) ;
#38000=CARTESIAN_POINT ( 'NONE',  ( 9.201707288021751197, -78.34189891696935604, -0.9444728895368803556 ) ) ;
#38004=CARTESIAN_POINT ( 'NONE',  ( -9.173272937381000247, -77.30536039296298156, 2.837265496132999942 ) ) ;
#38007=CARTESIAN_POINT ( 'NONE',  ( 8.747999954847186288, -80.26119791688729777, -6.721802296415280153 ) ) ;
#38010=EDGE_CURVE ( 'NONE', #47367, #53060, #38448, .T. ) ;
#38017=CARTESIAN_POINT ( 'NONE',  ( -10.98042387750000159, -78.81580120733299566, -1.228081885531999928 ) ) ;
#38020=DIRECTION ( 'NONE',  ( -3.675129797337999037E-09, -0.9999999999999997780, 2.168720877525999531E-08 ) ) ;
#38023=CARTESIAN_POINT ( 'NONE',  ( 2.300365334442000087, -78.19821921635399065, -11.08603795934999958 ) ) ;
#38025=ORIENTED_EDGE ( 'NONE', *, *, #2903, .T. ) ;
#38028=AXIS2_PLACEMENT_3D ( 'NONE', #4960, #53670, #4673 ) ;
#38033=CARTESIAN_POINT ( 'NONE',  ( -4.373213035511999358, -79.59836458285249705, -8.733596771889999388 ) ) ;
#38040=DIRECTION ( 'NONE',  ( 1.000000000000000000, 0.000000000000000000, 0.000000000000000000 ) ) ;
#38046=EDGE_CURVE ( 'NONE', #10899, #43630, #8429, .T. ) ;
#38050=CARTESIAN_POINT ( 'NONE',  ( 5.684557159767942736, -77.82291666666665719, 7.396918292183182864 ) ) ;
#38072=DIRECTION ( 'NONE',  ( 0.000000000000000000, 0.000000000000000000, -1.000000000000000000 ) ) ;
#38073=ORIENTED_EDGE ( 'NONE', *, *, #12471, .T. ) ;
#38078=CARTESIAN_POINT ( 'NONE',  ( -10.55666020218318124, -80.07743442317976701, 3.092866764600493479 ) ) ;
#38079=CARTESIAN_POINT ( 'NONE',  ( -9.448492440162999273, -79.59134532229998626, -1.455010287921000067 ) ) ;
#38088=AXIS2_PLACEMENT_3D ( 'NONE', #50114, #19100, #45689 ) ;
#38095=CARTESIAN_POINT ( 'NONE',  ( -0.6514981722053709845, -79.82982811315835647, 10.95643146437133097 ) ) ;
#38112=ORIENTED_EDGE ( 'NONE', *, *, #50332, .T. ) ;
#38113=CARTESIAN_POINT ( 'NONE',  ( 9.233111569183694911, -77.35500786911740079, 0.5775652420082610927 ) ) ;
#38114=DIRECTION ( 'NONE',  ( 0.7071067811864976127, -0.7071067811865975328, -1.721794132147993560E-09 ) ) ;
#38121=CARTESIAN_POINT ( 'NONE',  ( 9.366620387600999464, -79.19857194687799051, -5.860402389062000061 ) ) ;
#38122=CARTESIAN_POINT ( 'NONE',  ( -7.000000000000000000, -81.10000000285099020, -1.099999997148999986 ) ) ;
#38135=CARTESIAN_POINT ( 'NONE',  ( -9.004250860540000900, -77.10273344151168828, -2.744961831234999927 ) ) ;
#38148=CARTESIAN_POINT ( 'NONE',  ( -9.813193589766999736, -78.90680422843898612, -4.915816122623000162 ) ) ;
#38158=CARTESIAN_POINT ( 'NONE',  ( 4.019191877497999776, -79.02515797775897965, 10.52497178225999974 ) ) ;
#38173=ORIENTED_EDGE ( 'NONE', *, *, #27197, .T. ) ;
#38177=CARTESIAN_POINT ( 'NONE',  ( 7.152873968220873735, -79.94241816209181195, -6.324799438550645192 ) ) ;
#38185=CARTESIAN_POINT ( 'NONE',  ( -0.5684419807725448193, -78.22027183137143425, -9.237336331917868293 ) ) ;
#38187=EDGE_LOOP ( 'NONE', ( #25779, #10745, #57561 ) ) ;
#38193=CARTESIAN_POINT ( 'NONE',  ( 6.983565664416999219, -78.45877258413898403, -6.737990796766999857 ) ) ;
#38208=CARTESIAN_POINT ( 'NONE',  ( 11.00860450206999985, -80.25708356157298340, 1.960025359315999971 ) ) ;
#38215=CARTESIAN_POINT ( 'NONE',  ( -10.50000000000000000, -81.99999999999998579, 0.000000000000000000 ) ) ;
#38219=CARTESIAN_POINT ( 'NONE',  ( -4.746402720823999388, -79.54046787954499109, -8.268135452721999457 ) ) ;
#38221=CARTESIAN_POINT ( 'NONE',  ( 8.436594745246246418, -79.14112415376850151, 4.819671195624712468 ) ) ;
#38227=CARTESIAN_POINT ( 'NONE',  ( 7.194421757875000267, -77.68875345315298375, 8.251970588205999491 ) ) ;
#38249=CIRCLE ( 'NONE', #2453, 10.69999999999999929 ) ;
#38265=CARTESIAN_POINT ( 'NONE',  ( 7.560105429166095625, -77.04631109317882931, -6.032831105176230224 ) ) ;
#38268=CARTESIAN_POINT ( 'NONE',  ( -8.199591636648101201, -78.63841546258160520, -4.282090486464941392 ) ) ;
#38285=CARTESIAN_POINT ( 'NONE',  ( 0.4264610271018738907, -77.82239105019517922, 10.82843159672154165 ) ) ;
#38286=CARTESIAN_POINT ( 'NONE',  ( 9.632126701410999914, -79.13978643196745111, 5.261763182588000909 ) ) ;
#38293=CARTESIAN_POINT ( 'NONE',  ( 8.413103616488427861, -78.31587669965468024, -3.846938760799505808 ) ) ;
#38298=CARTESIAN_POINT ( 'NONE',  ( 9.738918081334000831, -77.58012407454400261, 0.1147619655162999963 ) ) ;
#38304=CARTESIAN_POINT ( 'NONE',  ( -7.000000000000000000, -80.99999999999998579, 0.000000000000000000 ) ) ;
#38311=CARTESIAN_POINT ( 'NONE',  ( 0.000000000000000000, -81.79999999999998295, 0.000000000000000000 ) ) ;
#38312=ORIENTED_EDGE ( 'NONE', *, *, #10786, .T. ) ;
#38314=CARTESIAN_POINT ( 'NONE',  ( -11.10670190495999954, -77.60177020116098845, 2.709833645475999919 ) ) ;
#38319=CARTESIAN_POINT ( 'NONE',  ( 9.534323188421000239, -79.25198956143150042, -1.008198710029000189 ) ) ;
#38323=EDGE_LOOP ( 'NONE', ( #4792, #16368, #26123, #54455, #51852, #12078 ) ) ;
#38327=CARTESIAN_POINT ( 'NONE',  ( 5.000000000000000000, -80.49999999999998579, 0.000000000000000000 ) ) ;
#38329=CARTESIAN_POINT ( 'NONE',  ( 8.057046250017998901, -76.82309468548459108, -4.844044839845999206 ) ) ;
#38331=CARTESIAN_POINT ( 'NONE',  ( 9.611650271896847286, -79.80833333333332291, -5.539808784079878201 ) ) ;
#38335=ADVANCED_FACE ( 'NONE', ( #57530 ), #39908, .F. ) ;
#38341=VECTOR ( 'NONE', #23318, 1000.000000000000000 ) ;
#38345=AXIS2_PLACEMENT_3D ( 'NONE', #47612, #57305, #57015 ) ;
#38353=CARTESIAN_POINT ( 'NONE',  ( 7.433005562543999467, -77.46490363863499340, -6.293657445383999516 ) ) ;
#38358=ORIENTED_EDGE ( 'NONE', *, *, #51404, .T. ) ;
#38360=CARTESIAN_POINT ( 'NONE',  ( 9.492479839331700475, -79.00604488997433350, 0.7216432697597927604 ) ) ;
#38365=CARTESIAN_POINT ( 'NONE',  ( -9.557645832987999412, -79.65522106308299044, -1.471819245595999970 ) ) ;
#38367=CARTESIAN_POINT ( 'NONE',  ( -10.71369944335147117, -78.62083333333333712, -2.879226727952084453 ) ) ;
#38374=EDGE_CURVE ( 'NONE', #54466, #54943, #46573, .T. ) ;
#38378=ADVANCED_FACE ( 'NONE', ( #8516 ), #1308, .F. ) ;
#38380=DIRECTION ( 'NONE',  ( 0.000000000000000000, -1.000000000000000000, 0.000000000000000000 ) ) ;
#38384=VERTEX_POINT ( 'NONE', #16810 ) ;
#38389=VECTOR ( 'NONE', #37579, 1000.000000000000000 ) ;
#38392=CARTESIAN_POINT ( 'NONE',  ( 9.611650271896829523, -77.49166666666666003, 5.539808784079915505 ) ) ;
#38402=CARTESIAN_POINT ( 'NONE',  ( 9.249977667285287808, -77.35017732644061539, 0.02052228013975116935 ) ) ;
#38403=CARTESIAN_POINT ( 'NONE',  ( -11.00724581733999941, -77.98431219114199564, 0.8512868710715000287 ) ) ;
#38414=CARTESIAN_POINT ( 'NONE',  ( -2.183649677207000206, -78.38389367123097884, 10.83095413486000069 ) ) ;
#38419=CARTESIAN_POINT ( 'NONE',  ( -9.705904104064821070, -77.19999999999998863, 5.072841802772233954 ) ) ;
#38421=DIRECTION ( 'NONE',  ( 1.000000000000000000, 0.000000000000000000, 0.000000000000000000 ) ) ;
#38428=CARTESIAN_POINT ( 'NONE',  ( -1.900968108529000000, -77.18800492889859299, -9.219409434742001253 ) ) ;
#38441=CARTESIAN_POINT ( 'NONE',  ( -10.65673661723999999, -78.85061951977299088, 2.626400817186000047 ) ) ;
#38448=LINE ( 'NONE', #47918, #2233 ) ;
#38450=CARTESIAN_POINT ( 'NONE',  ( 7.396918292183150001, -78.19791666666664298, -5.684557159767978263 ) ) ;
#38451=CARTESIAN_POINT ( 'NONE',  ( 4.145744906942999464, -79.33417387541800281, -10.47576887544000002 ) ) ;
#38460=ORIENTED_EDGE ( 'NONE', *, *, #24981, .T. ) ;
#38465=ORIENTED_EDGE ( 'NONE', *, *, #55726, .F. ) ;
#38468=CARTESIAN_POINT ( 'NONE',  ( 8.645097183540606522, -79.96524141418557008, -4.039558020937342064 ) ) ;
#38476=CARTESIAN_POINT ( 'NONE',  ( 5.628633445105355904, -79.32351257642946507, 7.438899466706690333 ) ) ;
#38479=CARTESIAN_POINT ( 'NONE',  ( -6.608220602749067751, -77.53848782482791080, 6.472502597521285317 ) ) ;
#38481=CARTESIAN_POINT ( 'NONE',  ( 11.00000000000000000, -79.84999999999999432, 0.000000000000000000 ) ) ;
#38482=CARTESIAN_POINT ( 'NONE',  ( 8.553489385229999797, -79.11597592151899505, 4.133741566275999979 ) ) ;
#38499=CARTESIAN_POINT ( 'NONE',  ( -11.00182790298000057, -80.03886997964798411, 2.541920722147000156 ) ) ;
#38504=EDGE_LOOP ( 'NONE', ( #15000, #32485, #8395, #19903 ) ) ;
#38510=CARTESIAN_POINT ( 'NONE',  ( -9.520759628685000919, -79.45279990477098409, 0.4955186682686999466 ) ) ;
#38512=CARTESIAN_POINT ( 'NONE',  ( 9.364915788055299117, -79.11789567091318531, 2.156547985526540145 ) ) ;
#38518=CARTESIAN_POINT ( 'NONE',  ( -6.501459582243999336, -77.88191509035799243, -8.943106734674001856 ) ) ;
#38523=CARTESIAN_POINT ( 'NONE',  ( -3.831287612370999796, -76.86181488578978360, -8.693171758988999187 ) ) ;
#38529=AXIS2_PLACEMENT_3D ( 'NONE', #4804, #49089, #26926 ) ;
#38546=ORIENTED_EDGE ( 'NONE', *, *, #8823, .T. ) ;
#38559=CARTESIAN_POINT ( 'NONE',  ( -5.122414477196733706, -78.67842178786030161, -7.702078103099229800 ) ) ;
#38578=CARTESIAN_POINT ( 'NONE',  ( -7.351123050927758307, -78.01612418245753133, -7.965508956423190234 ) ) ;
#38584=LINE ( 'NONE', #48330, #5951 ) ;
#38589=CARTESIAN_POINT ( 'NONE',  ( -9.554254755627999529, -78.38301937267999620, 1.212198840764999952 ) ) ;
#38602=VERTEX_POINT ( 'NONE', #27981 ) ;
#38604=CARTESIAN_POINT ( 'NONE',  ( 6.991733533204999240, -78.23490392501999224, -8.905552786469000281 ) ) ;
#38611=CARTESIAN_POINT ( 'NONE',  ( -0.6514213267380000172, -80.01047135062401594, 9.745581310452999801 ) ) ;
#38615=ORIENTED_EDGE ( 'NONE', *, *, #38802, .T. ) ;
#38639=CARTESIAN_POINT ( 'NONE',  ( -9.269456094077998642, -77.52182670896797845, -0.1220293046851000096 ) ) ;
#38646=FACE_OUTER_BOUND ( 'NONE', #42748, .T. ) ;
#38647=CYLINDRICAL_SURFACE ( 'NONE', #5918, 9.250000000000000000 ) ;
#38651=CARTESIAN_POINT ( 'NONE',  ( -1.763894203521005233, -79.36019707299011827, -9.362682977635801151 ) ) ;
#38652=CARTESIAN_POINT ( 'NONE',  ( 0.000000000000000000, -74.64999999999999147, 0.000000000000000000 ) ) ;
#38655=CARTESIAN_POINT ( 'NONE',  ( 1.635612940292999973, -79.21786873972098419, -9.418908357094000650 ) ) ;
#38671=CARTESIAN_POINT ( 'NONE',  ( -7.357969701303999521, -79.88385172005297363, 8.079184909054573538 ) ) ;
#38679=STYLED_ITEM ( 'NONE', ( #3966 ), #55564 ) ;
#38686=CARTESIAN_POINT ( 'NONE',  ( 6.000000000000000000, -81.99999999999998579, 0.000000000000000000 ) ) ;
#38688=CARTESIAN_POINT ( 'NONE',  ( 2.098039488145003517, -79.95716955824430272, 9.032790411606809400 ) ) ;
#38689=ORIENTED_EDGE ( 'NONE', *, *, #42061, .F. ) ;
#38690=LINE ( 'NONE', #28959, #50122 ) ;
#38693=CARTESIAN_POINT ( 'NONE',  ( 3.122028716178808061, -77.25255616389402746, -8.707463557169358381 ) ) ;
#38698=CARTESIAN_POINT ( 'NONE',  ( 0.000000000000000000, -74.64999999999999147, 0.000000000000000000 ) ) ;
#38702=CARTESIAN_POINT ( 'NONE',  ( 7.267180141948999861, -79.31094136420898622, 8.322618964701998578 ) ) ;
#38709=CARTESIAN_POINT ( 'NONE',  ( -9.309572583879614172, -77.20000000000000284, 5.728019906940674311 ) ) ;
#38721=CARTESIAN_POINT ( 'NONE',  ( -1.199999999999999956, -80.99999999999998579, -7.000000000000000000 ) ) ;
#38729=CARTESIAN_POINT ( 'NONE',  ( 6.612939829087000732, -79.69339014975298596, 8.759739992124000452 ) ) ;
#38733=DIRECTION ( 'NONE',  ( -1.000000000000000000, 0.000000000000000000, 0.000000000000000000 ) ) ;
#38736=AXIS2_PLACEMENT_3D ( 'NONE', #32029, #50070, #5977 ) ;
#38738=ADVANCED_FACE ( 'NONE', ( #25017 ), #41697, .T. ) ;
#38739=CARTESIAN_POINT ( 'NONE',  ( 10.99999999999999822, -77.96041666666667425, 1.439896632895345086 ) ) ;
#38740=CARTESIAN_POINT ( 'NONE',  ( -5.850594862776000049, -78.16198602556298169, 9.500638896661000032 ) ) ;
#38743=CARTESIAN_POINT ( 'NONE',  ( -9.309367086190000862, -77.13855160546319212, -0.1968645694141999969 ) ) ;
#38746=EDGE_CURVE ( 'NONE', #11813, #33386, #37944, .T. ) ;
#38747=ORIENTED_EDGE ( 'NONE', *, *, #46148, .T. ) ;
#38764=ORIENTED_EDGE ( 'NONE', *, *, #7840, .F. ) ;
#38766=CARTESIAN_POINT ( 'NONE',  ( -5.620083643312043797, -77.52702428364116827, 7.346969722847941142 ) ) ;
#38768=CARTESIAN_POINT ( 'NONE',  ( 10.90987126150000108, -77.07178011482669433, 1.690571823134000118 ) ) ;
#38771=CARTESIAN_POINT ( 'NONE',  ( 7.890274420948999001, -79.03070443413199087, -5.649267206312000411 ) ) ;
#38775=CARTESIAN_POINT ( 'NONE',  ( -8.744140569415000286, -80.31565346514499026, 7.086030162020000134 ) ) ;
#38785=CARTESIAN_POINT ( 'NONE',  ( 9.250225651199979637, -79.36043693044713621, 1.210484955505027882 ) ) ;
#38786=CARTESIAN_POINT ( 'NONE',  ( 8.479715450285999268, -80.18656123089598964, -7.288724056671999740 ) ) ;
#38796=B_SPLINE_CURVE_WITH_KNOTS ( 'NONE', 3,
 ( #25577, #25866, #43024, #56886 ),
 .UNSPECIFIED., .F., .F.,
 ( 4, 4 ),
 ( 0.000000000000000000, 1.000000000000000000 ),
 .UNSPECIFIED. ) ;
#38797=CARTESIAN_POINT ( 'NONE',  ( 7.830816902459000417, -79.59348277179398679, -5.626419586328999856 ) ) ;
#38802=EDGE_CURVE ( 'NONE', #29877, #52834, #30458, .T. ) ;
#38803=CARTESIAN_POINT ( 'NONE',  ( 8.796335266379992746, -77.39791666666667425, -6.760013919724047859 ) ) ;
#38805=EDGE_CURVE ( 'NONE', #52835, #49740, #53682, .T. ) ;
#38806=CARTESIAN_POINT ( 'NONE',  ( -0.008233557564672998319, -77.68199712970098858, 11.05658471417999955 ) ) ;
#38812=CARTESIAN_POINT ( 'NONE',  ( -6.294203684166999935, -77.26153958204697858, 7.343715272572999275 ) ) ;
#38814=CARTESIAN_POINT ( 'NONE',  ( -11.00000000000000000, -77.59999999999999432, 0.000000000000000000 ) ) ;
#38826=ORIENTED_EDGE ( 'NONE', *, *, #51838, .F. ) ;
#38828=ORIENTED_EDGE ( 'NONE', *, *, #1178, .T. ) ;
#38834=ORIENTED_EDGE ( 'NONE', *, *, #21089, .F. ) ;
#38844=CARTESIAN_POINT ( 'NONE',  ( -6.294306073545501867, -77.28129539589265562, 7.343834734617976423 ) ) ;
#38860=DIRECTION ( 'NONE',  ( 0.000000000000000000, 1.000000000000000000, 0.000000000000000000 ) ) ;
#38863=CONICAL_SURFACE ( 'NONE', #13406, 4.899999999795999983, 0.7853981633972997312 ) ;
#38875=CARTESIAN_POINT ( 'NONE',  ( -6.715271092063999525, -77.95666193574498948, -6.903502308617000871 ) ) ;
#38879=ORIENTED_EDGE ( 'NONE', *, *, #32753, .T. ) ;
#38881=CARTESIAN_POINT ( 'NONE',  ( -5.539808784079903070, -78.78333333333334565, -9.611650271896833075 ) ) ;
#38885=CARTESIAN_POINT ( 'NONE',  ( 3.902863791433999641, -79.21678520010797797, 10.22034591202999820 ) ) ;
#38887=CARTESIAN_POINT ( 'NONE',  ( 3.929414825497000496, -80.02429038178499354, -10.50786154751999923 ) ) ;
#38890=ORIENTED_EDGE ( 'NONE', *, *, #58377, .T. ) ;
#38893=AXIS2_PLACEMENT_3D ( 'NONE', #38652, #21511, #12930 ) ;
#38895=CARTESIAN_POINT ( 'NONE',  ( -4.465297566879000257, -80.04294400888201722, 8.686876450551999085 ) ) ;
#38902=CONICAL_SURFACE ( 'NONE', #5913, 9.649999999948999374, 0.7853981633972997312 ) ;
#38921=CARTESIAN_POINT ( 'NONE',  ( -9.252372813388998196, -77.46665409050798701, -1.135340161459000186 ) ) ;
#38923=AXIS2_PLACEMENT_3D ( 'NONE', #5597, #23609, #10049 ) ;
#38927=CARTESIAN_POINT ( 'NONE',  ( 0.8649477812003000254, -78.40288999989098784, -9.701111330267998767 ) ) ;
#38936=CARTESIAN_POINT ( 'NONE',  ( 4.657751049633202634, -79.41546676809356597, -8.372025729518147941 ) ) ;
#38937=CARTESIAN_POINT ( 'NONE',  ( -5.350956159761850017, -79.99999999999998579, -7.703458012427442547 ) ) ;
#38940=CARTESIAN_POINT ( 'NONE',  ( -0.09809059825999000282, -79.83113977864098842, -9.780255580327999354 ) ) ;
#38942=CARTESIAN_POINT ( 'NONE',  ( 5.539808784079905735, -78.76666666666666572, -9.611650271896829523 ) ) ;
#38959=B_SPLINE_CURVE_WITH_KNOTS ( 'NONE', 3,
 ( #33895, #57212, #11775, #16779, #48092, #28894, #47804, #7334, #24477, #25336, #42782, #20910, #38050, #47523, #20340, #16491, #11494, #16204 ),
 .UNSPECIFIED., .F., .F.,
 ( 4, 2, 2, 2, 2, 2, 2, 2, 4 ),
 ( 0.000000000000000000, 0.1250000000000000555, 0.2500000000000001110, 0.3750000000000001665, 0.5000000000000001110, 0.6250000000000001110, 0.7500000000000002220, 0.8750000000000001110, 1.000000000000000000 ),
 .UNSPECIFIED. ) ;
#38960=CARTESIAN_POINT ( 'NONE',  ( 6.653382217586999658, -79.52491157019498758, 7.150748904218000135 ) ) ;
#38981=CARTESIAN_POINT ( 'NONE',  ( 6.788068531828999497, -79.94435522376399206, 8.991721824839000732 ) ) ;
#38982=CARTESIAN_POINT ( 'NONE',  ( 7.215423847483414477, -77.29618573409882742, -5.793044792516142572 ) ) ;
#38989=DIRECTION ( 'NONE',  ( 0.000000000000000000, 0.000000000000000000, -1.000000000000000000 ) ) ;
#38994=CARTESIAN_POINT ( 'NONE',  ( 7.338671297540000360, -79.37481710499199039, 8.404493039061998516 ) ) ;
#39009=CARTESIAN_POINT ( 'NONE',  ( -3.470329948268000120, -78.04774788529299201, 8.867197205552999506 ) ) ;
#39020=CARTESIAN_POINT ( 'NONE',  ( -4.985523414424999800, -78.45732655911598386, -9.777963635945001286 ) ) ;
#39029=CARTESIAN_POINT ( 'NONE',  ( 9.250000000000000000, -78.24999999999998579, -1.152201742116999973E-14 ) ) ;
#39031=CARTESIAN_POINT ( 'NONE',  ( 11.02792952375000013, -78.91278856042799816, -2.305147454016000186 ) ) ;
#39045=ORIENTED_EDGE ( 'NONE', *, *, #30539, .F. ) ;
#39049=CARTESIAN_POINT ( 'NONE',  ( 0.5449807741670494865, -78.22973173042375095, -9.235034757777352610 ) ) ;
#39053=ORIENTED_EDGE ( 'NONE', *, *, #48256, .F. ) ;
#39054=CARTESIAN_POINT ( 'NONE',  ( -6.550240698926310223, -77.53778409855667064, 6.531065114973362284 ) ) ;
#39057=CARTESIAN_POINT ( 'NONE',  ( -0.5548610165507998904, -77.95059892722998995, -9.688283574444998436 ) ) ;
#39061=CARTESIAN_POINT ( 'NONE',  ( 1.791008777272000030, -80.29243406013898721, 11.11143388882000060 ) ) ;
#39077=CARTESIAN_POINT ( 'NONE',  ( -11.02922838689999985, -80.07413114498598361, -2.420755946928999869 ) ) ;
#39089=CARTESIAN_POINT ( 'NONE',  ( -3.862434228255000157, -79.36513192999699129, 8.716192152569998797 ) ) ;
#39092=DIRECTION ( 'NONE',  ( 0.000000000000000000, 0.000000000000000000, -1.000000000000000000 ) ) ;
#39095=CARTESIAN_POINT ( 'NONE',  ( -7.973554211391000734, -77.36784033438198094, -7.659671442301999811 ) ) ;
#39104=CARTESIAN_POINT ( 'NONE',  ( 5.539808784079867543, -77.43333333333333712, 9.611650271896852615 ) ) ;
#39109=CIRCLE ( 'NONE', #23054, 9.549999999999998934 ) ;
#39125=CARTESIAN_POINT ( 'NONE',  ( 8.082524092276891281, -79.70833333333332860, -4.658475568430806568 ) ) ;
#39134=CARTESIAN_POINT ( 'NONE',  ( -11.00000000000000711, -78.68958333333334565, 1.439896632895276696 ) ) ;
#39150=VECTOR ( 'NONE', #29338, 1000.000000000000000 ) ;
#39156=CARTESIAN_POINT ( 'NONE',  ( -10.13785388426000011, -78.34083892477998745, -4.205702700205000255 ) ) ;
#39164=CARTESIAN_POINT ( 'NONE',  ( -9.275907895452998986, -77.87139044835899426, 2.590510119660999866 ) ) ;
#39169=CARTESIAN_POINT ( 'NONE',  ( 4.601781879248937557, -78.93432654680742644, 8.115879808169474074 ) ) ;
#39172=CARTESIAN_POINT ( 'NONE',  ( -8.032634178075001685, -78.43019927879299757, -7.427287829177999789 ) ) ;
#39175=CARTESIAN_POINT ( 'NONE',  ( 1.785229341567000194, -80.23309620847798840, 11.07557821988999969 ) ) ;
#39181=CARTESIAN_POINT ( 'NONE',  ( 9.523132023602000729, -80.50917187374454898, 1.108936319727999997 ) ) ;
#39188=EDGE_CURVE ( 'NONE', #28511, #30828, #51837, .T. ) ;
#39194=CARTESIAN_POINT ( 'NONE',  ( 9.074254517363083750, -78.83453198432620468, -1.794298757601813010 ) ) ;
#39199=CARTESIAN_POINT ( 'NONE',  ( -11.00000000000000000, -78.09999999999999432, 2.733298954964999989E-14 ) ) ;
#39202=ADVANCED_FACE ( 'NONE', ( #42390 ), #38863, .T. ) ;
#39205=AXIS2_PLACEMENT_3D ( 'NONE', #9098, #50431, #32387 ) ;
#39224=EDGE_CURVE ( 'NONE', #18080, #11813, #23783, .T. ) ;
#39225=CARTESIAN_POINT ( 'NONE',  ( -5.860463241014358005, -79.17777220148535378, 7.502936674103677817 ) ) ;
#39226=CARTESIAN_POINT ( 'NONE',  ( -7.566790551998485270, -80.00000000000000000, -5.513831221825833850 ) ) ;
#39229=CARTESIAN_POINT ( 'NONE',  ( -8.038032936864000888, -79.82032020290799323, -5.764166645736000127 ) ) ;
#39255=CARTESIAN_POINT ( 'NONE',  ( 8.796335266379964324, -77.50208333333333144, 6.760013919724087827 ) ) ;
#39264=CARTESIAN_POINT ( 'NONE',  ( -0.7277978613523643503, -79.98136350393239979, 9.221261735625438050 ) ) ;
#39267=CARTESIAN_POINT ( 'NONE',  ( 10.71485332735033502, -80.17911206518367351, -2.929766398920109705 ) ) ;
#39269=CARTESIAN_POINT ( 'NONE',  ( -0.6687410688009000070, -80.00053993242899253, 11.24641019779000040 ) ) ;
#39270=CARTESIAN_POINT ( 'NONE',  ( 9.249996844504634552, -77.35002626973081874, 0.002854433395025519210 ) ) ;
#39276=FACE_OUTER_BOUND ( 'NONE', #49078, .T. ) ;
#39277=CARTESIAN_POINT ( 'NONE',  ( -2.421270742014151267, -77.70429338144477072, -9.009162903448457271 ) ) ;
#39279=CARTESIAN_POINT ( 'NONE',  ( 1.000000000000000000, -81.99999999999998579, 7.000000000000000000 ) ) ;
#39280=CARTESIAN_POINT ( 'NONE',  ( -0.6558374186847000242, -79.87278845086298418, 11.02940581592999969 ) ) ;
#39295=CARTESIAN_POINT ( 'NONE',  ( -2.142155038640999987, -77.53611896097199008, 9.278014228403000274 ) ) ;
#39308=CARTESIAN_POINT ( 'NONE',  ( 9.981840466370998755, -78.65397303944499185, 4.563647388395000171 ) ) ;
#39317=CARTESIAN_POINT ( 'NONE',  ( -5.539808784079931492, -78.11666666666666003, 9.611650271896815312 ) ) ;
#39320=CARTESIAN_POINT ( 'NONE',  ( 10.48730647577000141, -77.96533954523499688, -3.808884262352000061 ) ) ;
#39335=CARTESIAN_POINT ( 'NONE',  ( -5.320285352961153791, -79.67214536383268353, 7.903715897855382089 ) ) ;
#39343=CARTESIAN_POINT ( 'NONE',  ( -1.173906744531483248, -78.21502352218460885, -9.176430860882623719 ) ) ;
#39347=CARTESIAN_POINT ( 'NONE',  ( -4.496256502423060297, -77.51547528653394181, 8.084058354872142971 ) ) ;
#39352=CARTESIAN_POINT ( 'NONE',  ( 2.867548251969000095, -77.97902275635898661, -9.270807752789000489 ) ) ;
#39354=CARTESIAN_POINT ( 'NONE',  ( -9.250000000000000000, -77.49999999999998579, -1.203901273580999948E-14 ) ) ;
#39356=CARTESIAN_POINT ( 'NONE',  ( -10.49924843836999955, -80.33887287015198808, -4.054558598941000014 ) ) ;
#39367=CARTESIAN_POINT ( 'NONE',  ( 5.684123266893727155, -78.42295138177613012, 7.396499574309489233 ) ) ;
#39370=DIRECTION ( 'NONE',  ( -0.7071067811865474617, -0.7071067811865474617, 3.205717710189212192E-10 ) ) ;
#39374=CARTESIAN_POINT ( 'NONE',  ( -8.027667713925865201, -79.64209375582814232, -4.635885087717896091 ) ) ;
#39383=CARTESIAN_POINT ( 'NONE',  ( 1.621664633118000021, -80.15957412722899278, -9.284183544346999994 ) ) ;
#39385=CARTESIAN_POINT ( 'NONE',  ( 9.363982905857531236, -77.19999999999997442, 5.400558314209766841 ) ) ;
#39387=CARTESIAN_POINT ( 'NONE',  ( 0.000000000000000000, -80.49999999999998579, -10.69999999999999929 ) ) ;
#39396=CARTESIAN_POINT ( 'NONE',  ( 9.611650271896820641, -77.39166666666666572, 5.539808784079911952 ) ) ;
#39405=CARTESIAN_POINT ( 'NONE',  ( 4.100000000000000533, -78.69999999999998863, 0.000000000000000000 ) ) ;
#39409=FILL_AREA_STYLE_COLOUR ( '', #5693 ) ;
#39410=ORIENTED_EDGE ( 'NONE', *, *, #17071, .F. ) ;
#39425=CARTESIAN_POINT ( 'NONE',  ( -9.312499999988999022, -77.13750000001088836, -2.050180145195999796E-09 ) ) ;
#39426=CARTESIAN_POINT ( 'NONE',  ( -7.707166124622999881, -77.30197135713177659, -5.896629607976000109 ) ) ;
#39432=EDGE_CURVE ( 'NONE', #46115, #1066, #20953, .T. ) ;
#39434=CARTESIAN_POINT ( 'NONE',  ( -10.29678529194292658, -80.12898668796422896, -3.869235002584780148 ) ) ;
#39450=AXIS2_PLACEMENT_3D ( 'NONE', #22654, #9663, #3554 ) ;
#39458=CARTESIAN_POINT ( 'NONE',  ( -8.614692902062000002, -77.35976152403699757, 3.831263898871999807 ) ) ;
#39464=CARTESIAN_POINT ( 'NONE',  ( 8.931020339874743641, -78.87206237794539732, 2.484699444477077357 ) ) ;
#39468=CARTESIAN_POINT ( 'NONE',  ( -10.87240354821999944, -78.87967694811598562, -1.216000584195999767 ) ) ;
#39471=ORIENTED_EDGE ( 'NONE', *, *, #55726, .T. ) ;
#39480=CARTESIAN_POINT ( 'NONE',  ( 0.000000000000000000, -74.64999999999999147, 0.000000000000000000 ) ) ;
#39481=B_SPLINE_CURVE_WITH_KNOTS ( 'NONE', 3,
 ( #25104, #43704, #16258, #25963, #34523, #12396, #51991, #2688, #48145, #7676, #25677, #7388, #3260, #39255, #38392, #43987, #20681, #39547 ),
 .UNSPECIFIED., .F., .F.,
 ( 4, 2, 2, 2, 2, 2, 2, 2, 4 ),
 ( 0.000000000000000000, 0.1250000000000000278, 0.2500000000000000000, 0.3750000000000001110, 0.5000000000000001110, 0.6250000000000001110, 0.7500000000000002220, 0.8750000000000001110, 1.000000000000000000 ),
 .UNSPECIFIED. ) ;
#39486=CIRCLE ( 'NONE', #37597, 5.000000000000000000 ) ;
#39491=CARTESIAN_POINT ( 'NONE',  ( 8.700421281190083178, -78.82251712223430218, -3.142473759474660344 ) ) ;
#39502=CARTESIAN_POINT ( 'NONE',  ( -9.376541175504000236, -77.45795096818498848, -0.1234390441450999854 ) ) ;
#39507=CARTESIAN_POINT ( 'NONE',  ( 0.000000000000000000, -77.04999999999999716, 0.000000000000000000 ) ) ;
#39510=CYLINDRICAL_SURFACE ( 'NONE', #25943, 1.000000000000000000 ) ;
#39516=CARTESIAN_POINT ( 'NONE',  ( 3.573639641522492028, -79.09450849937717010, 8.866719865068596107 ) ) ;
#39518=CARTESIAN_POINT ( 'NONE',  ( 1.439896632895286466, -78.96458333333333712, 11.00000000000000711 ) ) ;
#39520=CARTESIAN_POINT ( 'NONE',  ( -5.407072851296999438, -80.19379678548699530, 7.853270924851000423 ) ) ;
#39538=CARTESIAN_POINT ( 'NONE',  ( -0.5483576180056000116, -79.45068147198898600, -9.751923335751000010 ) ) ;
#39547=CARTESIAN_POINT ( 'NONE',  ( 11.00000000000000000, -77.44999999999998863, 0.000000000000000000 ) ) ;
#39555=CARTESIAN_POINT ( 'NONE',  ( 3.434537346384257006, -79.94481355672635914, 8.588818010512337509 ) ) ;
#39558=CARTESIAN_POINT ( 'NONE',  ( -11.07910306079999962, -79.63533932610398836, -2.045094064781999954 ) ) ;
#39559=CARTESIAN_POINT ( 'NONE',  ( 4.243585900913456221, -77.26294495438891374, -8.219156677414845902 ) ) ;
#39562=VECTOR ( 'NONE', #51181, 1000.000000000000000 ) ;
#39567=DIRECTION ( 'NONE',  ( 0.000000000000000000, -1.000000000000000000, 0.000000000000000000 ) ) ;
#39570=CARTESIAN_POINT ( 'NONE',  ( -4.428614322242999890, -79.90088080519498703, 10.12250943391000035 ) ) ;
#39576=CARTESIAN_POINT ( 'NONE',  ( -7.667248634474823632, -77.19999999999998863, 7.744282795875710335 ) ) ;
#39578=CARTESIAN_POINT ( 'NONE',  ( 9.250000000000000000, -79.25028042812365925, 0.03259666451019458538 ) ) ;
#39584=CARTESIAN_POINT ( 'NONE',  ( 2.243017272178000177, -78.85064318342999456, -9.366006557871001448 ) ) ;
#39595=CARTESIAN_POINT ( 'NONE',  ( -10.13785388426000011, -78.46144477612099877, -4.205702700205000255 ) ) ;
#39599=CARTESIAN_POINT ( 'NONE',  ( -4.100000000000000533, -81.79999999999998295, 0.000000000000000000 ) ) ;
#39603=CARTESIAN_POINT ( 'NONE',  ( 11.00000000000000355, -77.83958333333332291, -1.439896632895299566 ) ) ;
#39604=CARTESIAN_POINT ( 'NONE',  ( -9.242272388666000538, -78.69574075788399625, 6.250760013846000440 ) ) ;
#39619=CARTESIAN_POINT ( 'NONE',  ( 7.345645686283435616, -79.55621302496926717, 6.245313084360852862 ) ) ;
#39624=CARTESIAN_POINT ( 'NONE',  ( -7.666962656759157113, -78.14788324491564708, -5.230267631833246611 ) ) ;
#39626=ADVANCED_FACE ( 'NONE', ( #40412 ), #37321, .F. ) ;
#39630=CARTESIAN_POINT ( 'NONE',  ( -7.080981860525860760, -77.54444738242287372, 5.951650271570930073 ) ) ;
#39631=CARTESIAN_POINT ( 'NONE',  ( -7.062685404271999978, -77.73978399679897677, 8.485436034813998774 ) ) ;
#39633=CARTESIAN_POINT ( 'NONE',  ( -8.680270256945998852, -77.23654793159298038, 3.860428508128000313 ) ) ;
#39637=CARTESIAN_POINT ( 'NONE',  ( -7.179058446792000225, -80.00010590276899336, -8.667882172381000672 ) ) ;
#39660=CARTESIAN_POINT ( 'NONE',  ( 0.000000000000000000, -80.19999999999998863, 0.000000000000000000 ) ) ;
#39664=CARTESIAN_POINT ( 'NONE',  ( 5.007692372854583240, -77.26250000000000284, -9.832060106187633153 ) ) ;
#39668=FACE_OUTER_BOUND ( 'NONE', #36566, .T. ) ;
#39689=ORIENTED_EDGE ( 'NONE', *, *, #40805, .F. ) ;
#39690=SURFACE_SIDE_STYLE ('',( #22263 ) ) ;
#39698=VERTEX_POINT ( 'NONE', #36755 ) ;
#39699=CARTESIAN_POINT ( 'NONE',  ( 2.604371601988999529, -77.49395168096407360, -10.72853197743999942 ) ) ;
#39701=EDGE_CURVE ( 'NONE', #21244, #29877, #6047, .T. ) ;
#39702=ORIENTED_EDGE ( 'NONE', *, *, #410, .T. ) ;
#39722=CARTESIAN_POINT ( 'NONE',  ( 10.73701163424265026, -77.19999999999998863, -0.8148447674452932166 ) ) ;
#39725=CARTESIAN_POINT ( 'NONE',  ( 5.539808784079907511, -79.36666666666666003, -9.611650271896827746 ) ) ;
#39739=CARTESIAN_POINT ( 'NONE',  ( 7.350012343602999820, -77.58715215706898505, -6.223385617129999936 ) ) ;
#39745=CARTESIAN_POINT ( 'NONE',  ( 10.71369944335146229, -78.92916666666664582, -2.879226727952112874 ) ) ;
#39749=CARTESIAN_POINT ( 'NONE',  ( -10.76843015134999959, -79.79903360897698406, 1.073136842994000029 ) ) ;
#39751=CARTESIAN_POINT ( 'NONE',  ( -7.226987988700000365, -79.87689231032499038, -8.725751546883000032 ) ) ;
#39756=CYLINDRICAL_SURFACE ( 'NONE', #2179, 11.00000000000000000 ) ;
#39757=CARTESIAN_POINT ( 'NONE',  ( -2.217000330786000450, -79.64323432020552218, 9.512392227823999846 ) ) ;
#39764=AXIS2_PLACEMENT_3D ( 'NONE', #38311, #1741, #51041 ) ;
#39776=DIRECTION ( 'NONE',  ( -0.7071067811864980568, 0.7071067811865969777, 1.168837541411996137E-09 ) ) ;
#39777=CARTESIAN_POINT ( 'NONE',  ( -1.439896632895359962, -77.98541666666666572, 10.99999999999999645 ) ) ;
#39780=DIRECTION ( 'NONE',  ( 0.000000000000000000, 1.000000000000000000, 0.000000000000000000 ) ) ;
#39783=CARTESIAN_POINT ( 'NONE',  ( -9.183761103090999356, -77.50442046432299037, 1.919071004230999966 ) ) ;
#39800=CARTESIAN_POINT ( 'NONE',  ( 9.611650271896820641, -78.89166666666666572, 5.539808784079911952 ) ) ;
#39803=CARTESIAN_POINT ( 'NONE',  ( 9.494251020668999175, -78.90826789792399154, 1.836410959852999847 ) ) ;
#39815=FACE_OUTER_BOUND ( 'NONE', #40021, .T. ) ;
#39822=CARTESIAN_POINT ( 'NONE',  ( -8.448510849392999233, -79.22801525502798370, 4.901364000006999788 ) ) ;
#39824=ORIENTED_EDGE ( 'NONE', *, *, #31373, .T. ) ;
#39831=CARTESIAN_POINT ( 'NONE',  ( -3.536740297498699448, -78.25459137991194325, 9.036885296280029678 ) ) ;
#39838=CARTESIAN_POINT ( 'NONE',  ( 3.524287703716790343, -79.94398289640221833, 8.552247391394926623 ) ) ;
#39839=DIRECTION ( 'NONE',  ( -1.000000000000000000, 0.000000000000000000, 0.000000000000000000 ) ) ;
#39841=CARTESIAN_POINT ( 'NONE',  ( -6.574673376928999780, -79.04539988511800175, 9.148912741538998361 ) ) ;
#39851=CARTESIAN_POINT ( 'NONE',  ( 5.418544735220999442, -78.39158470334899675, 9.753510481391998610 ) ) ;
#39863=CARTESIAN_POINT ( 'NONE',  ( 0.000000000000000000, -75.10000000032299283, -4.199999999676998996 ) ) ;
#39864=CIRCLE ( 'NONE', #38028, 1.200000000000000622 ) ;
#39868=CARTESIAN_POINT ( 'NONE',  ( 1.459128634122999868, -77.28030449881099173, -9.409639786240999726 ) ) ;
#39873=ADVANCED_FACE ( 'NONE', ( #56522 ), #38902, .F. ) ;
#39879=CARTESIAN_POINT ( 'NONE',  ( -9.871730464199000465, -79.89415484708798942, 4.797141237513000256 ) ) ;
#39886=CARTESIAN_POINT ( 'NONE',  ( -4.211014631457025814, -77.41241489099887474, 8.267936520958334867 ) ) ;
#39887=DIRECTION ( 'NONE',  ( 0.000000000000000000, -1.000000000000000000, 0.000000000000000000 ) ) ;
#39888=CARTESIAN_POINT ( 'NONE',  ( 11.03731426084000056, -79.00475665554398574, 1.633797283747999929 ) ) ;
#39890=CIRCLE ( 'NONE', #2211, 2.600000000000000089 ) ;
#39895=CARTESIAN_POINT ( 'NONE',  ( 8.018769647075153273, -79.51052682219849999, 7.624166446277075515 ) ) ;
#39902=ORIENTED_EDGE ( 'NONE', *, *, #23579, .F. ) ;
#39903=CARTESIAN_POINT ( 'NONE',  ( -6.452442768351031255, -79.68423335831413112, 7.009317820372825913 ) ) ;
#39908=CONICAL_SURFACE ( 'NONE', #35174, 1.099999997148999986, 0.7853981633972997312 ) ;
#39910=CARTESIAN_POINT ( 'NONE',  ( -8.666955468490126435, -78.12913193041232773, -3.288494062500119774 ) ) ;
#39915=CARTESIAN_POINT ( 'NONE',  ( -1.459284021221519234, -77.48767362326580610, 9.134122967561379980 ) ) ;
#39916=CARTESIAN_POINT ( 'NONE',  ( 6.574300740938999077, -77.48530632747599611, -8.869200617850999890 ) ) ;
#39918=CARTESIAN_POINT ( 'NONE',  ( 0.8618009059429999619, -78.52253077722298258, -9.665816497589000633 ) ) ;
#39923=CARTESIAN_POINT ( 'NONE',  ( 8.693423296916000353, -80.18569232445499040, -7.148151291522000683 ) ) ;
#39926=CARTESIAN_POINT ( 'NONE',  ( -2.421167930323333106, -78.60416666666664298, -9.009247259181917045 ) ) ;
#39935=CARTESIAN_POINT ( 'NONE',  ( -9.660486042390999728, -80.07923827687199037, 5.576357409276999633 ) ) ;
#39936=B_SPLINE_CURVE_WITH_KNOTS ( 'NONE', 3,
 ( #21490, #31195, #16782, #12909, #30624, #13200, #34763, #48373, #21198, #39777, #48942, #57791, #40374, #44506, #8786, #35043, #58381, #39199 ),
 .UNSPECIFIED., .F., .F.,
 ( 4, 2, 2, 2, 2, 2, 2, 2, 4 ),
 ( 0.000000000000000000, 0.1249999999999999445, 0.2499999999999998890, 0.3749999999999999445, 0.5000000000000000000, 0.6250000000000000000, 0.7500000000000001110, 0.8750000000000000000, 1.000000000000000000 ),
 .UNSPECIFIED. ) ;
#39944=CIRCLE ( 'NONE', #47530, 1.000000000000000000 ) ;
#39945=CARTESIAN_POINT ( 'NONE',  ( 10.61050599188999932, -77.92876026662598576, -2.901234667509999809 ) ) ;
#39950=CARTESIAN_POINT ( 'NONE',  ( 7.236935317891325603, -77.20000000000000284, 8.029755504972245106 ) ) ;
#39963=CARTESIAN_POINT ( 'NONE',  ( -0.5065222552852000071, -77.20932084810999640, 9.658707080791000266 ) ) ;
#39978=ORIENTED_EDGE ( 'NONE', *, *, #12177, .F. ) ;
#39987=ORIENTED_EDGE ( 'NONE', *, *, #39432, .T. ) ;
#39988=CARTESIAN_POINT ( 'NONE',  ( -9.808193611224998776, -77.81204876761717060, 5.067887917229000116 ) ) ;
#39995=CARTESIAN_POINT ( 'NONE',  ( 4.545264886168000729, -77.54575478459899784, 8.573871732259998879 ) ) ;
#40001=CARTESIAN_POINT ( 'NONE',  ( -9.130570360603488922, -78.61295919940000942, -1.481171073185931109 ) ) ;
#40013=CARTESIAN_POINT ( 'NONE',  ( 11.00000000000000000, -77.44999999999998863, 0.000000000000000000 ) ) ;
#40021=EDGE_LOOP ( 'NONE', ( #2533, #7791, #17539, #57089, #7156, #57260 ) ) ;
#40028=CARTESIAN_POINT ( 'NONE',  ( -1.922928979007999750, -77.56575641046499925, -9.325916353809999393 ) ) ;
#40034=CARTESIAN_POINT ( 'NONE',  ( 1.157617308350565644, -78.96545863123837705, 9.256449997036533262 ) ) ;
#40036=VERTEX_POINT ( 'NONE', #26573 ) ;
#40040=CARTESIAN_POINT ( 'NONE',  ( 10.70231528814999855, -80.02182239623499527, 4.045645928379999923 ) ) ;
#40055=DIRECTION ( 'NONE',  ( 0.000000000000000000, -1.000000000000000000, 0.000000000000000000 ) ) ;
#40061=CARTESIAN_POINT ( 'NONE',  ( 8.550487401031416468, -78.81900159872047595, -3.528449567620169702 ) ) ;
#40067=CARTESIAN_POINT ( 'NONE',  ( 0.000000000000000000, -81.99999999999998579, -7.000000000000000000 ) ) ;
#40070=CARTESIAN_POINT ( 'NONE',  ( -2.858407197967999913, -79.99999999999998579, 8.797272775729998884 ) ) ;
#40097=CARTESIAN_POINT ( 'NONE',  ( 9.078688998878000405, -79.10553623779898658, 3.126726393672000004 ) ) ;
#40099=CARTESIAN_POINT ( 'NONE',  ( -2.865983266988000100, -79.30827256302897865, -9.351425617539000257 ) ) ;
#40113=ORIENTED_EDGE ( 'NONE', *, *, #43777, .T. ) ;
#40117=CARTESIAN_POINT ( 'NONE',  ( -0.5483576180056000116, -79.39037854631799007, -9.751923335751000010 ) ) ;
#40125=ADVANCED_FACE ( 'NONE', ( #18039 ), #37195, .F. ) ;
#40126=CARTESIAN_POINT ( 'NONE',  ( -8.073593340907574856, -78.39671052555694075, -5.384321531606748756 ) ) ;
#40135=CARTESIAN_POINT ( 'NONE',  ( 6.953009658842218776, -79.90740165580891130, 6.100783007042114292 ) ) ;
#40137=ORIENTED_EDGE ( 'NONE', *, *, #36087, .F. ) ;
#40138=CARTESIAN_POINT ( 'NONE',  ( 9.887211716164999942, -79.41060049144299171, 5.401109038458000278 ) ) ;
#40146=CARTESIAN_POINT ( 'NONE',  ( 10.45148855949000044, -78.33539999468298731, 3.906137931512999817 ) ) ;
#40151=B_SPLINE_CURVE_WITH_KNOTS ( 'NONE', 3,
 ( #49933, #9477, #33642, #56100, #15645, #24213, #47256, #2088, #20086, #56386, #15058, #10943, #33052, #51100, #38078, #43103, #55511, #11802, #51682, #37787, #42520, #47552, #2373, #10651, #25079, #15936, #11520, #11230, #29209, #6788 ),
 .UNSPECIFIED., .F., .F.,
 ( 4, 2, 1, 1, 2, 2, 1, 2, 2, 2, 1, 1, 2, 2, 1, 2, 2, 4 ),
 ( 0.6954909650194412984, 0.7335545943920098733, 0.7430705017351519892, 0.7478284554067230472, 0.7490179438246158394, 0.7502074322425086317, 0.7525864090782941052, 0.7716182237645784481, 0.8477454825097158198, 0.8667772971960001627, 0.8715352508675713317, 0.8739142277033569162, 0.8745089719123033678, 0.8751037161212498194, 0.8762932045391426117, 0.8858091118822855048, 0.9238727412548570772, 1.000000000000000000 ),
 .UNSPECIFIED. ) ;
#40172=CARTESIAN_POINT ( 'NONE',  ( 9.233664981878000333, -79.72560072109197904, 5.933249305785000871 ) ) ;
#40178=ORIENTED_EDGE ( 'NONE', *, *, #31333, .T. ) ;
#40184=CARTESIAN_POINT ( 'NONE',  ( -9.663285910017000546, -79.20140313587198477, 5.577858467032999812 ) ) ;
#40186=CARTESIAN_POINT ( 'NONE',  ( 0.000000000000000000, -76.39999999999999147, 0.000000000000000000 ) ) ;
#40188=VECTOR ( 'NONE', #50143, 1000.000000000000114 ) ;
#40189=ADVANCED_FACE ( 'NONE', ( #45495 ), #44596, .F. ) ;
#40192=CIRCLE ( 'NONE', #17572, 4.100000000000000533 ) ;
#40208=CARTESIAN_POINT ( 'NONE',  ( -5.647686975130659981, -78.17275673027563698, -7.326454094270782313 ) ) ;
#40213=CARTESIAN_POINT ( 'NONE',  ( 1.967341388825386339, -77.45803376817946173, 9.038427814231061674 ) ) ;
#40214=CARTESIAN_POINT ( 'NONE',  ( -9.808193611224998776, -77.89219955680599128, 5.067887917229000116 ) ) ;
#40216=CARTESIAN_POINT ( 'NONE',  ( -7.456816947376000648, -78.83519289764198845, 6.210200510404999541 ) ) ;
#40221=CARTESIAN_POINT ( 'NONE',  ( -4.017143116098000455, -80.39449815114798525, 10.51352533724000082 ) ) ;
#40251=DIRECTION ( 'NONE',  ( -1.000000000000000000, 0.000000000000000000, 0.000000000000000000 ) ) ;
#40264=CARTESIAN_POINT ( 'NONE',  ( 0.000000000000000000, -81.89999999962999766, -4.199999999630000147 ) ) ;
#40291=EDGE_LOOP ( 'NONE', ( #37854, #27336, #6836, #46433 ) ) ;
#40294=CARTESIAN_POINT ( 'NONE',  ( 10.69999999997999929, -81.80000000002199556, -2.760617010408999913E-10 ) ) ;
#40297=CARTESIAN_POINT ( 'NONE',  ( 6.240531904507999883, -78.02895987979198367, 7.431451467605000083 ) ) ;
#40317=CARTESIAN_POINT ( 'NONE',  ( 10.71369944335147828, -78.42916666666667425, -2.879226727952064913 ) ) ;
#40327=CARTESIAN_POINT ( 'NONE',  ( -11.26138982850999959, -77.18296943548479305, -0.5357607033695001020 ) ) ;
#40331=CARTESIAN_POINT ( 'NONE',  ( -9.269208960685000775, -78.47531894259199703, -2.179940704506999616 ) ) ;
#40341=B_SPLINE_CURVE_WITH_KNOTS ( 'NONE', 3,
 ( #39425, #21700, #30837, #16993 ),
 .UNSPECIFIED., .F., .F.,
 ( 4, 4 ),
 ( 0.000000000000000000, 1.000000000000000000 ),
 .UNSPECIFIED. ) ;
#40354=CARTESIAN_POINT ( 'NONE',  ( -4.373213035511999358, -79.83807026975351562, -8.733596771889999388 ) ) ;
#40355=EDGE_LOOP ( 'NONE', ( #34150, #21750, #11398, #55390 ) ) ;
#40357=ORIENTED_EDGE ( 'NONE', *, *, #25865, .F. ) ;
#40360=CARTESIAN_POINT ( 'NONE',  ( -9.250000000000000000, -78.49999999999998579, 0.000000000000000000 ) ) ;
#40369=CARTESIAN_POINT ( 'NONE',  ( -1.439896632895359962, -78.48541666666665151, 10.99999999999999645 ) ) ;
#40373=AXIS2_PLACEMENT_3D ( 'NONE', #11293, #42876, #6561 ) ;
#40374=CARTESIAN_POINT ( 'NONE',  ( -6.760013919724099374, -78.02708333333333712, 8.796335266379958995 ) ) ;
#40399=CARTESIAN_POINT ( 'NONE',  ( -9.055195227533998192, -78.85919638534799958, -3.586521308946000186 ) ) ;
#40407=VECTOR ( 'NONE', #3844, 1000.000000000000000 ) ;
#40412=FACE_OUTER_BOUND ( 'NONE', #10439, .T. ) ;
#40421=CARTESIAN_POINT ( 'NONE',  ( 5.496668217546000434, -80.00271666237398449, -8.073860231047000013 ) ) ;
#40436=CARTESIAN_POINT ( 'NONE',  ( 8.132368178600600572, -79.89002859466290829, 4.407339140889335205 ) ) ;
#40438=CARTESIAN_POINT ( 'NONE',  ( -4.097768037502161675, -80.35541789187665529, 10.32471114121541866 ) ) ;
#40439=EDGE_LOOP ( 'NONE', ( #29103, #38460, #57165, #24525 ) ) ;
#40441=CARTESIAN_POINT ( 'NONE',  ( 2.878446107591830394, -77.25035309939079298, -8.790621935832806599 ) ) ;
#40455=VERTEX_POINT ( 'NONE', #17655 ) ;
#40460=DIRECTION ( 'NONE',  ( 0.000000000000000000, 1.000000000000000000, 0.000000000000000000 ) ) ;
#40472=CARTESIAN_POINT ( 'NONE',  ( 9.981840466370998755, -78.71427596511499303, 4.563647388395000171 ) ) ;
#40473=CARTESIAN_POINT ( 'NONE',  ( -11.00000000000000000, -79.11041666666666572, -1.439896632895321327 ) ) ;
#40478=EDGE_CURVE ( 'NONE', #20614, #17190, #32315, .T. ) ;
#40480=CARTESIAN_POINT ( 'NONE',  ( 7.910248556510421025, -77.20622010308966310, -4.849172256848496509 ) ) ;
#40484=CARTESIAN_POINT ( 'NONE',  ( 5.365758882164000099, -78.14158470334899675, 9.658494679878000255 ) ) ;
#40489=CARTESIAN_POINT ( 'NONE',  ( -1.210822168571097146, -79.88541666666665719, 9.249999999999992895 ) ) ;
#40490=CARTESIAN_POINT ( 'NONE',  ( -6.272971974831352604, -79.62293377770998859, 9.114735501174530796 ) ) ;
#40492=EDGE_LOOP ( 'NONE', ( #44199, #42236, #6010, #44605, #45965, #46252, #46127, #26457, #11884, #32203, #44028 ) ) ;
#40493=EDGE_LOOP ( 'NONE', ( #5082, #50755, #49816, #50365 ) ) ;
#40495=EDGE_CURVE ( 'NONE', #15896, #10446, #54268, .T. ) ;
#40498=VERTEX_POINT ( 'NONE', #13209 ) ;
#40499=CARTESIAN_POINT ( 'NONE',  ( -7.255724684302470529, -79.80670072624305078, -6.257106228078864518 ) ) ;
#40503=CIRCLE ( 'NONE', #44249, 2.799999999999999822 ) ;
#40504=LINE ( 'NONE', #34393, #6105 ) ;
#40506=CARTESIAN_POINT ( 'NONE',  ( -5.862706933886596694, -78.17042577989984409, -7.154751683068700352 ) ) ;
#40512=CARTESIAN_POINT ( 'NONE',  ( 6.771057570713677976, -77.40985474823717993, 6.320815176807171198 ) ) ;
#40513=CARTESIAN_POINT ( 'NONE',  ( -11.00724581733999941, -77.86370633980098432, 0.8512868710715000287 ) ) ;
#40516=CARTESIAN_POINT ( 'NONE',  ( 8.898653440358000211, -78.60780226460998676, -3.871004561473999850 ) ) ;
#40535=CARTESIAN_POINT ( 'NONE',  ( 0.7438124352902001357, -80.49061853915497977, 11.37744605582999924 ) ) ;
#40552=EDGE_CURVE ( 'NONE', #52990, #18080, #39864, .T. ) ;
#40556=ADVANCED_FACE ( 'NONE', ( #57799 ), #28580, .F. ) ;
#40570=CARTESIAN_POINT ( 'NONE',  ( -2.879226727952091114, -79.49583333333333712, 10.71369944335146940 ) ) ;
#40574=ORIENTED_EDGE ( 'NONE', *, *, #52223, .F. ) ;
#40575=CIRCLE ( 'NONE', #6606, 4.100000000000000533 ) ;
#40581=CARTESIAN_POINT ( 'NONE',  ( -10.55592303174000079, -79.87819379990754953, -3.904632140252999317 ) ) ;
#40586=CARTESIAN_POINT ( 'NONE',  ( -1.776188306762000124, -77.46214197229863885, -10.89629776253999971 ) ) ;
#40590=EDGE_LOOP ( 'NONE', ( #51324, #31632, #49969, #4623 ) ) ;
#40595=CARTESIAN_POINT ( 'NONE',  ( -9.669247687117000112, -77.71629775937297779, -0.8224101967608999919 ) ) ;
#40606=CARTESIAN_POINT ( 'NONE',  ( 10.36935812844000004, -78.17876026662598576, -2.835297515976000327 ) ) ;
#40615=CARTESIAN_POINT ( 'NONE',  ( -8.796335266380001627, -79.14791666666667425, 6.760013919724038978 ) ) ;
#40618=CARTESIAN_POINT ( 'NONE',  ( -9.385460185241999653, -79.85105627184799459, -2.646321958768000471 ) ) ;
#40629=CARTESIAN_POINT ( 'NONE',  ( -3.470329948268000120, -78.36162362607598197, 8.867197205552999506 ) ) ;
#40651=DIRECTION ( 'NONE',  ( 1.776356839400000238E-14, 1.000000000000000000, -1.894780628693999933E-13 ) ) ;
#40663=CARTESIAN_POINT ( 'NONE',  ( 7.719754268718227230, -78.80359534466445837, -5.095877674619078590 ) ) ;
#40667=CARTESIAN_POINT ( 'NONE',  ( 2.421252246090693117, -77.74597346547214727, -9.009672662381980501 ) ) ;
#40679=CARTESIAN_POINT ( 'NONE',  ( 7.355581160863136070, -79.79837709061000339, -5.642938462726122317 ) ) ;
#40683=CARTESIAN_POINT ( 'NONE',  ( 10.36935812844000004, -78.07876026662599145, -2.835297515976000327 ) ) ;
#40687=CARTESIAN_POINT ( 'NONE',  ( -2.769480662737825227, -78.20484845553691855, -10.72687993797705985 ) ) ;
#40690=DIRECTION ( 'NONE',  ( 0.000000000000000000, 1.000000000000000000, 0.000000000000000000 ) ) ;
#40705=CARTESIAN_POINT ( 'NONE',  ( -0.9882926940093508250, -76.99166666656056179, -9.458333332648651393 ) ) ;
#40713=CARTESIAN_POINT ( 'NONE',  ( -6.146531642657000027, -77.91423522357898435, 9.376936153619999104 ) ) ;
#40720=CARTESIAN_POINT ( 'NONE',  ( 8.985706068735000329, -79.54809944676298983, -3.828549499589000149 ) ) ;
#40732=CARTESIAN_POINT ( 'NONE',  ( 2.867548251969000095, -77.89887176884063535, -9.270807752789000489 ) ) ;
#40733=CARTESIAN_POINT ( 'NONE',  ( 5.960820980064980290, -79.91975476581831117, 7.102596592892035154 ) ) ;
#40736=CARTESIAN_POINT ( 'NONE',  ( -6.294203684166999935, -77.18138806810267738, 7.343715272572999275 ) ) ;
#40737=CARTESIAN_POINT ( 'NONE',  ( 2.922072168813211412, -77.25074815672523698, -8.776223896002093738 ) ) ;
#40742=CARTESIAN_POINT ( 'NONE',  ( 5.500000000000000000, -80.99999999999998579, 0.000000000000000000 ) ) ;
#40746=ORIENTED_EDGE ( 'NONE', *, *, #42061, .T. ) ;
#40755=CARTESIAN_POINT ( 'NONE',  ( 4.510926502723999754, -77.54314704349698673, 8.509098192649000580 ) ) ;
#40764=CARTESIAN_POINT ( 'NONE',  ( 10.55657102546000026, -78.65809125644999256, -3.003801718854000047 ) ) ;
#40765=CARTESIAN_POINT ( 'NONE',  ( -1.439896632895338202, -79.21458333333333712, -10.99999999999999822 ) ) ;
#40777=CARTESIAN_POINT ( 'NONE',  ( 10.73159385090000129, -78.47100192322299961, -3.053603293876000269 ) ) ;
#40781=CARTESIAN_POINT ( 'NONE',  ( -1.842497806997727139, -79.58834702216799428, 10.91026042240053862 ) ) ;
#40789=CARTESIAN_POINT ( 'NONE',  ( 10.90625000000000000, -80.29374999999798490, -5.301077343649000152E-10 ) ) ;
#40795=CARTESIAN_POINT ( 'NONE',  ( -5.812602142628422897, -78.17097178526422852, -7.195572196038425794 ) ) ;
#40796=AXIS2_PLACEMENT_3D ( 'NONE', #51366, #50785, #23321 ) ;
#40800=LINE ( 'NONE', #14215, #49138 ) ;
#40801=EDGE_LOOP ( 'NONE', ( #17851, #33513, #4379, #37746 ) ) ;
#40802=CARTESIAN_POINT ( 'NONE',  ( -1.490426546943438124, -77.48793975142889678, 9.129111009367720797 ) ) ;
#40803=CARTESIAN_POINT ( 'NONE',  ( -6.065106684382000068, -77.41173743516598904, 9.224892016835999797 ) ) ;
#40805=EDGE_CURVE ( 'NONE', #13326, #27414, #42884, .T. ) ;
#40806=CARTESIAN_POINT ( 'NONE',  ( -4.475245744599999576, -78.97731204328599119, -8.610626265545000990 ) ) ;
#40813=B_SPLINE_CURVE_WITH_KNOTS ( 'NONE', 3,
 ( #37619, #50643, #51513, #15486, #47382, #42646, #20213, #33178, #51225, #6914 ),
 .UNSPECIFIED., .F., .F.,
 ( 4, 2, 2, 2, 4 ),
 ( 0.000000000000000000, 0.2500000000000000000, 0.5000000000000000000, 0.7500000000000000000, 1.000000000000000000 ),
 .UNSPECIFIED. ) ;
#40814=CARTESIAN_POINT ( 'NONE',  ( 7.195688986358000250, -79.24706562342598204, 8.240744890341000328 ) ) ;
#40816=CARTESIAN_POINT ( 'NONE',  ( 5.684557159767975598, -78.67708333333330017, -7.396918292183157106 ) ) ;
#40828=CARTESIAN_POINT ( 'NONE',  ( -4.165479847964999927, -80.46200396371098407, 10.49531740235000044 ) ) ;
#40832=ORIENTED_EDGE ( 'NONE', *, *, #32647, .T. ) ;
#40838=CARTESIAN_POINT ( 'NONE',  ( -8.796335266379976758, -79.75208333333333144, -6.760013919724066511 ) ) ;
#40840=DIRECTION ( 'NONE',  ( 0.000000000000000000, 1.000000000000000000, 0.000000000000000000 ) ) ;
#40852=CARTESIAN_POINT ( 'NONE',  ( 2.632967082928999947, -77.24351440681299152, 9.306700570505000769 ) ) ;
#40855=CARTESIAN_POINT ( 'NONE',  ( 10.92207628522714202, -78.10253042142522872, 0.3426783470800407461 ) ) ;
#40861=DIRECTION ( 'NONE',  ( -1.000000000000000000, 0.000000000000000000, 0.000000000000000000 ) ) ;
#40882=CARTESIAN_POINT ( 'NONE',  ( -9.346518596363001308, -77.68787393024398114, 2.610229778083999808 ) ) ;
#40889=CARTESIAN_POINT ( 'NONE',  ( 7.000000000000000000, -80.99999999999998579, 0.000000000000000000 ) ) ;
#40897=CONICAL_SURFACE ( 'NONE', #31434, 1.099999997148999986, 0.7853981633972997312 ) ;
#40899=CARTESIAN_POINT ( 'NONE',  ( 0.000000000000000000, -76.89999999999999147, 0.000000000000000000 ) ) ;
#40921=CARTESIAN_POINT ( 'NONE',  ( -9.411482030169999291, -79.02239977856800124, -0.1876179646513999877 ) ) ;
#40934=CARTESIAN_POINT ( 'NONE',  ( 9.203868716350999790, -79.66626286943098023, 5.914103205931999341 ) ) ;
#40940=VERTEX_POINT ( 'NONE', #48192 ) ;
#40957=CARTESIAN_POINT ( 'NONE',  ( 6.650092250953310469, -78.78900554370888187, -6.429455470012980456 ) ) ;
#40961=DIRECTION ( 'NONE',  ( 0.000000000000000000, 1.000000000000000000, 0.000000000000000000 ) ) ;
#40969=CARTESIAN_POINT ( 'NONE',  ( -2.799999999999999822, -78.69999999999998863, 0.000000000000000000 ) ) ;
#41004=ORIENTED_EDGE ( 'NONE', *, *, #9898, .T. ) ;
#41005=CARTESIAN_POINT ( 'NONE',  ( -1.333681084703000064, -77.87755051491399172, 11.13229884148000082 ) ) ;
#41011=CARTESIAN_POINT ( 'NONE',  ( -7.545891804452000251, -79.95556382368950210, 6.201630566990999682 ) ) ;
#41023=CARTESIAN_POINT ( 'NONE',  ( 9.177586578508210025, -79.86080595070167476, 1.207628619463350983 ) ) ;
#41038=DIRECTION ( 'NONE',  ( 0.000000000000000000, -1.000000000000000000, 0.000000000000000000 ) ) ;
#41051=CARTESIAN_POINT ( 'NONE',  ( -5.310864497047000476, -77.62841853088399091, 8.034172531070000289 ) ) ;
#41059=CARTESIAN_POINT ( 'NONE',  ( 3.176617583302000281, -79.84208835542798965, 10.50586082162000068 ) ) ;
#41062=DIRECTION ( 'NONE',  ( 1.000000000000000000, 0.000000000000000000, 0.000000000000000000 ) ) ;
#41071=CARTESIAN_POINT ( 'NONE',  ( -10.72788417900999924, -78.78770885299998383, 2.643935454766999982 ) ) ;
#41075=CARTESIAN_POINT ( 'NONE',  ( 7.788616085187482163, -78.76231864851705211, 7.733387248865380315 ) ) ;
#41095=CARTESIAN_POINT ( 'NONE',  ( 2.852630567793418059, -77.45022947118953027, 8.799033844256978654 ) ) ;
#41096=CARTESIAN_POINT ( 'NONE',  ( 6.574300740938999077, -77.60591217881798798, -8.869200617850999890 ) ) ;
#41098=CARTESIAN_POINT ( 'NONE',  ( 3.248345031021000029, -78.23829248593298757, 9.144340540792999406 ) ) ;
#41103=CARTESIAN_POINT ( 'NONE',  ( 2.542269563431000190, -78.57284911944198313, -10.64070870773999822 ) ) ;
#41116=CARTESIAN_POINT ( 'NONE',  ( -5.511117113485999752, -78.15441511928399621, -7.631433854063000233 ) ) ;
#41125=CARTESIAN_POINT ( 'NONE',  ( -9.813193589766999736, -78.84650130276799018, -4.915816122623000162 ) ) ;
#41128=EDGE_CURVE ( 'NONE', #53170, #31439, #52832, .T. ) ;
#41140=CARTESIAN_POINT ( 'NONE',  ( -0.8405563561534999950, -76.94822717842869508, -9.635375415708001157 ) ) ;
#41143=CARTESIAN_POINT ( 'NONE',  ( -9.250000000000000000, -77.99999999999998579, 0.000000000000000000 ) ) ;
#41152=DIRECTION ( 'NONE',  ( 0.000000000000000000, 1.000000000000000000, 0.000000000000000000 ) ) ;
#41159=CARTESIAN_POINT ( 'NONE',  ( 6.068451062995785072, -78.28202394152809518, -6.981743368066175570 ) ) ;
#41170=CARTESIAN_POINT ( 'NONE',  ( -0.5548610165507998904, -77.82999307588899285, -9.688283574444998436 ) ) ;
#41173=AXIS2_PLACEMENT_3D ( 'NONE', #47527, #29187, #15914 ) ;
#41190=CARTESIAN_POINT ( 'NONE',  ( 10.00419727105263057, -77.19999999999998863, -4.081745277459294385 ) ) ;
#41191=ORIENTED_EDGE ( 'NONE', *, *, #24298, .T. ) ;
#41195=CARTESIAN_POINT ( 'NONE',  ( 1.677867312386000176, -79.96794690487999446, -9.605949203754001076 ) ) ;
#41199=FACE_OUTER_BOUND ( 'NONE', #56484, .T. ) ;
#41202=CARTESIAN_POINT ( 'NONE',  ( 1.956384561158000190, -77.10404663294119132, 10.99260293793000010 ) ) ;
#41205=CARTESIAN_POINT ( 'NONE',  ( -0.1509935689429000305, -78.33319979694698532, 9.520902119764999227 ) ) ;
#41211=AXIS2_PLACEMENT_3D ( 'NONE', #22951, #40961, #2987 ) ;
#41212=EDGE_CURVE ( 'NONE', #6548, #32058, #57024, .T. ) ;
#41224=ORIENTED_EDGE ( 'NONE', *, *, #33890, .F. ) ;
#41234=CARTESIAN_POINT ( 'NONE',  ( 8.240271889161402186, -78.05562457600899506, -5.125597231812675680 ) ) ;
#41243=CARTESIAN_POINT ( 'NONE',  ( 7.846823748142760735, -78.80564564162774843, -4.898151885573968300 ) ) ;
#41248=CARTESIAN_POINT ( 'NONE',  ( -5.640425023195567711, -80.18229393084122592, -9.443705758514129300 ) ) ;
#41253=CARTESIAN_POINT ( 'NONE',  ( -9.254388464354001087, -79.90752053325199711, 5.469807505829999528 ) ) ;
#41260=CARTESIAN_POINT ( 'NONE',  ( 8.027497949466866345, -79.80879597959544469, -4.635833453492248957 ) ) ;
#41261=AXIS2_PLACEMENT_3D ( 'NONE', #11042, #42615, #2181 ) ;
#41267=CARTESIAN_POINT ( 'NONE',  ( -2.402886566874598451, -77.34315645986228560, 10.56757644837470700 ) ) ;
#41276=CARTESIAN_POINT ( 'NONE',  ( -9.260506811358984791, -80.00000000000000000, -0.7327802946142877305 ) ) ;
#41281=CARTESIAN_POINT ( 'NONE',  ( 1.692299031616999905, -79.40949596206999672, -9.745343228177999251 ) ) ;
#41293=ORIENTED_EDGE ( 'NONE', *, *, #49269, .F. ) ;
#41295=CARTESIAN_POINT ( 'NONE',  ( -6.151115499150000332, -77.13436266505908634, -9.032717438718000480 ) ) ;
#41300=CARTESIAN_POINT ( 'NONE',  ( 9.647254834573999460, -80.24781774801149936, -1.526580663425000095 ) ) ;
#41312=CARTESIAN_POINT ( 'NONE',  ( 8.949233952815241366, -79.87044664050942799, 2.340432196254297548 ) ) ;
#41317=B_SPLINE_CURVE_WITH_KNOTS ( 'NONE', 3,
 ( #10837, #42123, #31853, #28813, #47155, #13562, #19982, #46570, #323, #46861, #6389, #6685, #50987, #22719, #24404, #15245, #42419, #1689, #24693, #33537, #19392, #5802, #49894, #1988, #45170, #19681, #54317, #37969, #4720, #51574, #6094, #10538, #37681, #51283, #33239, #11131, #37384, #55994, #25, #15540, #40732, #29109, #35996, #9438, #1398, #49600, #54021, #9148, #27132, #18301, #36294, #13857, #27429, #45464, #23808, #41824, #55400, #14947, #32945, #28521, #7838, #39426, #43571, #43285, #11705 ),
 .UNSPECIFIED., .F., .F.,
 ( 4, 1, 1, 1, 1, 1, 1, 1, 1, 1, 1, 1, 1, 1, 1, 1, 1, 1, 1, 1, 1, 1, 1, 1, 1, 1, 1, 1, 1, 1, 1, 1, 1, 1, 1, 1, 1, 1, 1, 1, 1, 1, 1, 1, 1, 1, 1, 1, 1, 1, 1, 1, 1, 1, 1, 1, 1, 1, 1, 1, 1, 1, 4 ),
 ( 0.000000000000000000, 0.01249973505302583512, 0.02874974388395608663, 0.04499975271488634160, 0.06124976154581659310, 0.07749977037674685154, 0.09374977920767710304, 0.1099997880386073545, 0.1262497968695376060, 0.1424998057004678575, 0.1587498145313981091, 0.1749998233623283606, 0.1912498321932586398, 0.2074998410241888636, 0.2237498498551191428, 0.2399998586860493666, 0.2562498675169795903, 0.2724998763479098973, 0.2887498851788401488, 0.3049998940097703448, 0.3212499028407005963, 0.3374999116716309033, 0.3537499205025611548, 0.3699999293334913508, 0.3862499381644216023, 0.4024999469953519093, 0.4187499558262821608, 0.4349999646572124123, 0.4512499734881426083, 0.4674999823190729153, 0.4837499911500031669, 0.4999999999809334184, 0.5162500088118636699, 0.5325000176427939769, 0.5487500264737241729, 0.5650000353046543689, 0.5812500441355847869, 0.5975000529665149829, 0.6137500617974452899, 0.6300000706283754859, 0.6462500794593056819, 0.6625000882902359889, 0.6787500971211661849, 0.6950001059520964919, 0.7112501147830267989, 0.7275001236139569949, 0.7437501324448873019, 0.7600001412758174979, 0.7762501501067478049, 0.7925001589376780009, 0.8087501677686081969, 0.8250001765995385039, 0.8412501854304688109, 0.8575001942613991179, 0.8737502030923293139, 0.8900002119232595099, 0.9062502207541898169, 0.9225002295851200129, 0.9387502384160503199, 0.9550002472469805159, 0.9712502560779107119, 0.9875002649088411300, 1.000000000000000000 ),
 .UNSPECIFIED. ) ;
#41326=CARTESIAN_POINT ( 'NONE',  ( 3.229284361504000334, -79.90857183731299074, 10.68004289648999894 ) ) ;
#41339=CARTESIAN_POINT ( 'NONE',  ( -1.186507705731999929, -78.88609509508398787, -9.667052097962999468 ) ) ;
#41346=DIRECTION ( 'NONE',  ( -1.000000000000000000, 0.000000000000000000, 0.000000000000000000 ) ) ;
#41350=CARTESIAN_POINT ( 'NONE',  ( -10.57157196544999955, -79.97318600897997953, 2.324769239444999691 ) ) ;
#41351=CARTESIAN_POINT ( 'NONE',  ( -5.539808784079904846, -79.18333333333332291, -9.611650271896831299 ) ) ;
#41368=DIRECTION ( 'NONE',  ( 0.000000000000000000, 0.7071067811866525998, -0.7071067811864425456 ) ) ;
#41369=CARTESIAN_POINT ( 'NONE',  ( 6.084059575412256393, -78.62185687685334301, -9.135208697462157801 ) ) ;
#41377=CARTESIAN_POINT ( 'NONE',  ( 9.552813797205702784, -80.26770833350961709, -5.504922207147467716 ) ) ;
#41379=AXIS2_PLACEMENT_3D ( 'NONE', #26205, #16494, #47526 ) ;
#41388=CARTESIAN_POINT ( 'NONE',  ( 9.132654035730695341, -77.36284952363988054, 1.468098543608952422 ) ) ;
#41389=CARTESIAN_POINT ( 'NONE',  ( -5.876696946710000091, -77.51048305282198214, -9.346046374399000101 ) ) ;
#41397=CARTESIAN_POINT ( 'NONE',  ( 10.84079038992999955, -79.66845093841598668, -1.471421101766999806 ) ) ;
#41419=PRODUCT_DEFINITION_FORMATION_WITH_SPECIFIED_SOURCE ( 'ANY', '', #41849, .NOT_KNOWN. ) ;
#41421=CARTESIAN_POINT ( 'NONE',  ( -5.755176823513999729, -78.28877243311998768, 9.345691860246999383 ) ) ;
#41425=CARTESIAN_POINT ( 'NONE',  ( 0.000000000000000000, -74.99999999999998579, -4.299999999999978506 ) ) ;
#41429=EDGE_CURVE ( 'NONE', #28511, #24529, #38584, .T. ) ;
#41431=CARTESIAN_POINT ( 'NONE',  ( 2.618044012240999585, -78.32284911944198313, -10.95786383906999895 ) ) ;
#41446=ORIENTED_EDGE ( 'NONE', *, *, #29345, .F. ) ;
#41452=CYLINDRICAL_SURFACE ( 'NONE', #7552, 11.00000000000000000 ) ;
#41455=CARTESIAN_POINT ( 'NONE',  ( 7.275474750695519077, -78.29713309960814627, -5.714788711246518105 ) ) ;
#41463=CARTESIAN_POINT ( 'NONE',  ( -5.351292223237999579, -77.69132919765699796, 8.095330809056001442 ) ) ;
#41476=CONICAL_SURFACE ( 'NONE', #28269, 10.59999999995999964, 0.7853981633972997312 ) ;
#41479=DIRECTION ( 'NONE',  ( 1.000000000000000000, 0.000000000000000000, 0.000000000000000000 ) ) ;
#41480=CARTESIAN_POINT ( 'NONE',  ( 2.639686428813980079, -77.20000000000000284, -10.63845845605472107 ) ) ;
#41485=CARTESIAN_POINT ( 'NONE',  ( -9.270924421324000519, -79.35427108146299702, -3.023218246060999981 ) ) ;
#41490=ADVANCED_FACE ( 'NONE', ( #507 ), #31743, .F. ) ;
#41492=CARTESIAN_POINT ( 'NONE',  ( -9.929563311754000310, -77.63992477412999449, 5.339448599216000346 ) ) ;
#41498=CARTESIAN_POINT ( 'NONE',  ( -7.831519877845000366, -78.56761851250499262, -5.222881475815000840 ) ) ;
#41511=EDGE_CURVE ( 'NONE', #18212, #28960, #53574, .T. ) ;
#41519=ORIENTED_EDGE ( 'NONE', *, *, #12890, .F. ) ;
#41521=DIRECTION ( 'NONE',  ( -1.000000000000000000, 0.000000000000000000, 0.000000000000000000 ) ) ;
#41525=CARTESIAN_POINT ( 'NONE',  ( 1.211040244683831313, -79.23558525598221536, -9.190809572653749981 ) ) ;
#41526=CARTESIAN_POINT ( 'NONE',  ( -2.183148623211547346, -77.74296245559024499, 9.455563964093084195 ) ) ;
#41530=B_SPLINE_CURVE_WITH_KNOTS ( 'NONE', 3,
 ( #24443, #33281, #51321, #15287, #28850, #38007, #41377, #960, #36354, #40789 ),
 .UNSPECIFIED., .F., .F.,
 ( 4, 2, 2, 2, 4 ),
 ( 0.1666666723472590150, 0.3750000042604442752, 0.5833333361736294798, 0.7916666680868147399, 1.000000000000000000 ),
 .UNSPECIFIED. ) ;
#41534=CARTESIAN_POINT ( 'NONE',  ( 7.033247818498722381, -78.79382002255685791, -6.010734345524098465 ) ) ;
#41539=CARTESIAN_POINT ( 'NONE',  ( -8.367750842354992002, -80.15659319994234977, -7.184025905134648227 ) ) ;
#41566=CARTESIAN_POINT ( 'NONE',  ( 8.315784280752016144, -78.31395558942278967, -4.050953114190261495 ) ) ;
#41571=CARTESIAN_POINT ( 'NONE',  ( -1.553298277364999924, -78.78095298048599204, 9.504760619105999453 ) ) ;
#41582=VERTEX_POINT ( 'NONE', #8740 ) ;
#41586=CARTESIAN_POINT ( 'NONE',  ( -4.716706279917999289, -77.08271516049769900, -9.880723834468000177 ) ) ;
#41590=B_SPLINE_CURVE_WITH_KNOTS ( 'NONE', 3,
 ( #36400, #45574, #31665, #31960, #45279, #48324, #44174, #9549, #52742, #13963, #49711, #34997, #22827, #40838, #18408, #12294, #7864, #21439 ),
 .UNSPECIFIED., .F., .F.,
 ( 4, 2, 2, 2, 2, 2, 2, 2, 4 ),
 ( 0.000000000000000000, 0.1250000000000000000, 0.2500000000000000000, 0.3750000000000000000, 0.5000000000000000000, 0.6250000000000000000, 0.7500000000000000000, 0.8750000000000000000, 1.000000000000000000 ),
 .UNSPECIFIED. ) ;
#41592=CARTESIAN_POINT ( 'NONE',  ( 9.534323188421000239, -79.13213671798298776, -1.008198710029000189 ) ) ;
#41601=LINE ( 'NONE', #10908, #47802 ) ;
#41603=CARTESIAN_POINT ( 'NONE',  ( 9.537698866016000920, -77.04321742767268688, 2.758499149798000261 ) ) ;
#41614=EDGE_CURVE ( 'NONE', #34245, #46717, #57743, .T. ) ;
#41622=CARTESIAN_POINT ( 'NONE',  ( -0.5026956014243000315, -77.27223151488298925, 9.585737870937999006 ) ) ;
#41627=CARTESIAN_POINT ( 'NONE',  ( -9.275907895452998986, -77.68526618914199844, 2.590510119660999866 ) ) ;
#41637=CARTESIAN_POINT ( 'NONE',  ( -10.96673197750000206, -78.49365534745898287, -0.4413686857046000278 ) ) ;
#41638=CARTESIAN_POINT ( 'NONE',  ( 8.796335266379964324, -79.29791666666666572, -6.760013919724084275 ) ) ;
#41649=B_SPLINE_CURVE_WITH_KNOTS ( 'NONE', 3,
 ( #17452, #43465, #57321, #31300, #30149, #21874 ),
 .UNSPECIFIED., .F., .F.,
 ( 4, 2, 4 ),
 ( 0.000000000000000000, 0.5000000000000000000, 1.000000000000000000 ),
 .UNSPECIFIED. ) ;
#41652=ADVANCED_FACE ( 'NONE', ( #26437 ), #15180, .F. ) ;
#41654=EDGE_CURVE ( 'NONE', #32058, #45010, #28144, .T. ) ;
#41657=CARTESIAN_POINT ( 'NONE',  ( -7.508608642448520776, -79.01514983751106058, -8.005536529047017069 ) ) ;
#41675=CARTESIAN_POINT ( 'NONE',  ( 9.129142538877060176, -77.36303958135555092, 1.489769077664636843 ) ) ;
#41680=CARTESIAN_POINT ( 'NONE',  ( -9.282419925074000489, -77.41400144119299398, -2.829762163499999872 ) ) ;
#41685=EDGE_CURVE ( 'NONE', #29148, #53060, #4133, .T. ) ;
#41686=CARTESIAN_POINT ( 'NONE',  ( 0.9061038674864000386, -78.79758795410299399, 10.90260483175000061 ) ) ;
#41697=CONICAL_SURFACE ( 'NONE', #1224, 10.59999999997999787, 0.7853981633972997312 ) ;
#41698=FACE_OUTER_BOUND ( 'NONE', #21932, .T. ) ;
#41701=CARTESIAN_POINT ( 'NONE',  ( -6.279067761433998918, -78.01229597363898449, 7.013166371532999932 ) ) ;
#41707=EDGE_LOOP ( 'NONE', ( #57197, #3678 ) ) ;
#41711=CARTESIAN_POINT ( 'NONE',  ( 9.304500756975000897, -79.01505542876398636, -5.821536072646999571 ) ) ;
#41724=VECTOR ( 'NONE', #39776, 1000.000000000000000 ) ;
#41726=CARTESIAN_POINT ( 'NONE',  ( 5.330173052271000245, -78.18464638465644612, 9.594439332582000546 ) ) ;
#41737=B_SPLINE_CURVE_WITH_KNOTS ( 'NONE', 3,
 ( #36250, #14676, #1138, #49849, #19418, #32674, #9684, #28248, #5252, #14974, #54842, #54270, #18547, #41267, #31806, #9393, #50430, #9980, #27960, #19125, #46010, #5532, #23542, #32972, #46597, #22968, #37118, #50727, #42147, #29420, #11157, #2579, #2012, #55729, #52960, #26079, #20010, #43022, #29131, #33561, #30508, #20291, #42732, #2295, #24428, #15860, #6710, #24719, #6999, #33267, #51599, #51307, #10866, #38285, #34129, #15272, #44104, #56307, #37992, #47178, #6415, #47473, #28837, #16153, #25001, #20580, #33847, #51884, #11441, #38578, #56594, #12509, #46886, #48536, #8082, #3653, #1716, #19709, #37707, #42444, #15567, #56018, #14874, #55329 ),
 .UNSPECIFIED., .F., .F.,
 ( 4, 2, 1, 2, 2, 2, 2, 2, 2, 2, 1, 2, 2, 2, 2, 2, 2, 2, 1, 2, 2, 2, 2, 2, 2, 2, 1, 2, 2, 2, 2, 2, 2, 2, 1, 2, 2, 2, 2, 2, 2, 2, 1, 2, 4 ),
 ( 0.000000000000000000, 0.01562500000000001735, 0.03125000000000003469, 0.04687500000000006245, 0.06250000000000008327, 0.09375000000000012490, 0.1250000000000001665, 0.1562500000000001943, 0.1875000000000002776, 0.2031250000000002776, 0.2187500000000003053, 0.2343750000000003053, 0.2500000000000003331, 0.2812500000000003886, 0.3125000000000003886, 0.3437500000000003886, 0.3750000000000004441, 0.3906250000000004441, 0.4062500000000004441, 0.4218750000000004441, 0.4375000000000004996, 0.4687500000000004996, 0.5000000000000005551, 0.5312500000000005551, 0.5625000000000006661, 0.5781250000000006661, 0.5937500000000006661, 0.6093750000000006661, 0.6250000000000006661, 0.6562500000000006661, 0.6875000000000005551, 0.7187500000000004441, 0.7500000000000003331, 0.7656250000000004441, 0.7812500000000004441, 0.7968750000000004441, 0.8125000000000004441, 0.8437500000000003331, 0.8750000000000003331, 0.9062500000000002220, 0.9375000000000001110, 0.9531250000000001110, 0.9687500000000000000, 0.9843750000000000000, 1.000000000000000000 ),
 .UNSPECIFIED. ) ;
#41748=CARTESIAN_POINT ( 'NONE',  ( 3.554000211758443051, -78.25642266958941207, -8.539967886276961906 ) ) ;
#41752=CARTESIAN_POINT ( 'NONE',  ( -7.972207510795373153, -77.55765093248844266, 4.695355910174569658 ) ) ;
#41756=CARTESIAN_POINT ( 'NONE',  ( 5.927986824875999261, -77.94714365981798210, -7.683077610609999830 ) ) ;
#41770=CARTESIAN_POINT ( 'NONE',  ( -2.421446639644671883, -79.49607851752138288, 9.010234589867415878 ) ) ;
#41780=CARTESIAN_POINT ( 'NONE',  ( 2.879226727952084897, -79.05416666666667425, 10.71369944335147117 ) ) ;
#41784=AXIS2_PLACEMENT_3D ( 'NONE', #36031, #46085, #5610 ) ;
#41788=CARTESIAN_POINT ( 'NONE',  ( 9.921600000191999058, -77.46856652213799066, 5.354231256300999497 ) ) ;
#41791=CARTESIAN_POINT ( 'NONE',  ( 7.038692338534999315, -77.82859895515098003, 6.250440358128999563 ) ) ;
#41799=CARTESIAN_POINT ( 'NONE',  ( -5.800000004703999679, -81.00000000470399186, 2.775962718112000159E-08 ) ) ;
#41804=DIRECTION ( 'NONE',  ( 1.000000000000000000, 0.000000000000000000, 0.000000000000000000 ) ) ;
#41818=CARTESIAN_POINT ( 'NONE',  ( 0.6056591908766266741, -79.23038445115356865, -9.249560979224405344 ) ) ;
#41824=CARTESIAN_POINT ( 'NONE',  ( 9.131029190779001325, -77.47251433190575653, -3.285576857342999535 ) ) ;
#41831=CARTESIAN_POINT ( 'NONE',  ( -3.762297919178509531, -78.69173512211914101, -8.453695876167582668 ) ) ;
#41835=CARTESIAN_POINT ( 'NONE',  ( -7.609649279793637255, -80.16460715866527664, -7.942784592428623114 ) ) ;
#41849=PRODUCT ( 'Push Button Connector', 'Push Button Connector', '', ( #51493 ) ) ;
#41859=CARTESIAN_POINT ( 'NONE',  ( 7.565568292094223324, -78.30138424788611928, -5.321967902146258034 ) ) ;
#41863=CARTESIAN_POINT ( 'NONE',  ( 7.600999290758999827, -78.69568149309900207, 5.914221820906000460 ) ) ;
#41873=CARTESIAN_POINT ( 'NONE',  ( 8.923648882468999233, -79.87442432477398313, -7.337453855139000503 ) ) ;
#41876=CARTESIAN_POINT ( 'NONE',  ( -10.93752463681999920, -77.51070342825998694, -2.465225665228000018 ) ) ;
#41883=CARTESIAN_POINT ( 'NONE',  ( -2.116314338179000387, -80.11792711497950847, -9.535298106756000536 ) ) ;
#41897=CARTESIAN_POINT ( 'NONE',  ( 7.201514106410999538, -76.91319389792408856, -6.116891697219999813 ) ) ;
#41904=VECTOR ( 'NONE', #33055, 1000.000000000000114 ) ;
#41922=CARTESIAN_POINT ( 'NONE',  ( 2.268344470944000157, -78.91451892421298453, -9.471763527590001175 ) ) ;
#41924=DIRECTION ( 'NONE',  ( -1.000000000000000000, 0.000000000000000000, 0.000000000000000000 ) ) ;
#41932=CARTESIAN_POINT ( 'NONE',  ( 1.684372618195999927, -78.35319357579599853, 10.84559388857000073 ) ) ;
#41935=CARTESIAN_POINT ( 'NONE',  ( 7.743925494623000283, -79.84195935437298886, -5.791931050047999463 ) ) ;
#41950=CARTESIAN_POINT ( 'NONE',  ( -11.00000000000000000, -79.59999999999999432, 0.000000000000000000 ) ) ;
#41951=CARTESIAN_POINT ( 'NONE',  ( -9.813348458551734765, -78.98705748317810560, -4.915893702512511787 ) ) ;
#41954=ORIENTED_EDGE ( 'NONE', *, *, #51653, .F. ) ;
#41968=CARTESIAN_POINT ( 'NONE',  ( 8.792064078896341783, -77.37518554897279444, 2.874290267169839819 ) ) ;
#41973=AXIS2_PLACEMENT_3D ( 'NONE', #45570, #5117, #41924 ) ;
#41978=FACE_OUTER_BOUND ( 'NONE', #40492, .T. ) ;
#41981=CARTESIAN_POINT ( 'NONE',  ( -4.100000000000000533, -78.69999999999998863, 0.000000000000000000 ) ) ;
#42004=CARTESIAN_POINT ( 'NONE',  ( 1.684372618195999927, -78.23258772445399245, 10.84559388857000073 ) ) ;
#42014=AXIS2_PLACEMENT_3D ( 'NONE', #39507, #44230, #22072 ) ;
#42029=DIRECTION ( 'NONE',  ( -0.7071067811865474617, 0.7071067811865474617, 7.319413740254484567E-10 ) ) ;
#42040=CARTESIAN_POINT ( 'NONE',  ( 7.019650986448177754, -78.29361464504475521, -6.023984796694146659 ) ) ;
#42048=CARTESIAN_POINT ( 'NONE',  ( 3.248345031021000029, -78.11768663459099571, 9.144340540792999406 ) ) ;
#42061=EDGE_CURVE ( 'NONE', #29374, #58355, #40813, .T. ) ;
#42071=CARTESIAN_POINT ( 'NONE',  ( 5.812955055244049873, -77.19999999999998863, -9.242863774950786038 ) ) ;
#42077=CARTESIAN_POINT ( 'NONE',  ( -6.811155457859999984, -79.33047884747199419, 6.825426861229999531 ) ) ;
#42082=FACE_OUTER_BOUND ( 'NONE', #6605, .T. ) ;
#42084=CARTESIAN_POINT ( 'NONE',  ( -10.25580049915999936, -77.27540488493299620, -4.414041361589999823 ) ) ;
#42087=CARTESIAN_POINT ( 'NONE',  ( 8.857396897828001769, -77.74332746776399006, -3.187116989308000026 ) ) ;
#42111=EDGE_CURVE ( 'NONE', #43554, #27720, #57080, .T. ) ;
#42123=CARTESIAN_POINT ( 'NONE',  ( 9.508122381440976767, -78.99355328149458444, -0.7695418330583383426 ) ) ;
#42127=CARTESIAN_POINT ( 'NONE',  ( -3.422957706972816094, -78.69494727339422013, -8.593410763649252715 ) ) ;
#42131=CARTESIAN_POINT ( 'NONE',  ( -5.563890944358950819, -80.18291473777019007, -9.489086410625162671 ) ) ;
#42147=CARTESIAN_POINT ( 'NONE',  ( -6.224830695901311550, -77.52669311147933229, -8.871307822741991700 ) ) ;
#42149=CARTESIAN_POINT ( 'NONE',  ( -7.508490145780001512, -78.91504759730605656, -8.005410190140000992 ) ) ;
#42156=CARTESIAN_POINT ( 'NONE',  ( 7.524111219894956903, -78.30076379627698202, -5.380381170981907601 ) ) ;
#42160=CARTESIAN_POINT ( 'NONE',  ( -8.012466620630000591, -78.43986703093798951, -5.343555802860000981 ) ) ;
#42176=CARTESIAN_POINT ( 'NONE',  ( 5.429444055910000344, -77.78519374448798374, -10.06097226053999982 ) ) ;
#42182=CARTESIAN_POINT ( 'NONE',  ( 9.630577183392999174, -79.09348223115100041, 1.628483183780000010 ) ) ;
#42194=AXIS2_PLACEMENT_3D ( 'NONE', #42907, #51774, #57337 ) ;
#42199=VECTOR ( 'NONE', #6931, 1000.000000000000000 ) ;
#42211=ORIENTED_EDGE ( 'NONE', *, *, #28484, .F. ) ;
#42214=CARTESIAN_POINT ( 'NONE',  ( 9.597472232836999240, -77.14168468004258727, -0.1661444564970999960 ) ) ;
#42220=CARTESIAN_POINT ( 'NONE',  ( 8.931146968900000260, -78.48816148727799202, -3.885139576175999920 ) ) ;
#42222=CARTESIAN_POINT ( 'NONE',  ( -9.146956334765603103, -77.74765838888041003, -6.250533269645468515 ) ) ;
#42223=B_SPLINE_CURVE_WITH_KNOTS ( 'NONE', 3,
 ( #55142, #37422, #46607, #32689 ),
 .UNSPECIFIED., .F., .F.,
 ( 4, 4 ),
 ( 0.000000000000000000, 1.000000000000000000 ),
 .UNSPECIFIED. ) ;
#42229=CARTESIAN_POINT ( 'NONE',  ( -1.210774177386837902, -77.98557709862954823, 9.250434933897750511 ) ) ;
#42231=CARTESIAN_POINT ( 'NONE',  ( -10.90760146693999921, -78.99931772544699982, -1.219937219691999974 ) ) ;
#42233=CARTESIAN_POINT ( 'NONE',  ( 4.238048199687000306, -79.74073595533198500, -8.569131342697998477 ) ) ;
#42236=ORIENTED_EDGE ( 'NONE', *, *, #46460, .F. ) ;
#42238=DIRECTION ( 'NONE',  ( 0.000000000000000000, 1.000000000000000000, 0.000000000000000000 ) ) ;
#42241=ADVANCED_FACE ( 'NONE', ( #35723 ), #40897, .F. ) ;
#42243=AXIS2_PLACEMENT_3D ( 'NONE', #6806, #11248, #16249 ) ;
#42251=CARTESIAN_POINT ( 'NONE',  ( -3.673276622528076629, -79.35225808950305293, 10.34286506330476740 ) ) ;
#42269=CARTESIAN_POINT ( 'NONE',  ( 8.193194696117055642, -77.38854057934830166, 4.293485181109531368 ) ) ;
#42270=CARTESIAN_POINT ( 'NONE',  ( -10.79754810892000094, -77.50716656116199488, -2.301543980133000211 ) ) ;
#42278=CARTESIAN_POINT ( 'NONE',  ( -10.88870934378999955, -79.47949549020498239, 1.874540603341000145 ) ) ;
#42304=CARTESIAN_POINT ( 'NONE',  ( 7.318097147681000614, -79.49262545241899147, -8.179820946710000484 ) ) ;
#42341=CARTESIAN_POINT ( 'NONE',  ( 6.931362644077239565, -78.29243420434676182, -6.125879640451257657 ) ) ;
#42343=ORIENTED_EDGE ( 'NONE', *, *, #34464, .T. ) ;
#42345=CARTESIAN_POINT ( 'NONE',  ( -9.012377310937894848, -77.58185562474179164, 2.097317376807573019 ) ) ;
#42349=CARTESIAN_POINT ( 'NONE',  ( -9.685922776715001348, -77.20466883505099531, 0.5943755449006998814 ) ) ;
#42363=CIRCLE ( 'NONE', #10323, 10.50000000000000000 ) ;
#42373=CARTESIAN_POINT ( 'NONE',  ( 8.558937808803998237, -79.68115074656799379, 4.441044281071000022 ) ) ;
#42379=CARTESIAN_POINT ( 'NONE',  ( -7.349905019660000427, -77.67524080624798444, 8.405004550887998249 ) ) ;
#42383=CARTESIAN_POINT ( 'NONE',  ( -5.511117113485999752, -78.59604234163299452, -7.631433854063000233 ) ) ;
#42390=FACE_OUTER_BOUND ( 'NONE', #10445, .T. ) ;
#42392=ORIENTED_EDGE ( 'NONE', *, *, #39224, .F. ) ;
#42414=CIRCLE ( 'NONE', #2835, 4.299999999999999822 ) ;
#42419=CARTESIAN_POINT ( 'NONE',  ( 5.091895231007000255, -78.58104366793577356, 8.260951054388000259 ) ) ;
#42425=CARTESIAN_POINT ( 'NONE',  ( -7.847716748518878127, -78.64456789939313808, -4.896326238464910219 ) ) ;
#42428=CARTESIAN_POINT ( 'NONE',  ( -5.608494644813585062, -80.18255198204721523, -9.462727630867055595 ) ) ;
#42444=CARTESIAN_POINT ( 'NONE',  ( 8.601671466536686239, -78.14867843084759613, -6.555704085095740652 ) ) ;
#42446=CARTESIAN_POINT ( 'NONE',  ( 0.9090372547675998893, -78.71840111697744646, 10.93790052300000148 ) ) ;
#42451=DIRECTION ( 'NONE',  ( 0.000000000000000000, 1.000000000000000000, 0.000000000000000000 ) ) ;
#42455=CARTESIAN_POINT ( 'NONE',  ( 1.492456682423999981, -77.46642875802798756, -9.624565956529000488 ) ) ;
#42466=CARTESIAN_POINT ( 'NONE',  ( -7.241278761924999863, -80.25027481282198494, -9.001616806789000336 ) ) ;
#42469=CARTESIAN_POINT ( 'NONE',  ( 3.794578590805999685, -77.90474154703099430, 10.66739949363999962 ) ) ;
#42475=CARTESIAN_POINT ( 'NONE',  ( 9.630577183392999174, -79.27363800027249852, 1.628483183780000010 ) ) ;
#42484=CARTESIAN_POINT ( 'NONE',  ( 9.250000000000000000, -78.34999999999999432, 0.000000000000000000 ) ) ;
#42487=CARTESIAN_POINT ( 'NONE',  ( 9.444950681165998674, -76.84924050810879237, -2.026199312500999827 ) ) ;
#42489=CARTESIAN_POINT ( 'NONE',  ( -10.99999999999999822, -79.61041666666666572, -1.439896632895323325 ) ) ;
#42492=CARTESIAN_POINT ( 'NONE',  ( 7.483407197968000801, -77.19999999999998863, -5.437013583705000208 ) ) ;
#42502=CARTESIAN_POINT ( 'NONE',  ( -8.355323416140999271, -77.28668387500499648, 4.941688539782999712 ) ) ;
#42507=CARTESIAN_POINT ( 'NONE',  ( -5.370832524224000259, -77.69229427166699509, 8.124890996387998499 ) ) ;
#42510=CARTESIAN_POINT ( 'NONE',  ( -4.043136777828878259, -77.79531677776081722, -10.31450538517582416 ) ) ;
#42520=CARTESIAN_POINT ( 'NONE',  ( -10.47663719470709331, -80.07552825402615326, 3.352253582661057774 ) ) ;
#42521=CARTESIAN_POINT ( 'NONE',  ( 7.655485751584000020, -79.77808361358998468, -5.725784120545999833 ) ) ;
#42523=CARTESIAN_POINT ( 'NONE',  ( 5.684557159767975598, -79.17708333333330017, -7.396918292183157106 ) ) ;
#42539=CARTESIAN_POINT ( 'NONE',  ( 3.366547962069000199, -79.36254827890498120, -9.168809063548000182 ) ) ;
#42557=CARTESIAN_POINT ( 'NONE',  ( 9.184859914837900874, -77.35958091549174753, 1.096818293188132065 ) ) ;
#42566=CARTESIAN_POINT ( 'NONE',  ( 4.665505440478000310, -78.83337134055398110, 10.01553556391000122 ) ) ;
#42583=CARTESIAN_POINT ( 'NONE',  ( 4.996366032364999654, -78.47410532222798452, 8.105967104710000370 ) ) ;
#42596=CARTESIAN_POINT ( 'NONE',  ( -10.81649518602000093, -79.35628189776099362, 1.862108609190000097 ) ) ;
#42604=CARTESIAN_POINT ( 'NONE',  ( -2.421167930323352646, -78.10416666666665719, -9.009247259181913492 ) ) ;
#42606=CARTESIAN_POINT ( 'NONE',  ( 9.951586773259000651, -79.39035858408298907, -5.281558014135000256 ) ) ;
#42608=FACE_BOUND ( 'NONE', #18735, .T. ) ;
#42615=DIRECTION ( 'NONE',  ( 0.000000000000000000, 1.000000000000000000, 0.000000000000000000 ) ) ;
#42620=CARTESIAN_POINT ( 'NONE',  ( 9.499941120207004985, -79.99343229508609454, -0.7840560289833928831 ) ) ;
#42632=CARTESIAN_POINT ( 'NONE',  ( -9.150401306387172085, -77.58846111580191973, 1.353620980104426996 ) ) ;
#42635=CARTESIAN_POINT ( 'NONE',  ( -7.707166124622999881, -77.26151649330898863, -5.896629607976000109 ) ) ;
#42640=FACE_BOUND ( 'NONE', #15865, .T. ) ;
#42646=CARTESIAN_POINT ( 'NONE',  ( -9.484300247301399978, -80.30416666667800030, -5.483079476845273525 ) ) ;
#42651=CARTESIAN_POINT ( 'NONE',  ( -8.839214553731000734, -80.04551656954198791, -6.848292123026999967 ) ) ;
#42654=ORIENTED_EDGE ( 'NONE', *, *, #26031, .T. ) ;
#42659=CARTESIAN_POINT ( 'NONE',  ( 9.474537194627000503, -79.71580382909299090, 1.059975283156000092 ) ) ;
#42666=CARTESIAN_POINT ( 'NONE',  ( 9.146564807811000009, -77.57451461849198893, -6.016234306896000028 ) ) ;
#42670=CARTESIAN_POINT ( 'NONE',  ( -6.563619111649000359, -78.08441341731199259, -6.747599474233999750 ) ) ;
#42678=ADVANCED_BREP_SHAPE_REPRESENTATION ( '', ( #55564, #43526 ), #9600 ) ;
#42694=EDGE_LOOP ( 'NONE', ( #27312, #50515, #37296 ) ) ;
#42711=CARTESIAN_POINT ( 'NONE',  ( -2.417559983778709842, -78.70412069868730498, -8.933467346123652675 ) ) ;
#42732=CARTESIAN_POINT ( 'NONE',  ( 10.83790964778171073, -77.70003328245064722, -0.06560966762940606545 ) ) ;
#42739=CARTESIAN_POINT ( 'NONE',  ( 8.953311532445939136, -78.32993639350726767, -2.326867093362477323 ) ) ;
#42743=CARTESIAN_POINT ( 'NONE',  ( -7.872620573787999732, -77.77909087844599867, 5.734242845189999827 ) ) ;
#42748=EDGE_LOOP ( 'NONE', ( #5466, #26388, #43418, #6592 ) ) ;
#42758=CARTESIAN_POINT ( 'NONE',  ( 9.248082609065999549, -77.75800271236998640, -6.531860890005000364 ) ) ;
#42768=CARTESIAN_POINT ( 'NONE',  ( -4.465297566879000257, -80.16279685233251939, 8.686876450551999085 ) ) ;
#42769=ORIENTED_EDGE ( 'NONE', *, *, #4555, .F. ) ;
#42776=CARTESIAN_POINT ( 'NONE',  ( -9.250000000000000000, -77.99999999999998579, 0.000000000000000000 ) ) ;
#42779=CARTESIAN_POINT ( 'NONE',  ( 6.760013919724077169, -79.77708333333333712, -8.796335266379973206 ) ) ;
#42782=CARTESIAN_POINT ( 'NONE',  ( 2.421167930323313566, -77.85416666666664298, 9.009247259181924150 ) ) ;
#42799=CARTESIAN_POINT ( 'NONE',  ( -7.872620573787999732, -77.72071810079599175, 5.734242845189999827 ) ) ;
#42806=CARTESIAN_POINT ( 'NONE',  ( 1.155251330895799677, -79.11532408967735819, 9.449995398207709840 ) ) ;
#42810=CARTESIAN_POINT ( 'NONE',  ( 8.486433606932997975, -79.36725937275299714, 4.401307641916000435 ) ) ;
#42812=CARTESIAN_POINT ( 'NONE',  ( 1.210822168571075386, -79.13541666666664298, -9.249999999999996447 ) ) ;
#42817=ADVANCED_FACE ( 'NONE', ( #52520 ), #43638, .T. ) ;
#42823=FACE_OUTER_BOUND ( 'NONE', #38323, .T. ) ;
#42827=ADVANCED_FACE ( 'NONE', ( #20362 ), #38647, .F. ) ;
#42829=CARTESIAN_POINT ( 'NONE',  ( -9.687172913667000174, -79.71974751974299522, -1.248753675804000096 ) ) ;
#42831=ORIENTED_EDGE ( 'NONE', *, *, #35921, .T. ) ;
#42839=ADVANCED_FACE ( 'NONE', ( #48109 ), #36085, .F. ) ;
#42847=EDGE_LOOP ( 'NONE', ( #23049, #9063, #21506, #38879 ) ) ;
#42848=CARTESIAN_POINT ( 'NONE',  ( 4.204440787238356236, -77.26257104358636241, -8.239219949706841462 ) ) ;
#42849=CARTESIAN_POINT ( 'NONE',  ( 4.799999999787999627, -74.99999999978798826, 2.226279959716000065E-09 ) ) ;
#42857=CARTESIAN_POINT ( 'NONE',  ( -4.385047663734000345, -79.83700506441199707, 10.02292886995000032 ) ) ;
#42873=CARTESIAN_POINT ( 'NONE',  ( 8.779834778627000347, -77.35854790367199030, 3.394951511978999914 ) ) ;
#42876=DIRECTION ( 'NONE',  ( 0.000000000000000000, 1.000000000000000000, 0.000000000000000000 ) ) ;
#42882=CIRCLE ( 'NONE', #57940, 9.549999999999998934 ) ;
#42884=LINE ( 'NONE', #10134, #1305 ) ;
#42886=CARTESIAN_POINT ( 'NONE',  ( -3.673218652927999539, -79.27200483476298132, 10.34270183798999909 ) ) ;
#42895=CARTESIAN_POINT ( 'NONE',  ( -4.391024480082000636, -78.77232678876399063, -10.37534762698999913 ) ) ;
#42907=CARTESIAN_POINT ( 'NONE',  ( 0.000000000000000000, -76.39999999999999147, 0.000000000000000000 ) ) ;
#42920=CARTESIAN_POINT ( 'NONE',  ( 0.03245390597466887156, -78.22536965980819446, -9.249895125673516461 ) ) ;
#42924=ORIENTED_EDGE ( 'NONE', *, *, #46460, .T. ) ;
#42925=CARTESIAN_POINT ( 'NONE',  ( -8.799679198670379066, -77.57509512262019769, 2.850925869413578173 ) ) ;
#42928=CARTESIAN_POINT ( 'NONE',  ( 1.260641617779999946, -77.69478446506998637, 9.621927669549000584 ) ) ;
#42949=CARTESIAN_POINT ( 'NONE',  ( 0.000000000000000000, -76.30000000005068728, 0.000000000000000000 ) ) ;
#42951=CONICAL_SURFACE ( 'NONE', #14611, 5.249999999862000166, 0.7853981633972997312 ) ;
#42955=CARTESIAN_POINT ( 'NONE',  ( 4.793796853326000473, -80.12492104470399568, -7.994680211816000970 ) ) ;
#42961=CARTESIAN_POINT ( 'NONE',  ( -9.642170440073000393, -77.83155199647998757, 5.184908120652999663 ) ) ;
#42971=DIRECTION ( 'NONE',  ( 0.000000000000000000, -1.000000000000000000, 0.000000000000000000 ) ) ;
#42976=VERTEX_POINT ( 'NONE', #39387 ) ;
#42977=ADVANCED_FACE ( 'NONE', ( #52675 ), #52107, .T. ) ;
#42979=ORIENTED_EDGE ( 'NONE', *, *, #41429, .F. ) ;
#43000=CARTESIAN_POINT ( 'NONE',  ( -8.707890922082185625, -79.81324511864698934, 4.310198284464144436 ) ) ;
#43003=CARTESIAN_POINT ( 'NONE',  ( -7.690083695982694145, -78.64705780292665338, -5.141504542771214936 ) ) ;
#43022=CARTESIAN_POINT ( 'NONE',  ( 6.123452257235864060, -77.62355967761020281, -8.862192408124634824 ) ) ;
#43023=CARTESIAN_POINT ( 'NONE',  ( 3.747727186550270595, -78.25250684441732574, -10.42547443909607097 ) ) ;
#43024=CARTESIAN_POINT ( 'NONE',  ( -9.331191635713286914, -77.45159008118203303, -0.1973268560526538207 ) ) ;
#43026=ORIENTED_EDGE ( 'NONE', *, *, #32128, .F. ) ;
#43032=CARTESIAN_POINT ( 'NONE',  ( -5.310864497047000476, -77.81454279010098674, 8.034172531070000289 ) ) ;
#43040=ORIENTED_EDGE ( 'NONE', *, *, #10495, .T. ) ;
#43042=CARTESIAN_POINT ( 'NONE',  ( 7.267180141948999861, -79.12481710499199039, 8.322618964701998578 ) ) ;
#43047=CARTESIAN_POINT ( 'NONE',  ( -8.870296161681000768, -77.67513961849198267, -7.212480266026999765 ) ) ;
#43049=ORIENTED_EDGE ( 'NONE', *, *, #41212, .F. ) ;
#43052=FACE_OUTER_BOUND ( 'NONE', #22483, .T. ) ;
#43053=CARTESIAN_POINT ( 'NONE',  ( -8.448510849392999233, -79.46847394982049195, 4.901364000006999788 ) ) ;
#43055=FACE_OUTER_BOUND ( 'NONE', #9362, .T. ) ;
#43072=DIRECTION ( 'NONE',  ( 0.7071067811865969777, -0.7071067811864980568, -1.725239202167994796E-11 ) ) ;
#43074=ADVANCED_FACE ( 'NONE', ( #2513 ), #30377, .T. ) ;
#43078=CARTESIAN_POINT ( 'NONE',  ( 0.000000000000000000, -81.79999999999998295, 0.000000000000000000 ) ) ;
#43091=CARTESIAN_POINT ( 'NONE',  ( 4.202230864774000096, -78.43131382901999871, -8.786407198941001084 ) ) ;
#43097=EDGE_CURVE ( 'NONE', #9068, #43122, #43530, .T. ) ;
#43100=CARTESIAN_POINT ( 'NONE',  ( -9.498650009403984740, -79.25105001372490676, -0.1253404953979189163 ) ) ;
#43103=CARTESIAN_POINT ( 'NONE',  ( -10.53088506292314008, -80.07679749114764434, 3.178975094537701107 ) ) ;
#43104=CARTESIAN_POINT ( 'NONE',  ( -9.473445107265000331, -79.06847810668898546, 1.282537450098000020 ) ) ;
#43106=CARTESIAN_POINT ( 'NONE',  ( -7.396918292183162436, -79.05208333333331439, -5.684557159767966716 ) ) ;
#43116=DIRECTION ( 'NONE',  ( 0.000000000000000000, 1.000000000000000000, 0.000000000000000000 ) ) ;
#43118=CARTESIAN_POINT ( 'NONE',  ( 6.613044192456900561, -79.77364340449305757, 8.759878235630585763 ) ) ;
#43119=CARTESIAN_POINT ( 'NONE',  ( 9.523132023602000729, -79.96870456638698954, 1.108936319727999997 ) ) ;
#43122=VERTEX_POINT ( 'NONE', #31669 ) ;
#43126=VECTOR ( 'NONE', #50601, 1000.000000000000000 ) ;
#43140=ORIENTED_EDGE ( 'NONE', *, *, #1079, .F. ) ;
#43141=CARTESIAN_POINT ( 'NONE',  ( 6.980683240476435181, -77.29306357213712886, -6.070245327366276200 ) ) ;
#43150=CARTESIAN_POINT ( 'NONE',  ( 6.762881825298999949, -79.17047959254598766, -8.737352176957999816 ) ) ;
#43165=CARTESIAN_POINT ( 'NONE',  ( 5.315453493860999856, -78.81519127177598705, -7.900401732693999257 ) ) ;
#43171=ORIENTED_EDGE ( 'NONE', *, *, #55762, .F. ) ;
#43174=CIRCLE ( 'NONE', #42194, 10.69999999999999929 ) ;
#43177=CARTESIAN_POINT ( 'NONE',  ( -0.6514878906251000412, -79.74957485841899540, 10.95625855609000077 ) ) ;
#43188=CARTESIAN_POINT ( 'NONE',  ( -9.332307860560000279, -78.63186501710099208, 6.311653060910999535 ) ) ;
#43197=ORIENTED_EDGE ( 'NONE', *, *, #38746, .T. ) ;
#43209=CARTESIAN_POINT ( 'NONE',  ( -4.233603723169751198, -77.51295453581894890, 8.224218726036120586 ) ) ;
#43212=CARTESIAN_POINT ( 'NONE',  ( -5.681372509047000641, -78.40538019329399333, -7.867192369580999767 ) ) ;
#43218=CARTESIAN_POINT ( 'NONE',  ( -3.493617039247999934, -80.52908066372398821, -10.33892454317000187 ) ) ;
#43237=CARTESIAN_POINT ( 'NONE',  ( -9.283978793531677098, -77.14367230500779726, -1.155228012124903891 ) ) ;
#43240=CARTESIAN_POINT ( 'NONE',  ( 2.041361922787999994, -79.53503745527798685, -9.423965843603999915 ) ) ;
#43242=CARTESIAN_POINT ( 'NONE',  ( 2.056966010086916707, -79.49179605286448691, -9.496002254240691443 ) ) ;
#43249=CARTESIAN_POINT ( 'NONE',  ( -10.42144728442999835, -77.34603694916899030, 3.353826678397000105 ) ) ;
#43255=CARTESIAN_POINT ( 'NONE',  ( -8.324924863653999196, -77.22734602334399767, 4.923709561474999497 ) ) ;
#43263=LINE ( 'NONE', #30529, #29350 ) ;
#43285=CARTESIAN_POINT ( 'NONE',  ( -9.478938303170380664, -77.25897152220545649, -1.070660778503142785 ) ) ;
#43287=B_SPLINE_CURVE_WITH_KNOTS ( 'NONE', 3,
 ( #48023, #39134, #20839, #56861, #57146, #52434, #24697, #55997, #7842, #52150, #48304, #43289, #52722, #47734, #11417, #15838, #51578, #2843 ),
 .UNSPECIFIED., .F., .F.,
 ( 4, 2, 2, 2, 2, 2, 2, 2, 4 ),
 ( 0.000000000000000000, 0.1250000000000000278, 0.2500000000000000000, 0.3750000000000001110, 0.5000000000000001110, 0.6250000000000001110, 0.7500000000000002220, 0.8750000000000001110, 1.000000000000000000 ),
 .UNSPECIFIED. ) ;
#43289=CARTESIAN_POINT ( 'NONE',  ( 5.539808784079868431, -78.53333333333334565, 9.611650271896850839 ) ) ;
#43290=CARTESIAN_POINT ( 'NONE',  ( -8.730066282802408040, -78.62683183961394207, -3.057454265489415679 ) ) ;
#43292=CARTESIAN_POINT ( 'NONE',  ( -10.80277078588560968, -80.11543121848195881, -2.112588677537822424 ) ) ;
#43308=CARTESIAN_POINT ( 'NONE',  ( 7.174506471390958318, -78.28110187774559847, -8.441707957340311097 ) ) ;
#43318=CARTESIAN_POINT ( 'NONE',  ( -1.160011803644999784, -79.07221935430098370, -9.451177169703999681 ) ) ;
#43323=CARTESIAN_POINT ( 'NONE',  ( 9.249483092228999226, -78.85084128437098627, 0.09778817195952001218 ) ) ;
#43327=CARTESIAN_POINT ( 'NONE',  ( 10.52250585264000016, -78.59875340478899375, -2.994108701640999737 ) ) ;
#43329=CARTESIAN_POINT ( 'NONE',  ( -7.155892224914999211, -79.94076805110799455, -8.639911640714998953 ) ) ;
#43336=CARTESIAN_POINT ( 'NONE',  ( -7.545891804452000251, -80.07541666714000428, 6.201630566990999682 ) ) ;
#43339=VERTEX_POINT ( 'NONE', #41425 ) ;
#43367=CARTESIAN_POINT ( 'NONE',  ( 9.164371241867000251, -77.49332746776399006, -3.297574176498999865 ) ) ;
#43368=DIRECTION ( 'NONE',  ( 0.000000000000000000, 1.000000000000000000, 0.000000000000000000 ) ) ;
#43375=CARTESIAN_POINT ( 'NONE',  ( -8.848325884602834535, -79.28052203371991880, -3.567648052095428568 ) ) ;
#43377=CARTESIAN_POINT ( 'NONE',  ( -2.903215668995137388, -80.00000000000000000, -8.988737031711306003 ) ) ;
#43380=CARTESIAN_POINT ( 'NONE',  ( 9.602680411058999610, -78.97214363870799048, 1.857383748591999950 ) ) ;
#43382=CARTESIAN_POINT ( 'NONE',  ( -5.684557159767956058, -79.07291666666664298, -7.396918292183169541 ) ) ;
#43396=CARTESIAN_POINT ( 'NONE',  ( -9.699833017908000343, -79.20018498761599801, 1.146274062705999963 ) ) ;
#43401=B_SPLINE_CURVE_WITH_KNOTS ( 'NONE', 3,
 ( #6614, #16924, #20772, #39354 ),
 .UNSPECIFIED., .F., .F.,
 ( 4, 4 ),
 ( 0.000000000000000000, 1.000000000000000000 ),
 .UNSPECIFIED. ) ;
#43408=DIRECTION ( 'NONE',  ( 0.000000000000000000, -1.000000000000000000, 1.567264836428999919E-13 ) ) ;
#43415=CARTESIAN_POINT ( 'NONE',  ( 3.107115389279428985, -79.94787407444857763, 8.714688932331064564 ) ) ;
#43418=ORIENTED_EDGE ( 'NONE', *, *, #38010, .F. ) ;
#43419=CARTESIAN_POINT ( 'NONE',  ( -11.25716098398999954, -78.62401457012799710, -0.4530573336216000002 ) ) ;
#43420=CARTESIAN_POINT ( 'NONE',  ( 7.509078405248583721, -77.30045981524069987, -5.401436182427549859 ) ) ;
#43431=CARTESIAN_POINT ( 'NONE',  ( 3.197825632618000125, -79.84469609652998656, 10.57600109144000022 ) ) ;
#43432=CARTESIAN_POINT ( 'NONE',  ( 0.000000000000000000, -74.99999999999998579, 0.000000000000000000 ) ) ;
#43446=CARTESIAN_POINT ( 'NONE',  ( 4.108390852610000366, -78.30356234745399036, -8.590197950816000017 ) ) ;
#43460=CARTESIAN_POINT ( 'NONE',  ( 3.915498778898000687, -79.21582012609798085, 10.25343288338999947 ) ) ;
#43465=CARTESIAN_POINT ( 'NONE',  ( -11.00000000000000533, -79.69292008887531154, 0.9786566581930159492 ) ) ;
#43472=CARTESIAN_POINT ( 'NONE',  ( 4.757299607910999484, -78.51949559976999637, 10.21259197296000032 ) ) ;
#43478=EDGE_CURVE ( 'NONE', #26583, #47291, #21304, .T. ) ;
#43495=CARTESIAN_POINT ( 'NONE',  ( -7.272255731327333272, -77.54700831801773120, 5.716658912645681490 ) ) ;
#43497=CARTESIAN_POINT ( 'NONE',  ( 5.341789944771999643, -77.64435487080298515, 9.661750877468000098 ) ) ;
#43500=CARTESIAN_POINT ( 'NONE',  ( -6.473047519705999342, -78.26326104764899583, 7.229824698717000508 ) ) ;
#43504=CARTESIAN_POINT ( 'NONE',  ( -1.870137171474999915, -79.92126121676598416, -11.09839649295000008 ) ) ;
#43522=CARTESIAN_POINT ( 'NONE',  ( 7.483407197968000801, -77.19999999999998863, -5.437013583705000208 ) ) ;
#43526=AXIS2_PLACEMENT_3D ( 'NONE', #45889, #10156, #14564 ) ;
#43527=CARTESIAN_POINT ( 'NONE',  ( 9.316358549523000576, -79.28289437949098328, 1.425245117218999935 ) ) ;
#43530=LINE ( 'NONE', #16667, #17201 ) ;
#43533=CARTESIAN_POINT ( 'NONE',  ( 10.84676810008999936, -77.63163403582298372, 1.484029919422999999 ) ) ;
#43539=CARTESIAN_POINT ( 'NONE',  ( 5.684557159767968493, -78.32291666666665719, 7.396918292183160659 ) ) ;
#43554=VERTEX_POINT ( 'NONE', #11306 ) ;
#43562=CARTESIAN_POINT ( 'NONE',  ( -9.250000000000001776, -79.51041666666667140, -1.210822168571065616 ) ) ;
#43571=CARTESIAN_POINT ( 'NONE',  ( -9.161237776338555960, -77.27573413481378850, -3.065692136626856801 ) ) ;
#43578=CARTESIAN_POINT ( 'NONE',  ( -9.250001407686912813, -78.60108681346355297, -0.1266027648973193087 ) ) ;
#43581=CARTESIAN_POINT ( 'NONE',  ( -10.89834548151206306, -80.11100334882785035, -1.491191014881230847 ) ) ;
#43608=CARTESIAN_POINT ( 'NONE',  ( 9.508660861234000450, -78.70270957562398451, -0.5057122284909000287 ) ) ;
#43613=CARTESIAN_POINT ( 'NONE',  ( 9.178424375319440998, -78.86168501646835693, 1.303869873657260481 ) ) ;
#43616=CARTESIAN_POINT ( 'NONE',  ( 8.291742182491999458, -78.17736808979898910, 7.136865503491999441 ) ) ;
#43618=CARTESIAN_POINT ( 'NONE',  ( -11.27530493984999893, -79.72949423886399245, 1.941616567897000101 ) ) ;
#43628=CARTESIAN_POINT ( 'NONE',  ( 9.647254834573999460, -80.48752343491251793, -1.526580663425000095 ) ) ;
#43630=VERTEX_POINT ( 'NONE', #26582 ) ;
#43638=CONICAL_SURFACE ( 'NONE', #19119, 4.899999999795999983, 0.7853981633972997312 ) ;
#43644=CARTESIAN_POINT ( 'NONE',  ( 9.073237612486709125, -78.83448602473089295, -1.799436367680483873 ) ) ;
#43647=CARTESIAN_POINT ( 'NONE',  ( 1.478685717397393518, -77.04374999986741557, -9.318529382992288390 ) ) ;
#43649=DIRECTION ( 'NONE',  ( 0.000000000000000000, 1.000000000000000000, 0.000000000000000000 ) ) ;
#43651=CARTESIAN_POINT ( 'NONE',  ( 0.000000000000000000, -76.29999999995945359, 0.000000000000000000 ) ) ;
#43657=CIRCLE ( 'NONE', #18219, 1.000000000000000000 ) ;
#43659=EDGE_CURVE ( 'NONE', #45010, #56496, #24939, .T. ) ;
#43667=VERTEX_POINT ( 'NONE', #39599 ) ;
#43671=CARTESIAN_POINT ( 'NONE',  ( -9.495705824214729418, -79.25230558782985213, -0.2751968363797689388 ) ) ;
#43672=CARTESIAN_POINT ( 'NONE',  ( -6.603396513061970730, -79.99999999999998579, -6.628355741337830231 ) ) ;
#43675=CARTESIAN_POINT ( 'NONE',  ( 4.384927929828000615, -79.93236317768199228, -8.866115152190999993 ) ) ;
#43677=CARTESIAN_POINT ( 'NONE',  ( -11.00000000000000000, -78.59999999999999432, 0.000000000000000000 ) ) ;
#43685=CARTESIAN_POINT ( 'NONE',  ( -9.549999999999998934, -79.99999999999998579, 0.000000000000000000 ) ) ;
#43691=CARTESIAN_POINT ( 'NONE',  ( 9.179330843189999811, -77.22671943548499485, 6.243840602170999787 ) ) ;
#43697=CARTESIAN_POINT ( 'NONE',  ( 8.985706068735000329, -79.42749359542099796, -3.828549499589000149 ) ) ;
#43704=CARTESIAN_POINT ( 'NONE',  ( -11.00000000000000711, -77.68958333333333144, 1.439896632895276696 ) ) ;
#43712=CARTESIAN_POINT ( 'NONE',  ( 1.314364188573257319, -79.96416879256437937, 9.155857543867112369 ) ) ;
#43718=CARTESIAN_POINT ( 'NONE',  ( -2.226613147434000073, -78.51164515279698719, 11.04405396508999893 ) ) ;
#43719=CARTESIAN_POINT ( 'NONE',  ( 6.769035029585133145, -77.29037018802434034, -6.304485289422735228 ) ) ;
#43726=CARTESIAN_POINT ( 'NONE',  ( 5.539808784079867543, -78.43333333333333712, 9.611650271896852615 ) ) ;
#43729=CARTESIAN_POINT ( 'NONE',  ( -2.977158780993999887, -78.95343179000198575, 10.75305190397999944 ) ) ;
#43743=CARTESIAN_POINT ( 'NONE',  ( 9.480930971721999612, -78.90046275916299123, 0.8843128721991000418 ) ) ;
#43748=ORIENTED_EDGE ( 'NONE', *, *, #33558, .F. ) ;
#43753=CARTESIAN_POINT ( 'NONE',  ( -9.091539081997000338, -78.82252716544098803, 6.148815634104000338 ) ) ;
#43754=CARTESIAN_POINT ( 'NONE',  ( 1.417398248412324424, -80.36536458333203825, 10.83463541661525831 ) ) ;
#43763=CARTESIAN_POINT ( 'NONE',  ( 5.539808784079868431, -78.03333333333331723, 9.611650271896850839 ) ) ;
#43765=CARTESIAN_POINT ( 'NONE',  ( -8.774483958462999666, -78.19007837989597931, 6.892026619272999532 ) ) ;
#43771=CARTESIAN_POINT ( 'NONE',  ( -9.250000000000000000, -79.99999999999998579, 2.662757480928999879E-14 ) ) ;
#43777=EDGE_CURVE ( 'NONE', #1033, #42976, #21113, .T. ) ;
#43779=DIRECTION ( 'NONE',  ( 0.000000000000000000, -1.000000000000000000, 0.000000000000000000 ) ) ;
#43783=SHAPE_DEFINITION_REPRESENTATION ( #33367, #46016 ) ;
#43785=CARTESIAN_POINT ( 'NONE',  ( 0.01737526028195334263, -78.22524228320165207, -9.249935897884874691 ) ) ;
#43791=CARTESIAN_POINT ( 'NONE',  ( -4.204260939637024741, -77.51267571432379100, 8.239242333927206730 ) ) ;
#43792=CARTESIAN_POINT ( 'NONE',  ( -5.876696946710000091, -77.38987720147999028, -9.346046374399000101 ) ) ;
#43797=CARTESIAN_POINT ( 'NONE',  ( 5.927986824875999261, -78.00744658548798327, -7.683077610609999830 ) ) ;
#43802=CARTESIAN_POINT ( 'NONE',  ( 3.942135768300999654, -79.96302238210400049, -10.54187931140000067 ) ) ;
#43806=ORIENTED_EDGE ( 'NONE', *, *, #55117, .T. ) ;
#43814=CARTESIAN_POINT ( 'NONE',  ( -9.567284400036999870, -80.01536253608898619, 5.522558287099000651 ) ) ;
#43818=CARTESIAN_POINT ( 'NONE',  ( -8.796335266380014062, -80.14791666668804737, 6.760013919724027431 ) ) ;
#43824=CARTESIAN_POINT ( 'NONE',  ( 4.739049146600000206, -80.18879678548698564, -7.903376716697000148 ) ) ;
#43826=CARTESIAN_POINT ( 'NONE',  ( 4.401050137192186185, -77.19999999999998863, 9.873231036884021705 ) ) ;
#43839=CARTESIAN_POINT ( 'NONE',  ( 2.632967082928999947, -77.06260562980078532, 9.306700570505000769 ) ) ;
#43862=CARTESIAN_POINT ( 'NONE',  ( -4.658475568430814562, -79.58333333333330017, -8.082524092276884176 ) ) ;
#43865=FACE_OUTER_BOUND ( 'NONE', #16902, .T. ) ;
#43874=CARTESIAN_POINT ( 'NONE',  ( -8.743226456218904374, -78.62649317345338318, -3.019661628328330405 ) ) ;
#43901=CARTESIAN_POINT ( 'NONE',  ( -5.120069445942999842, -77.47345684055298420, -8.157089945504001349 ) ) ;
#43909=CARTESIAN_POINT ( 'NONE',  ( 8.185910223524000884, -78.06499867246799340, -6.914387615432000977 ) ) ;
#43913=CARTESIAN_POINT ( 'NONE',  ( -1.629734310963000032, -80.48366320050999434, -10.59064910002000026 ) ) ;
#43921=CYLINDRICAL_SURFACE ( 'NONE', #36523, 11.00000000000000000 ) ;
#43930=CARTESIAN_POINT ( 'NONE',  ( 9.041762528755288741, -78.83306936774171447, -1.957752293751276351 ) ) ;
#43949=CARTESIAN_POINT ( 'NONE',  ( -10.49999999996000000, -76.19999999995870610, -1.566656233679999990E-09 ) ) ;
#43954=EDGE_LOOP ( 'NONE', ( #40113, #19088, #54500, #29135 ) ) ;
#43959=CARTESIAN_POINT ( 'NONE',  ( 7.495001602003393160, -79.05287805411308000, 5.870005187018274562 ) ) ;
#43961=CARTESIAN_POINT ( 'NONE',  ( -1.439896632895359962, -78.98541666666666572, 10.99999999999999645 ) ) ;
#43963=CARTESIAN_POINT ( 'NONE',  ( 9.780341196751001220, -79.45766319606099160, 0.08914745397413999239 ) ) ;
#43969=CYLINDRICAL_SURFACE ( 'NONE', #48811, 1.000000000000000000 ) ;
#43973=VERTEX_POINT ( 'NONE', #49570 ) ;
#43978=CARTESIAN_POINT ( 'NONE',  ( 9.647254834573999460, -80.06766197889000125, -1.526580663425000095 ) ) ;
#43982=CYLINDRICAL_SURFACE ( 'NONE', #426, 11.00000000000000000 ) ;
#43987=CARTESIAN_POINT ( 'NONE',  ( 10.71369944335147117, -77.47083333333331723, 2.879226727952105769 ) ) ;
#43997=CARTESIAN_POINT ( 'NONE',  ( 1.445445956927814191, -79.96300696816564368, 9.136058195600192278 ) ) ;
#44000=ORIENTED_EDGE ( 'NONE', *, *, #33798, .T. ) ;
#44001=CARTESIAN_POINT ( 'NONE',  ( 6.344372811184452843, -77.28524184710113332, -6.736967749196288047 ) ) ;
#44008=LINE ( 'NONE', #21562, #40407 ) ;
#44010=CARTESIAN_POINT ( 'NONE',  ( 10.48730647577000141, -78.27921528601798684, -3.808884262352000061 ) ) ;
#44023=CARTESIAN_POINT ( 'NONE',  ( 7.830665294675000609, -78.90749084168798788, -5.606588350762000239 ) ) ;
#44028=ORIENTED_EDGE ( 'NONE', *, *, #29153, .F. ) ;
#44035=CARTESIAN_POINT ( 'NONE',  ( 8.867070753125000593, -78.62999890211698073, -6.468312982590000537 ) ) ;
#44036=CARTESIAN_POINT ( 'NONE',  ( 10.60938144191372068, -80.30677083333185351, 2.852067028529588377 ) ) ;
#44043=CARTESIAN_POINT ( 'NONE',  ( -10.71369944335147117, -77.62083333333335133, -2.879226727952084453 ) ) ;
#44047=CARTESIAN_POINT ( 'NONE',  ( 10.92153517268999963, -78.97666430121098813, -2.282908042080999955 ) ) ;
#44055=CARTESIAN_POINT ( 'NONE',  ( 0.000000000000000000, -76.89999999999999147, 0.000000000000000000 ) ) ;
#44061=CARTESIAN_POINT ( 'NONE',  ( -2.654829587612529629, -79.64748934874999975, 9.152484904945515254 ) ) ;
#44066=CARTESIAN_POINT ( 'NONE',  ( -6.537588131481950171, -78.16270971461653971, -6.543733269810712905 ) ) ;
#44068=VERTEX_POINT ( 'NONE', #4976 ) ;
#44070=CARTESIAN_POINT ( 'NONE',  ( -6.946610297121736721, -77.54270072396643343, 6.109334087155939841 ) ) ;
#44071=CARTESIAN_POINT ( 'NONE',  ( -1.776188306762000124, -77.48198983581598043, -10.89629776253999971 ) ) ;
#44075=CARTESIAN_POINT ( 'NONE',  ( -4.814859605045999302, -78.74646614284199586, 8.425427962446999430 ) ) ;
#44078=CARTESIAN_POINT ( 'NONE',  ( -11.11771682179999843, -80.35741463048398714, 1.751409206030000165 ) ) ;
#44082=CARTESIAN_POINT ( 'NONE',  ( -11.00000000000000000, -79.69999999999998863, 0.000000000000000000 ) ) ;
#44092=CARTESIAN_POINT ( 'NONE',  ( 7.395758551695209349, -79.40217280339305717, 5.683424056470474994 ) ) ;
#44104=CARTESIAN_POINT ( 'NONE',  ( -4.952462208631658314, -77.86317697277696936, 9.641482076232696485 ) ) ;
#44105=CARTESIAN_POINT ( 'NONE',  ( -1.444794657067000054, -79.63356627858598813, -9.313366329545999633 ) ) ;
#44132=( NAMED_UNIT ( * ) SI_UNIT ( $, .STERADIAN. ) SOLID_ANGLE_UNIT ( ) );
#44135=AXIS2_PLACEMENT_3D ( 'NONE', #8213, #30183, #24335 ) ;
#44141=CARTESIAN_POINT ( 'NONE',  ( 9.554844271749594498, -78.06000170479207156, -5.239760174894856348 ) ) ;
#44167=CARTESIAN_POINT ( 'NONE',  ( 10.75000000000000000, -77.19999999999998863, -6.141891925717000695E-13 ) ) ;
#44174=CARTESIAN_POINT ( 'NONE',  ( 5.539808784079907511, -79.86666666666667425, -9.611650271896827746 ) ) ;
#44178=EDGE_LOOP ( 'NONE', ( #46189, #16975, #9723, #2930, #29788 ) ) ;
#44181=EDGE_CURVE ( 'NONE', #31248, #55607, #39944, .T. ) ;
#44184=CARTESIAN_POINT ( 'NONE',  ( -7.784718833714999064, -77.84296661922998339, 5.670217160303000270 ) ) ;
#44187=DIRECTION ( 'NONE',  ( -1.000000000000000000, 0.000000000000000000, 0.000000000000000000 ) ) ;
#44191=CARTESIAN_POINT ( 'NONE',  ( -8.035810179446766455, -79.05885488453131416, 4.621717112953465545 ) ) ;
#44195=CARTESIAN_POINT ( 'NONE',  ( 6.696351723200000272, -79.04823107411199601, -8.651398149159000184 ) ) ;
#44197=CARTESIAN_POINT ( 'NONE',  ( -1.864102395052000150, -79.98252921644699143, -11.06258289461000111 ) ) ;
#44199=ORIENTED_EDGE ( 'NONE', *, *, #49457, .F. ) ;
#44203=CARTESIAN_POINT ( 'NONE',  ( 9.767191983224998708, -80.00043356103655867, 0.05162932631433000269 ) ) ;
#44217=CARTESIAN_POINT ( 'NONE',  ( 0.000000000000000000, -76.39999999999999147, 0.000000000000000000 ) ) ;
#44228=DIRECTION ( 'NONE',  ( 1.000000000000000000, 0.000000000000000000, 0.000000000000000000 ) ) ;
#44230=DIRECTION ( 'NONE',  ( 0.000000000000000000, 1.000000000000000000, 0.000000000000000000 ) ) ;
#44231=CIRCLE ( 'NONE', #22582, 9.750000000000000000 ) ;
#44240=CARTESIAN_POINT ( 'NONE',  ( 1.121668155292469438, -80.00000000000000000, -9.414507127281368071 ) ) ;
#44241=CARTESIAN_POINT ( 'NONE',  ( 11.00000000000000000, -78.84999999999999432, 0.000000000000000000 ) ) ;
#44244=CARTESIAN_POINT ( 'NONE',  ( -9.133499927808999885, -79.16970150572998932, -3.177109475039999964 ) ) ;
#44249=AXIS2_PLACEMENT_3D ( 'NONE', #5441, #50042, #49460 ) ;
#44256=DIRECTION ( 'NONE',  ( 0.000000000000000000, -1.000000000000000000, 0.000000000000000000 ) ) ;
#44259=ADVANCED_FACE ( 'NONE', ( #13917 ), #8912, .F. ) ;
#44262=CARTESIAN_POINT ( 'NONE',  ( -8.396223008680999911, -79.81252310367197822, -4.990405176070999538 ) ) ;
#44276=CARTESIAN_POINT ( 'NONE',  ( 2.590478588064626386, -79.95266178902241450, 8.887573261231658250 ) ) ;
#44277=CARTESIAN_POINT ( 'NONE',  ( 8.423937229337077781, -80.14385089984534716, -7.240779987882011604 ) ) ;
#44279=CARTESIAN_POINT ( 'NONE',  ( 11.23392183412000023, -78.87684575912199136, 0.8531908288953000685 ) ) ;
#44286=VECTOR ( 'NONE', #55460, 1000.000000000000114 ) ;
#44290=CARTESIAN_POINT ( 'NONE',  ( 8.199999995296000321, -81.00000000470399186, 2.775962726994000217E-08 ) ) ;
#44291=CARTESIAN_POINT ( 'NONE',  ( -9.937637090044999510, -79.95706551386098226, 4.829168387547000840 ) ) ;
#44305=CARTESIAN_POINT ( 'NONE',  ( -8.517419447173999458, -77.10976152403689809, 3.788002893487000033 ) ) ;
#44309=ORIENTED_EDGE ( 'NONE', *, *, #23579, .T. ) ;
#44315=CARTESIAN_POINT ( 'NONE',  ( 6.083963560182000130, -78.60190654778497787, -9.135064530700001129 ) ) ;
#44316=CARTESIAN_POINT ( 'NONE',  ( 8.694733073939660883, -80.32630208333191035, 6.682997992873382920 ) ) ;
#44317=EDGE_CURVE ( 'NONE', #20614, #54465, #31028, .T. ) ;
#44320=CARTESIAN_POINT ( 'NONE',  ( 9.249483092228999226, -79.25084128437099196, 0.09778817195952001218 ) ) ;
#44325=CARTESIAN_POINT ( 'NONE',  ( -10.51276546006999979, -78.28204647501199531, 3.399949415165999689 ) ) ;
#44332=CARTESIAN_POINT ( 'NONE',  ( 4.054145691792253814, -79.54511357774050850, 10.29526509435834036 ) ) ;
#44338=ORIENTED_EDGE ( 'NONE', *, *, #32753, .F. ) ;
#44344=CARTESIAN_POINT ( 'NONE',  ( -9.249888792690324379, -78.10286309832869733, -0.3112582798825216379 ) ) ;
#44350=CARTESIAN_POINT ( 'NONE',  ( -1.170847499494476862, -77.48521246895937509, 9.179786802956089176 ) ) ;
#44351=CARTESIAN_POINT ( 'NONE',  ( 9.391860901740999523, -77.10358982349210066, 5.803232400709999794 ) ) ;
#44354=CARTESIAN_POINT ( 'NONE',  ( -3.536681740116999872, -78.29514014419099510, 9.036735673663999435 ) ) ;
#44358=CARTESIAN_POINT ( 'NONE',  ( -1.635010352784000087, -80.42239520082898707, -10.62493487727000030 ) ) ;
#44363=ORIENTED_EDGE ( 'NONE', *, *, #4584, .T. ) ;
#44370=CARTESIAN_POINT ( 'NONE',  ( -9.249777342727782070, -78.58959268168034384, 1.210717463251290482 ) ) ;
#44373=CARTESIAN_POINT ( 'NONE',  ( 5.550018459581000485, -80.45535737381698027, 9.959756219182001047 ) ) ;
#44383=CARTESIAN_POINT ( 'NONE',  ( 9.423985469995999509, -79.21901863870799332, 1.441710213756000059 ) ) ;
#44385=CARTESIAN_POINT ( 'NONE',  ( 3.321932689531000182, -77.19999999999998863, 10.22385755016999909 ) ) ;
#44396=CARTESIAN_POINT ( 'NONE',  ( 7.559982449049000408, -77.08685820500399188, -6.032732969207000195 ) ) ;
#44400=ADVANCED_FACE ( 'NONE', ( #17699 ), #43982, .T. ) ;
#44431=CARTESIAN_POINT ( 'NONE',  ( 1.260641617779999946, -77.57417861372799450, 9.621927669549000584 ) ) ;
#44433=FACE_BOUND ( 'NONE', #51715, .T. ) ;
#44438=CARTESIAN_POINT ( 'NONE',  ( -8.731575513440832381, -78.62679321767426188, -3.053146778519897797 ) ) ;
#44444=DIRECTION ( 'NONE',  ( 0.000000000000000000, -1.000000000000000000, 0.000000000000000000 ) ) ;
#44448=ORIENTED_EDGE ( 'NONE', *, *, #46354, .F. ) ;
#44449=CARTESIAN_POINT ( 'NONE',  ( 9.249483092228999226, -78.85084128437098627, 0.09778817195952001218 ) ) ;
#44450=CARTESIAN_POINT ( 'NONE',  ( 2.879226727952094222, -79.34583333333331723, -10.71369944335146940 ) ) ;
#44458=ORIENTED_EDGE ( 'NONE', *, *, #30472, .T. ) ;
#44463=CARTESIAN_POINT ( 'NONE',  ( -7.921993249237998747, -78.50374277172099369, -5.283218639336999978 ) ) ;
#44470=CARTESIAN_POINT ( 'NONE',  ( -8.604107503949739666, -79.06923224600832611, 3.550580747324208364 ) ) ;
#44474=ORIENTED_EDGE ( 'NONE', *, *, #41654, .T. ) ;
#44475=CARTESIAN_POINT ( 'NONE',  ( -10.40934573790000073, -78.34592221579498528, 3.366502286031999969 ) ) ;
#44477=CARTESIAN_POINT ( 'NONE',  ( -9.616088855336998975, -79.70165346197198630, 5.532765289540999554 ) ) ;
#44488=EDGE_CURVE ( 'NONE', #37542, #27414, #45754, .T. ) ;
#44490=CIRCLE ( 'NONE', #33192, 10.50000000000000000 ) ;
#44492=CARTESIAN_POINT ( 'NONE',  ( 0.000000000000000000, -80.99999999999998579, 7.000000000000000000 ) ) ;
#44506=CARTESIAN_POINT ( 'NONE',  ( -8.796335266380006956, -78.04791666666666572, 6.760013919724027431 ) ) ;
#44520=DIRECTION ( 'NONE',  ( -0.7071067811865474617, -0.7071067811865474617, 1.305612310955086883E-09 ) ) ;
#44532=CARTESIAN_POINT ( 'NONE',  ( 8.963249880471998665, -78.87092023966599186, -2.560381131858999737 ) ) ;
#44537=CARTESIAN_POINT ( 'NONE',  ( 0.000000000000000000, -77.01875000000549676, 0.000000000000000000 ) ) ;
#44545=CARTESIAN_POINT ( 'NONE',  ( -10.78523893070000028, -77.41014297881199013, 2.631402515253999930 ) ) ;
#44554=CARTESIAN_POINT ( 'NONE',  ( -5.809791519574999619, -79.19554259676998242, 7.851562197947999699 ) ) ;
#44569=CARTESIAN_POINT ( 'NONE',  ( -0.7613100899427974744, -79.98164650648521956, 9.218583111519835782 ) ) ;
#44572=CARTESIAN_POINT ( 'NONE',  ( 0.9331110433225999756, -78.98921517645298707, 11.22756599386000076 ) ) ;
#44573=CARTESIAN_POINT ( 'NONE',  ( 2.900604236686527670, -77.25055390848557124, -8.783348422349369855 ) ) ;
#44582=CARTESIAN_POINT ( 'NONE',  ( -0.5280093414736000135, -79.17817062466399136, -11.14507989169999824 ) ) ;
#44596=CONICAL_SURFACE ( 'NONE', #41784, 1.099999997148999986, 0.7853981633972997312 ) ;
#44600=CARTESIAN_POINT ( 'NONE',  ( -4.778484498315999751, -78.62325255039799288, 8.361775879827998637 ) ) ;
#44605=ORIENTED_EDGE ( 'NONE', *, *, #30923, .T. ) ;
#44612=CARTESIAN_POINT ( 'NONE',  ( -9.505686244346000180, -79.38849246909899193, 5.486888517706000279 ) ) ;
#44613=CARTESIAN_POINT ( 'NONE',  ( -10.48321433724633245, -80.43697916666563685, 2.816410591909088268 ) ) ;
#44616=CARTESIAN_POINT ( 'NONE',  ( 9.332634751654579119, -79.20070731308940992, 0.09866879888904338258 ) ) ;
#44620=CARTESIAN_POINT ( 'NONE',  ( -10.99999999999999822, -77.61041666666666572, -1.439896632895323325 ) ) ;
#44623=CARTESIAN_POINT ( 'NONE',  ( -7.632977269198000236, -78.80811017521499195, -8.138136006783000198 ) ) ;
#44627=B_SPLINE_SURFACE_WITH_KNOTS ( 'NONE', 3, 3, ( 
 ( #32900, #28180, #41195, #54201, #27604, #13737, #40618, #18190, #49780, #45938, #5758, #1072, #499, #18477, #36468, #50073, #5186, #23190, #784, #50360, #14613, #18764, #23474, #41485, #27891, #19059, #36757, #23765, #32607, #10201, #54776, #14317, #37047, #15790, #33493 ),
 ( #37924, #52392, #51531, #25220, #11087, #28771, #47397, #34355, #55949, #15201, #6051, #33778, #20793, #19636, #42373, #46820, #2797, #38797, #6345, #43240, #46527, #56816, #34065, #29637, #1942, #51818, #42077, #29066, #16373, #7219, #24059, #24933, #19936, #55652, #15499 ),
 ( #42955, #11373, #1647, #11946, #16084, #6640, #29351, #37634, #52102, #24649, #33191, #6929, #11661, #47109, #51238, #42659, #2226, #2509, #10790, #20227, #24360, #38219, #56241, #20513, #38510, #56525, #47690, #39089, #25509, #17821, #25797, #26648, #44383, #48537, #17518 ),
 ( #43824, #57096, #39383, #35807, #8083, #7796, #26080, #58260, #44685, #13077, #53838, #21937, #8662, #34928, #48262, #57964, #35508, #57388, #12225, #29923, #44105, #53537, #3654, #49113, #4237, #22235, #7510, #21367, #3936, #34644, #30215, #35213, #43527, #3372, #3087 ) ),
 .UNSPECIFIED., .F., .F., .F.,
 ( 4, 4 ),
 ( 4, 1, 1, 1, 1, 1, 1, 1, 1, 1, 1, 1, 1, 1, 1, 1, 1, 1, 1, 1, 1, 1, 1, 1, 1, 1, 1, 1, 1, 1, 1, 1, 4 ),
 ( -0.1387574078320000237, 1.138757407831999968 ),
 ( 0.4756668553019000045, 0.4923735486379000048, 0.5090802419739000051, 0.5257869353097999188, 0.5424936286457999746, 0.5592003219817999193, 0.5759070153176999440, 0.5926137086536999998, 0.6093204019896999446, 0.6260270953255999693, 0.6427337886616000251, 0.6594404819975999699, 0.6761471753334999946, 0.6928538686695000504, 0.7095605620054999951, 0.7262672553414000198, 0.7429739486774000756, 0.7596806420133999094, 0.7763873353493999652, 0.7930940286852999899, 0.8098007220212999346, 0.8265074153572999904, 0.8432141086932000151, 0.8599208020291999599, 0.8766274953652000157, 0.8933341887010999294, 0.9100408820370999852, 0.9267475753731000410, 0.9434542687089999546, 0.9601609620450000104, 0.9768676553809999552, 0.9935743487168999799, 1.010281042052999956 ),
 .UNSPECIFIED. ) ;
#44636=EDGE_LOOP ( 'NONE', ( #21534, #35765, #35585, #7963 ) ) ;
#44639=CARTESIAN_POINT ( 'NONE',  ( -0.4256071464968388396, -79.62857731458335309, 9.520305438052526270 ) ) ;
#44645=CARTESIAN_POINT ( 'NONE',  ( -5.372582819375519847, -78.17569175854035279, -7.531333529607578292 ) ) ;
#44649=ORIENTED_EDGE ( 'NONE', *, *, #23773, .T. ) ;
#44650=CARTESIAN_POINT ( 'NONE',  ( -1.624220529728441997, -77.48908808038281393, 9.106525592228415178 ) ) ;
#44651=CARTESIAN_POINT ( 'NONE',  ( -10.84202097104999929, -77.35475100115499458, 2.082001701158999740 ) ) ;
#44653=EDGE_CURVE ( 'NONE', #18080, #6792, #47570, .T. ) ;
#44655=CARTESIAN_POINT ( 'NONE',  ( -9.157500079073999544, -78.86361672676999035, 3.211059275314999795 ) ) ;
#44679=DIRECTION ( 'NONE',  ( -1.000000000000000000, 0.000000000000000000, 0.000000000000000000 ) ) ;
#44685=CARTESIAN_POINT ( 'NONE',  ( -8.446673021817000304, -79.98423817768198774, 4.180901655042999820 ) ) ;
#44687=CARTESIAN_POINT ( 'NONE',  ( 7.164578282910722962, -77.28124999999998579, -8.391376934739398052 ) ) ;
#44715=VERTEX_POINT ( 'NONE', #5551 ) ;
#44724=CARTESIAN_POINT ( 'NONE',  ( 10.94195044575999987, -77.58938080696006523, -1.468969119710000104 ) ) ;
#44732=CARTESIAN_POINT ( 'NONE',  ( 9.703485699160999900, -77.46048329721199366, 0.1143444355825999903 ) ) ;
#44739=CARTESIAN_POINT ( 'NONE',  ( -1.989514602459929504, -76.94999999999998863, -9.342458649981287166 ) ) ;
#44750=CARTESIAN_POINT ( 'NONE',  ( -10.71369944335148183, -79.17916666666667425, 2.879226727952048481 ) ) ;
#44761=CARTESIAN_POINT ( 'NONE',  ( 4.490468926300999364, -77.02113108638108940, 10.16576052825000076 ) ) ;
#44765=CARTESIAN_POINT ( 'NONE',  ( 1.236990682704000033, -77.82157087262599759, 9.441410396910001168 ) ) ;
#44791=VECTOR ( 'NONE', #16293, 1000.000000000000000 ) ;
#44798=CARTESIAN_POINT ( 'NONE',  ( -2.858407197967999913, -79.99999999999998579, 8.797272775729998884 ) ) ;
#44802=CARTESIAN_POINT ( 'NONE',  ( 7.396646590749633710, -77.79807357050631822, -5.684287846210173356 ) ) ;
#44804=ADVANCED_FACE ( 'NONE', ( #7592 ), #53187, .F. ) ;
#44821=DIRECTION ( 'NONE',  ( 0.000000000000000000, 1.000000000000000000, 2.031724556816999953E-13 ) ) ;
#44824=ORIENTED_EDGE ( 'NONE', *, *, #27994, .T. ) ;
#44840=DIRECTION ( 'NONE',  ( 0.000000000000000000, -1.000000000000000000, 0.000000000000000000 ) ) ;
#44844=EDGE_CURVE ( 'NONE', #57837, #1524, #3736, .T. ) ;
#44846=CARTESIAN_POINT ( 'NONE',  ( -6.031270819540000439, -77.00661118349269429, -8.856729339061999440 ) ) ;
#44854=CARTESIAN_POINT ( 'NONE',  ( -2.116314338179000387, -79.87746842018698601, -9.535298106756000536 ) ) ;
#44860=VERTEX_POINT ( 'NONE', #2599 ) ;
#44869=CONICAL_SURFACE ( 'NONE', #39205, 2.699999999213000379, 0.7853981633972997312 ) ;
#44870=CARTESIAN_POINT ( 'NONE',  ( 5.368767637727030362, -79.92621298444481681, 7.532222042164998577 ) ) ;
#44902=CARTESIAN_POINT ( 'NONE',  ( 9.250000000000000000, -78.74999999999998579, 0.000000000000000000 ) ) ;
#44905=CARTESIAN_POINT ( 'NONE',  ( -3.673218652927999539, -79.33230776043399146, 10.34270183798999909 ) ) ;
#44906=CARTESIAN_POINT ( 'NONE',  ( 9.611650271896824194, -79.30833333333332291, -5.539808784079918169 ) ) ;
#44912=CARTESIAN_POINT ( 'NONE',  ( 8.824074283052752321, -77.22496508380866942, -2.868679438668469750 ) ) ;
#44913=CARTESIAN_POINT ( 'NONE',  ( 11.00000000000000000, -77.84999999999999432, 0.000000000000000000 ) ) ;
#44916=CARTESIAN_POINT ( 'NONE',  ( -10.74684349920000059, -79.72579375008199065, 2.363312785431999963 ) ) ;
#44927=ORIENTED_EDGE ( 'NONE', *, *, #32322, .F. ) ;
#44930=CARTESIAN_POINT ( 'NONE',  ( 0.000000000000000000, -74.64999999999999147, 0.000000000000000000 ) ) ;
#44933=CARTESIAN_POINT ( 'NONE',  ( -1.185608318420265928, -79.63492132814884883, 9.455258074239862864 ) ) ;
#44941=CARTESIAN_POINT ( 'NONE',  ( -3.659791739852715331, -78.19279094063269042, -8.496079794231707893 ) ) ;
#44945=VERTEX_POINT ( 'NONE', #19077 ) ;
#44946=CARTESIAN_POINT ( 'NONE',  ( 1.369538937357239083, -77.46319207057830170, 9.148125136416654257 ) ) ;
#44947=CARTESIAN_POINT ( 'NONE',  ( 10.77519778174000109, -77.23148241939499314, -1.228540277667999892 ) ) ;
#44949=CARTESIAN_POINT ( 'NONE',  ( -9.669247687117000112, -77.89720653638498504, -0.8224101967608999919 ) ) ;
#44957=CARTESIAN_POINT ( 'NONE',  ( 9.250000000000000000, -78.74999999999998579, 0.000000000000000000 ) ) ;
#44997=DIRECTION ( 'NONE',  ( -1.000000000000000000, 0.000000000000000000, 0.000000000000000000 ) ) ;
#45001=DIRECTION ( 'NONE',  ( 0.000000000000000000, -1.000000000000000000, 0.000000000000000000 ) ) ;
#45006=DIRECTION ( 'NONE',  ( 1.000000000000000000, 0.000000000000000000, 0.000000000000000000 ) ) ;
#45008=SURFACE_STYLE_USAGE ( .BOTH. , #39690 ) ;
#45010=VERTEX_POINT ( 'NONE', #32914 ) ;
#45029=CARTESIAN_POINT ( 'NONE',  ( -9.022250383429000209, -78.73955560801599063, -3.573472734901999903 ) ) ;
#45054=CARTESIAN_POINT ( 'NONE',  ( -11.00000000000000888, -79.18958333333333144, 1.439896632895279360 ) ) ;
#45066=CARTESIAN_POINT ( 'NONE',  ( 8.286539809994000194, -78.24792830956099010, 4.690803151849999963 ) ) ;
#45078=CARTESIAN_POINT ( 'NONE',  ( 9.663556473158999793, -79.58198580643298214, -5.128693071642000056 ) ) ;
#45083=VERTEX_POINT ( 'NONE', #34946 ) ;
#45087=CARTESIAN_POINT ( 'NONE',  ( -9.699833017908000343, -79.74065229497952600, 1.146274062705999963 ) ) ;
#45095=AXIS2_PLACEMENT_3D ( 'NONE', #16309, #52324, #47332 ) ;
#45101=CARTESIAN_POINT ( 'NONE',  ( -0.4252449232878383056, -78.72143397250610519, -9.249944552399744779 ) ) ;
#45105=CARTESIAN_POINT ( 'NONE',  ( 8.777412155057099596, -77.82412362302341080, -2.980421710618992304 ) ) ;
#45114=PLANE ( 'NONE',  #10000 ) ;
#45117=CARTESIAN_POINT ( 'NONE',  ( 9.191325695085856395, -79.84005264655188228, -1.210935613487206908 ) ) ;
#45126=CARTESIAN_POINT ( 'NONE',  ( -7.412025882568599400, -78.16672174443260701, -8.233944902729591675 ) ) ;
#45129=CARTESIAN_POINT ( 'NONE',  ( 11.00000000000000000, -77.44999999999998863, 0.000000000000000000 ) ) ;
#45137=CARTESIAN_POINT ( 'NONE',  ( -4.832441116568999995, -78.74550106883198453, 8.456193503077001239 ) ) ;
#45139=CARTESIAN_POINT ( 'NONE',  ( -6.862215669877000046, -79.33480064555399736, -7.123593673834999862 ) ) ;
#45145=VECTOR ( 'NONE', #29126, 1000.000000000000114 ) ;
#45150=ORIENTED_EDGE ( 'NONE', *, *, #38046, .F. ) ;
#45151=CARTESIAN_POINT ( 'NONE',  ( 10.02418919408999898, -78.14383715211899073, -4.770675716736000105 ) ) ;
#45159=CARTESIAN_POINT ( 'NONE',  ( -4.373213035511999358, -79.35790588805998880, -8.733596771889999388 ) ) ;
#45170=CARTESIAN_POINT ( 'NONE',  ( -2.572125540837000290, -78.35365303490424083, -9.357076443458000270 ) ) ;
#45171=CARTESIAN_POINT ( 'NONE',  ( 7.030819185249340464, -79.90638907312039407, 6.010730751432092234 ) ) ;
#45179=CARTESIAN_POINT ( 'NONE',  ( -11.00000000000000000, -79.09999999999999432, 0.000000000000000000 ) ) ;
#45193=CARTESIAN_POINT ( 'NONE',  ( 7.247098260574433404, -76.95000000000000284, -6.187590336956020565 ) ) ;
#45197=CARTESIAN_POINT ( 'NONE',  ( 8.488869829350999652, -78.99276232907497786, 4.102512142575000631 ) ) ;
#45204=CARTESIAN_POINT ( 'NONE',  ( 0.9090372547675998893, -78.79855302811299111, 10.93790052299999971 ) ) ;
#45213=CARTESIAN_POINT ( 'NONE',  ( -1.439896632895311335, -77.71458333333332291, -11.00000000000000178 ) ) ;
#45217=CARTESIAN_POINT ( 'NONE',  ( 8.374122929021998729, -78.11349234901598493, 7.207772231549999908 ) ) ;
#45222=CARTESIAN_POINT ( 'NONE',  ( -8.082524092276901939, -79.95833333333331439, 4.658475568430788805 ) ) ;
#45233=ORIENTED_EDGE ( 'NONE', *, *, #53910, .T. ) ;
#45238=CARTESIAN_POINT ( 'NONE',  ( -4.968906709420642720, -78.17991984054995669, -7.802392233778754793 ) ) ;
#45245=CARTESIAN_POINT ( 'NONE',  ( 1.445297155599249983, -77.46252827442208400, 9.136381658210661172 ) ) ;
#45246=CARTESIAN_POINT ( 'NONE',  ( -9.177034484502000211, -77.38324421815998733, 6.137278520473000043 ) ) ;
#45248=CARTESIAN_POINT ( 'NONE',  ( -9.346518596363001308, -77.86878270725598838, 2.610229778083999808 ) ) ;
#45252=CARTESIAN_POINT ( 'NONE',  ( -8.744140569415000286, -80.43625931648698213, 7.086030162020000134 ) ) ;
#45253=CARTESIAN_POINT ( 'NONE',  ( -10.87240354821999944, -78.93804972576597834, -1.216000584195999767 ) ) ;
#45258=AXIS2_PLACEMENT_3D ( 'NONE', #40067, #53661, #17347 ) ;
#45269=CARTESIAN_POINT ( 'NONE',  ( -4.206058715153999650, -80.52587970449398824, 10.59755966650999959 ) ) ;
#45279=CARTESIAN_POINT ( 'NONE',  ( 8.796335266379992746, -79.89791666666666003, -6.760013919724047859 ) ) ;
#45282=DIRECTION ( 'NONE',  ( -1.000000000000000000, 0.000000000000000000, 0.000000000000000000 ) ) ;
#45287=EDGE_CURVE ( 'NONE', #21041, #24542, #42882, .T. ) ;
#45294=CARTESIAN_POINT ( 'NONE',  ( 9.250000000000005329, -78.26041666666667140, 1.210822168571039192 ) ) ;
#45301=CARTESIAN_POINT ( 'NONE',  ( 0.000000000000000000, -76.29999999995945359, 0.000000000000000000 ) ) ;
#45307=AXIS2_PLACEMENT_3D ( 'NONE', #17182, #43779, #4490 ) ;
#45313=CARTESIAN_POINT ( 'NONE',  ( 1.791008777272000030, -80.21228312261607130, 11.11143388882000060 ) ) ;
#45319=VERTEX_POINT ( 'NONE', #158 ) ;
#45325=CARTESIAN_POINT ( 'NONE',  ( 7.890274420948999001, -78.91009858278999900, -5.649267206312000411 ) ) ;
#45346=CARTESIAN_POINT ( 'NONE',  ( -2.879226727952071574, -79.30416666666667425, -10.71369944335147473 ) ) ;
#45357=DIRECTION ( 'NONE',  ( -1.000000000000000000, 0.000000000000000000, 0.000000000000000000 ) ) ;
#45361=CARTESIAN_POINT ( 'NONE',  ( -8.606866362194999454, -77.99211384739999176, -4.073355822332000109 ) ) ;
#45373=EDGE_CURVE ( 'NONE', #12448, #10446, #39109, .T. ) ;
#45384=B_SPLINE_CURVE_WITH_KNOTS ( 'NONE', 3,
 ( #6391, #51285, #7267, #33539, #2557, #29111, #56571, #16130, #43000, #24977, #51863, #10839, #6975, #25268, #55402, #46864, #51576, #14949, #56286 ),
 .UNSPECIFIED., .F., .F.,
 ( 4, 1, 1, 1, 1, 1, 1, 1, 1, 1, 1, 1, 1, 1, 1, 1, 4 ),
 ( 0.000000000000000000, 0.01250073040970592873, 0.04500068264926284506, 0.07750063488862506123, 0.1100005871281820868, 0.1425005393677388765, 0.1750004916071013217, 0.2075004438466583334, 0.2400003960862151509, 0.2725003483255775683, 0.3050003005651346077, 0.3375002528046914252, 0.3700002050440538426, 0.4025001572836108821, 0.4350001095231676440, 0.4675000617625301169, 0.5000000000000000000 ),
 .UNSPECIFIED. ) ;
#45399=CARTESIAN_POINT ( 'NONE',  ( -0.7887765935117789784, -78.71827052605868857, -9.221363235537282321 ) ) ;
#45407=AXIS2_PLACEMENT_3D ( 'NONE', #37578, #46467, #33139 ) ;
#45432=DIRECTION ( 'NONE',  ( -0.3090169943750105119, 0.000000000000000000, -0.9510565162951329921 ) ) ;
#45440=EDGE_CURVE ( 'NONE', #27909, #12885, #32477, .T. ) ;
#45445=CARTESIAN_POINT ( 'NONE',  ( 0.5770588204160999046, -77.36396459359899325, 11.19704361211000077 ) ) ;
#45447=ORIENTED_EDGE ( 'NONE', *, *, #43097, .T. ) ;
#45448=AXIS2_PLACEMENT_3D ( 'NONE', #14343, #53632, #32340 ) ;
#45452=CARTESIAN_POINT ( 'NONE',  ( 1.739862777674999972, -79.25120313159598595, 9.611119481339999382 ) ) ;
#45453=EDGE_CURVE ( 'NONE', #20866, #16241, #35527, .T. ) ;
#45458=EDGE_LOOP ( 'NONE', ( #36889, #2404, #15169, #42211 ) ) ;
#45464=CARTESIAN_POINT ( 'NONE',  ( 9.051070938631999852, -77.52936199016376406, 3.499832029064999794 ) ) ;
#45465=CARTESIAN_POINT ( 'NONE',  ( 8.236271263160999112, -79.88807656218412490, 4.209621724653113795 ) ) ;
#45472=DIRECTION ( 'NONE',  ( 0.000000000000000000, 1.000000000000000000, 0.000000000000000000 ) ) ;
#45486=CARTESIAN_POINT ( 'NONE',  ( -5.088691759813757095E-08, -76.94999999999998863, -9.499908983443795307 ) ) ;
#45490=CARTESIAN_POINT ( 'NONE',  ( 4.155310858692000231, -78.36743808823698032, -8.688302574878001394 ) ) ;
#45495=FACE_OUTER_BOUND ( 'NONE', #13352, .T. ) ;
#45499=CARTESIAN_POINT ( 'NONE',  ( 0.9090372547675998893, -78.85885595378398705, 10.93790052299999971 ) ) ;
#45511=ADVANCED_FACE ( 'NONE', ( #46770 ), #28718, .F. ) ;
#45513=CARTESIAN_POINT ( 'NONE',  ( -9.152236916771000708, -78.75961649866798098, 6.189866966782000546 ) ) ;
#45519=CARTESIAN_POINT ( 'NONE',  ( 0.5437984056370215313, -79.57105364439701134, 11.05137384886683094 ) ) ;
#45540=CARTESIAN_POINT ( 'NONE',  ( -1.534489406528057431, -77.48831705290680816, 9.121860746232874462 ) ) ;
#45541=CARTESIAN_POINT ( 'NONE',  ( 3.792698199283999649, -78.02275488312699281, -10.36819406884000117 ) ) ;
#45543=CARTESIAN_POINT ( 'NONE',  ( -4.814859605045999302, -78.80676906851299179, 8.425427962446999430 ) ) ;
#45549=CARTESIAN_POINT ( 'NONE',  ( 8.185910223524000884, -78.12337145011899509, -6.914387615432000977 ) ) ;
#45553=ORIENTED_EDGE ( 'NONE', *, *, #50627, .F. ) ;
#45564=CARTESIAN_POINT ( 'NONE',  ( -1.146763852601999867, -78.69446787273398058, -9.343239705575001608 ) ) ;
#45570=CARTESIAN_POINT ( 'NONE',  ( 0.000000000000000000, -74.64999999999999147, 0.000000000000000000 ) ) ;
#45574=CARTESIAN_POINT ( 'NONE',  ( 11.00000000000000711, -79.93958333333333144, -1.439896632895300010 ) ) ;
#45578=CARTESIAN_POINT ( 'NONE',  ( 11.00000000000000000, -79.94999999999998863, 0.000000000000000000 ) ) ;
#45592=CARTESIAN_POINT ( 'NONE',  ( -8.058638732054999920, -78.40938521931758487, -7.451332657186999775 ) ) ;
#45595=EDGE_LOOP ( 'NONE', ( #1316, #38826, #35774, #1383 ) ) ;
#45621=CARTESIAN_POINT ( 'NONE',  ( 4.186942200393000135, -78.37004582933998620, -8.754440266352000677 ) ) ;
#45650=CARTESIAN_POINT ( 'NONE',  ( 0.000000000000000000, -76.19999999999998863, -9.749999999999667821 ) ) ;
#45653=CARTESIAN_POINT ( 'NONE',  ( 10.26236580194999881, -77.96083789290199206, -4.398705269624000103 ) ) ;
#45656=CARTESIAN_POINT ( 'NONE',  ( -8.431119552239000114, -78.41847128433398950, 4.425675013809000191 ) ) ;
#45661=ORIENTED_EDGE ( 'NONE', *, *, #11379, .F. ) ;
#45667=VERTEX_POINT ( 'NONE', #49354 ) ;
#45668=CARTESIAN_POINT ( 'NONE',  ( -9.839875214663999614, -79.83481699542699062, 4.781661263485999847 ) ) ;
#45670=CYLINDRICAL_SURFACE ( 'NONE', #56735, 1.000000000000000000 ) ;
#45683=CARTESIAN_POINT ( 'NONE',  ( -4.657705497668140460, -79.18357720769643038, -8.081617589960574222 ) ) ;
#45684=CARTESIAN_POINT ( 'NONE',  ( 1.487051409078008701, -77.48714799342995718, -9.589708388838586117 ) ) ;
#45689=DIRECTION ( 'NONE',  ( -1.000000000000000000, 0.000000000000000000, 0.000000000000000000 ) ) ;
#45694=CARTESIAN_POINT ( 'NONE',  ( 3.884926167828604449, -78.75961067256588422, -8.428911604562424387 ) ) ;
#45697=CARTESIAN_POINT ( 'NONE',  ( -9.158362268698009956, -80.14686259273240410, -6.092845169229706315 ) ) ;
#45700=CARTESIAN_POINT ( 'NONE',  ( 0.000000000000000000, -80.35000000001998899, -10.84999999997999964 ) ) ;
#45705=CARTESIAN_POINT ( 'NONE',  ( 0.000000000000000000, -78.69999999999998863, -2.799999999999969180 ) ) ;
#45706=CARTESIAN_POINT ( 'NONE',  ( 7.000000000000000000, -80.99999999999998579, 0.000000000000000000 ) ) ;
#45716=CARTESIAN_POINT ( 'NONE',  ( 5.329123786712647970, -79.52101871112249398, -8.124383524005093449 ) ) ;
#45719=CARTESIAN_POINT ( 'NONE',  ( -1.199999995295999877, -81.00000000470399186, -7.000000027760000521 ) ) ;
#45727=CARTESIAN_POINT ( 'NONE',  ( -9.250000000000000000, -79.99999999999998579, 2.662757480928999879E-14 ) ) ;
#45739=CARTESIAN_POINT ( 'NONE',  ( 0.000000000000000000, -76.39999999999999147, -9.549999999999997158 ) ) ;
#45742=CARTESIAN_POINT ( 'NONE',  ( -2.843296433296999659, -78.09765876690597963, -10.84539213913000033 ) ) ;
#45751=CARTESIAN_POINT ( 'NONE',  ( 8.944729675425000082, -79.79320053239750621, 3.923329690209000908 ) ) ;
#45754=LINE ( 'NONE', #33007, #36241 ) ;
#45761=LINE ( 'NONE', #37166, #17430 ) ;
#45762=CARTESIAN_POINT ( 'NONE',  ( 8.993105270996114342, -79.86890122386594726, 2.164559197160741633 ) ) ;
#45765=CARTESIAN_POINT ( 'NONE',  ( 9.208615812369000508, -77.02473186629366353, 2.957800710608999850 ) ) ;
#45783=CARTESIAN_POINT ( 'NONE',  ( 7.685661446562000343, -76.94999999999998863, -5.583959896778000420 ) ) ;
#45788=CARTESIAN_POINT ( 'NONE',  ( -9.554254755627999529, -78.19689511346298616, 1.212198840764999952 ) ) ;
#45796=CARTESIAN_POINT ( 'NONE',  ( 10.55657102546000026, -78.71839418212100270, -3.003801718854000047 ) ) ;
#45809=CARTESIAN_POINT ( 'NONE',  ( -6.966543547089000477, -79.37764829398598465, -8.575847751312000611 ) ) ;
#45814=CARTESIAN_POINT ( 'NONE',  ( -9.439017928876026531, -79.49271986116634992, -5.601139116439918908 ) ) ;
#45832=ORIENTED_EDGE ( 'NONE', *, *, #4076, .F. ) ;
#45835=CARTESIAN_POINT ( 'NONE',  ( 7.482391911512093152, -77.40012167121783193, 5.438283650742095965 ) ) ;
#45836=CARTESIAN_POINT ( 'NONE',  ( -10.84202097104999929, -77.41505392682599052, 2.082001701158999740 ) ) ;
#45843=CARTESIAN_POINT ( 'NONE',  ( -3.493617039247999934, -80.58938358939499835, -10.33892454317000187 ) ) ;
#45844=CARTESIAN_POINT ( 'NONE',  ( -3.536853559812999759, -79.52798916675298813, -10.35270415072999839 ) ) ;
#45859=CARTESIAN_POINT ( 'NONE',  ( 1.222863591967999985, -77.44381939105899448, 9.333584474513999751 ) ) ;
#45869=CARTESIAN_POINT ( 'NONE',  ( 10.85730540529999999, -79.07124013742898683, 1.607151491820999922 ) ) ;
#45879=FACE_OUTER_BOUND ( 'NONE', #14870, .T. ) ;
#45889=CARTESIAN_POINT ( 'NONE',  ( 0.000000000000000000, 0.000000000000000000, 0.000000000000000000 ) ) ;
#45891=LINE ( 'NONE', #55310, #19562 ) ;
#45896=ORIENTED_EDGE ( 'NONE', *, *, #4707, .F. ) ;
#45899=CARTESIAN_POINT ( 'NONE',  ( -7.407754918741036754, -80.41680592794931215, -8.285828061842591907 ) ) ;
#45903=CARTESIAN_POINT ( 'NONE',  ( 5.896854890547934325, -78.28013406490441639, -7.126572464670269724 ) ) ;
#45912=CARTESIAN_POINT ( 'NONE',  ( -3.907230163516999699, -77.86187217243097791, -8.882807090995999744 ) ) ;
#45938=CARTESIAN_POINT ( 'NONE',  ( -6.603669512656000329, -79.76338829707400180, 7.175056597861000363 ) ) ;
#45944=CARTESIAN_POINT ( 'NONE',  ( -0.9873574601251999816, -77.29720827014600104, -11.23080870426000111 ) ) ;
#45945=B_SPLINE_CURVE_WITH_KNOTS ( 'NONE', 3,
 ( #40070, #52586, #22363, #13503, #23825, #1706, #1418, #27663, #560, #10856, #55124, #33258, #46293, #55718, #50718, #54836, #18827, #36529, #5819, #32092, #5244, #6113, #14093, #54553, #1129 ),
 .UNSPECIFIED., .F., .F.,
 ( 4, 2, 2, 2, 2, 2, 2, 2, 1, 2, 2, 2, 4 ),
 ( 0.000000000000000000, 0.1249999840576382637, 0.1874999760864574372, 0.2499999681152765829, 0.3749999521729150409, 0.4374999442017342699, 0.4999999362305534989, 0.5312499322449630856, 0.5624999282593725614, 0.6249999202881917348, 0.7499999043458301928, 0.8749998884034685398, 0.9999998724611069978 ),
 .UNSPECIFIED. ) ;
#45948=CARTESIAN_POINT ( 'NONE',  ( 6.053520011479999852, -78.34022787947299094, 7.208750930507999755 ) ) ;
#45965=ORIENTED_EDGE ( 'NONE', *, *, #25068, .F. ) ;
#45980=CARTESIAN_POINT ( 'NONE',  ( 5.928084975461002770, -78.02720074687999841, -7.683204820502274046 ) ) ;
#45987=CARTESIAN_POINT ( 'NONE',  ( 7.179580682979864292, -78.79576402591504802, -5.832456873467035230 ) ) ;
#45991=CARTESIAN_POINT ( 'NONE',  ( -9.698041772758232426, -80.13957045507287091, -5.198397055125564492 ) ) ;
#46008=EDGE_CURVE ( 'NONE', #57837, #57298, #52318, .T. ) ;
#46010=CARTESIAN_POINT ( 'NONE',  ( -10.21587511493324207, -77.42472830502559589, 3.417954814639385663 ) ) ;
#46016=SHAPE_REPRESENTATION ( 'Push Button Connector', ( #43526 ), #9600 ) ;
#46020=CARTESIAN_POINT ( 'NONE',  ( 8.335168759715775977, -78.31433322054517987, -4.010873337216996681 ) ) ;
#46024=CARTESIAN_POINT ( 'NONE',  ( 7.830665294675000609, -79.09361510090498371, -5.606588350762000239 ) ) ;
#46026=CARTESIAN_POINT ( 'NONE',  ( -9.342118770336998779, -79.29745298729598346, -3.249678031071000284 ) ) ;
#46035=FACE_OUTER_BOUND ( 'NONE', #26757, .T. ) ;
#46038=CARTESIAN_POINT ( 'NONE',  ( -1.320560947307999999, -77.81367477412999278, 11.02278443658000029 ) ) ;
#46043=CARTESIAN_POINT ( 'NONE',  ( -9.687172913667000174, -79.90065629675500247, -1.248753675804000096 ) ) ;
#46067=CARTESIAN_POINT ( 'NONE',  ( 11.26616169758000119, -78.37118338113400284, 0.05236123134324000700 ) ) ;
#46074=CARTESIAN_POINT ( 'NONE',  ( -9.483626256930000054, -77.39407522740199852, -0.1248487836051000166 ) ) ;
#46079=CARTESIAN_POINT ( 'NONE',  ( -8.012466620630000591, -78.25374277172099369, -5.343555802860000981 ) ) ;
#46085=DIRECTION ( 'NONE',  ( 0.000000000000000000, 1.000000000000000000, 0.000000000000000000 ) ) ;
#46088=CARTESIAN_POINT ( 'NONE',  ( -7.022507694776999543, -79.42070304043799922, 8.434951230355999030 ) ) ;
#46089=DIRECTION ( 'NONE',  ( 0.000000000000000000, -1.000000000000000000, 0.000000000000000000 ) ) ;
#46108=CARTESIAN_POINT ( 'NONE',  ( 7.318212639625410354, -79.63318163283004480, -8.179950038113810606 ) ) ;
#46109=EDGE_CURVE ( 'NONE', #26404, #1613, #53901, .T. ) ;
#46115=VERTEX_POINT ( 'NONE', #27306 ) ;
#46127=ORIENTED_EDGE ( 'NONE', *, *, #58377, .F. ) ;
#46130=CARTESIAN_POINT ( 'NONE',  ( 7.481666628245163153, -77.40013210855786951, 5.439281462751108798 ) ) ;
#46131=CARTESIAN_POINT ( 'NONE',  ( 2.604371601988999974, -77.51379954448199783, -10.72853197743999942 ) ) ;
#46139=CARTESIAN_POINT ( 'NONE',  ( 6.064331118019999245, -78.60094147377398599, -9.105586440592000841 ) ) ;
#46143=ORIENTED_EDGE ( 'NONE', *, *, #12879, .F. ) ;
#46148=EDGE_CURVE ( 'NONE', #3255, #30832, #6334, .T. ) ;
#46153=CARTESIAN_POINT ( 'NONE',  ( 9.400066902809999903, -78.32495809405799037, -0.4999367261865000356 ) ) ;
#46159=DIRECTION ( 'NONE',  ( 1.000000000000000000, 0.000000000000000000, 0.000000000000000000 ) ) ;
#46163=CARTESIAN_POINT ( 'NONE',  ( -1.297526016723000053, -78.42511598777798554, -10.89864408161000142 ) ) ;
#46189=ORIENTED_EDGE ( 'NONE', *, *, #39701, .F. ) ;
#46190=EDGE_LOOP ( 'NONE', ( #53404, #14853, #37885, #39702 ) ) ;
#46193=ORIENTED_EDGE ( 'NONE', *, *, #14062, .F. ) ;
#46199=CARTESIAN_POINT ( 'NONE',  ( 7.050495581552580049, -78.29403130279574441, -5.987855718153151763 ) ) ;
#46204=CARTESIAN_POINT ( 'NONE',  ( -8.449677353798556112, -77.56661759170884807, 3.770595868082258217 ) ) ;
#46208=CARTESIAN_POINT ( 'NONE',  ( 5.091895231007000255, -78.60089172978399574, 8.260951054388000259 ) ) ;
#46217=CIRCLE ( 'NONE', #49009, 2.600000000000000089 ) ;
#46230=CARTESIAN_POINT ( 'NONE',  ( -3.399186938124999724, -80.19999999999998863, -10.46162167925000119 ) ) ;
#46239=CARTESIAN_POINT ( 'NONE',  ( -0.008314555494097999877, -77.61812138891799862, 11.16535427852999973 ) ) ;
#46251=ORIENTED_EDGE ( 'NONE', *, *, #23582, .F. ) ;
#46252=ORIENTED_EDGE ( 'NONE', *, *, #54364, .F. ) ;
#46254=EDGE_CURVE ( 'NONE', #1613, #604, #47657, .T. ) ;
#46260=VERTEX_POINT ( 'NONE', #7205 ) ;
#46274=CARTESIAN_POINT ( 'NONE',  ( -8.592462595181881824, -78.31143903816993657, 4.510367428545268176 ) ) ;
#46281=CARTESIAN_POINT ( 'NONE',  ( 5.893929754856348957, -78.77983637771299641, -7.187357691034195639 ) ) ;
#46285=CARTESIAN_POINT ( 'NONE',  ( -5.045463033963281774, -80.18718913546477722, -9.777363391122731784 ) ) ;
#46293=CARTESIAN_POINT ( 'NONE',  ( 5.220449009264826579, -79.99999999999997158, 7.789606664612244380 ) ) ;
#46304=CARTESIAN_POINT ( 'NONE',  ( -10.76076152244900719, -78.11906335555218561, -2.634765227118816444 ) ) ;
#46306=CARTESIAN_POINT ( 'NONE',  ( -7.357853812480288802, -79.78374948186821314, 8.079057253869311950 ) ) ;
#46311=CARTESIAN_POINT ( 'NONE',  ( 7.864210892918562124, -78.30589158093161473, -4.886453465047767786 ) ) ;
#46315=CARTESIAN_POINT ( 'NONE',  ( -7.148970245326999873, -78.95149595525998620, -6.453327391511999522 ) ) ;
#46317=CARTESIAN_POINT ( 'NONE',  ( -7.000000000000000000, -80.99999999999998579, -1.199999999999970424 ) ) ;
#46326=ORIENTED_EDGE ( 'NONE', *, *, #48256, .T. ) ;
#46334=CARTESIAN_POINT ( 'NONE',  ( 9.226480760116999136, -79.06100957289298492, -2.263195259622999611 ) ) ;
#46339=ORIENTED_EDGE ( 'NONE', *, *, #22695, .F. ) ;
#46354=EDGE_CURVE ( 'NONE', #40498, #22275, #48305, .T. ) ;
#46365=CARTESIAN_POINT ( 'NONE',  ( -9.590711338355999871, -77.33019948661798537, -0.1262585230650999923 ) ) ;
#46371=CARTESIAN_POINT ( 'NONE',  ( 9.697485508432000856, -79.02821424072898537, 0.9045115177663000106 ) ) ;
#46381=CARTESIAN_POINT ( 'NONE',  ( 2.550499813263000348, -78.63411711912299040, -10.67515654612000020 ) ) ;
#46384=CARTESIAN_POINT ( 'NONE',  ( 5.784847688057999981, -79.31909213876200226, -7.749218217290000155 ) ) ;
#46417=CARTESIAN_POINT ( 'NONE',  ( 7.271493354192070768, -77.40312800509396141, 5.718980060901933449 ) ) ;
#46418=CARTESIAN_POINT ( 'NONE',  ( 7.528714304401000312, -78.17517044313399310, -8.074838600060001426 ) ) ;
#46427=CARTESIAN_POINT ( 'NONE',  ( 9.601044633201999190, -79.21897326909299863, 5.244783912358999878 ) ) ;
#46433=ORIENTED_EDGE ( 'NONE', *, *, #41654, .F. ) ;
#46439=VECTOR ( 'NONE', #19366, 1000.000000000000227 ) ;
#46443=CARTESIAN_POINT ( 'NONE',  ( -0.5382333298950999767, -77.69963385321997862, -9.397951872088000869 ) ) ;
#46453=CARTESIAN_POINT ( 'NONE',  ( 10.97550047727999889, -78.12021830712397730, 0.05101033830554000531 ) ) ;
#46460=EDGE_CURVE ( 'NONE', #30580, #36425, #20891, .T. ) ;
#46467=DIRECTION ( 'NONE',  ( 0.000000000000000000, 1.000000000000000000, 0.000000000000000000 ) ) ;
#46468=AXIS2_PLACEMENT_3D ( 'NONE', #47596, #20130, #38989 ) ;
#46477=SURFACE_STYLE_FILL_AREA ( #28428 ) ;
#46488=CARTESIAN_POINT ( 'NONE',  ( 0.000000000000000000, -74.64999999999999147, 0.000000000000000000 ) ) ;
#46493=CARTESIAN_POINT ( 'NONE',  ( 7.468847837488564068, -78.29994358424977463, -5.456927524485993608 ) ) ;
#46497=CARTESIAN_POINT ( 'NONE',  ( -9.207928684727265889, -77.59252129394877784, 0.8882674814189085444 ) ) ;
#46501=CARTESIAN_POINT ( 'NONE',  ( 9.690463944985998168, -78.51562024239699156, -0.5153813127049999832 ) ) ;
#46524=AXIS2_PLACEMENT_3D ( 'NONE', #33025, #45472, #51071 ) ;
#46527=CARTESIAN_POINT ( 'NONE',  ( -1.478176540950000062, -79.50581479701997978, -9.528551035451000573 ) ) ;
#46534=CARTESIAN_POINT ( 'NONE',  ( -3.004044512312000315, -77.78272331745698409, -10.86653804020000003 ) ) ;
#46543=FACE_BOUND ( 'NONE', #15062, .T. ) ;
#46564=EDGE_LOOP ( 'NONE', ( #31334, #4641, #28290, #58349 ) ) ;
#46570=CARTESIAN_POINT ( 'NONE',  ( -4.475245744599999576, -78.83685813009675769, -8.610626265545000990 ) ) ;
#46573=CIRCLE ( 'NONE', #48407, 9.250000000000000000 ) ;
#46575=CARTESIAN_POINT ( 'NONE',  ( -4.551864695536657734, -78.68412335589445661, -8.054303700184762604 ) ) ;
#46579=CARTESIAN_POINT ( 'NONE',  ( -6.819272535855454009, -80.17227384770239951, -8.636012267496480987 ) ) ;
#46590=CARTESIAN_POINT ( 'NONE',  ( -2.421146232948727217, -79.70460708974083275, -9.008471024255291226 ) ) ;
#46593=EDGE_CURVE ( 'NONE', #28511, #13326, #57984, .T. ) ;
#46597=CARTESIAN_POINT ( 'NONE',  ( -10.64366519981685322, -77.46551422760700234, -2.049234529886447831 ) ) ;
#46598=CARTESIAN_POINT ( 'NONE',  ( 7.788493169598003085, -78.66221640831159334, 7.733265204867000087 ) ) ;
#46604=CARTESIAN_POINT ( 'NONE',  ( 7.703316849872579475, -78.30345904569475124, -5.123123729073115307 ) ) ;
#46607=CARTESIAN_POINT ( 'NONE',  ( 9.415855586929327004, -78.95131608867242790, 0.09954321913080461937 ) ) ;
#46608=CARTESIAN_POINT ( 'NONE',  ( -2.552693750765000047, -78.49671468919598283, -9.286385980553001573 ) ) ;
#46618=CARTESIAN_POINT ( 'NONE',  ( -11.38514561087999866, -79.66561849808098827, 1.960531219681000081 ) ) ;
#46619=EDGE_LOOP ( 'NONE', ( #9819, #26321 ) ) ;
#46621=CARTESIAN_POINT ( 'NONE',  ( 5.377062312294000002, -77.72131800370499377, -9.963906840203000215 ) ) ;
#46627=CARTESIAN_POINT ( 'NONE',  ( 3.366547962069000199, -79.54345705591799742, -9.168809063548000182 ) ) ;
#46641=CARTESIAN_POINT ( 'NONE',  ( -9.467663399184001349, -77.16228479622688496, 0.6244416360999999194 ) ) ;
#46663=CARTESIAN_POINT ( 'NONE',  ( 8.584722543520001636, -79.05663806985799624, 4.148835967969999317 ) ) ;
#46665=CARTESIAN_POINT ( 'NONE',  ( -8.160216723678894724, -77.11145833334454380, 4.702279489708627302 ) ) ;
#46672=CARTESIAN_POINT ( 'NONE',  ( -9.008856688516557298, -78.07931792999902143, 2.421010749684254115 ) ) ;
#46676=CARTESIAN_POINT ( 'NONE',  ( -4.985523414424999800, -78.57793241045699517, -9.777963635945001286 ) ) ;
#46681=CARTESIAN_POINT ( 'NONE',  ( -4.460001432529999477, -79.72991637959898981, -8.580398187795999831 ) ) ;
#46698=CARTESIAN_POINT ( 'NONE',  ( 10.94426510211266645, -78.70613393985135531, 0.8311920584813466961 ) ) ;
#46717=VERTEX_POINT ( 'NONE', #48679 ) ;
#46718=CARTESIAN_POINT ( 'NONE',  ( 9.209373452604401322, -77.35755538323695646, 0.8669182893996996153 ) ) ;
#46719=CARTESIAN_POINT ( 'NONE',  ( 2.604371601988999974, -77.63440539582299493, -10.72853197743999942 ) ) ;
#46723=CARTESIAN_POINT ( 'NONE',  ( -9.685922776715001348, -77.38557761206399732, 0.5943755449006998814 ) ) ;
#46726=DIRECTION ( 'NONE',  ( 0.000000000000000000, -1.000000000000000000, 0.000000000000000000 ) ) ;
#46728=CARTESIAN_POINT ( 'NONE',  ( -10.98042387750000159, -79.00192546654999148, -1.228081885531999928 ) ) ;
#46741=CARTESIAN_POINT ( 'NONE',  ( 1.825776387079000029, -78.43865341057399121, 9.234594473601999809 ) ) ;
#46752=CARTESIAN_POINT ( 'NONE',  ( -4.985523414424999800, -78.39702363344498792, -9.777963635945001286 ) ) ;
#46759=DIRECTION ( 'NONE',  ( -3.675129381003999189E-09, -0.9999999999999997780, 2.168720766502999921E-08 ) ) ;
#46768=CARTESIAN_POINT ( 'NONE',  ( -9.469606800734000629, -80.05752053325198858, 5.597012331546999953 ) ) ;
#46769=ORIENTED_EDGE ( 'NONE', *, *, #45287, .F. ) ;
#46770=FACE_OUTER_BOUND ( 'NONE', #53788, .T. ) ;
#46783=DIRECTION ( 'NONE',  ( 0.000000000000000000, -1.000000000000000000, 0.000000000000000000 ) ) ;
#46786=ADVANCED_FACE ( 'NONE', ( #56954 ), #30354, .T. ) ;
#46787=CARTESIAN_POINT ( 'NONE',  ( 5.874230328676101287, -78.27988767441337359, -7.145232025174067303 ) ) ;
#46795=CARTESIAN_POINT ( 'NONE',  ( -9.702231720816998362, -78.77143470455798990, -0.1934140619087000024 ) ) ;
#46798=FACE_OUTER_BOUND ( 'NONE', #21063, .T. ) ;
#46812=AXIS2_PLACEMENT_3D ( 'NONE', #1231, #50232, #23057 ) ;
#46819=CARTESIAN_POINT ( 'NONE',  ( -3.765737196849845869, -77.19487930045538349, -8.507847610243468139 ) ) ;
#46820=CARTESIAN_POINT ( 'NONE',  ( 9.582741442650998920, -79.65192808831000093, 1.072080763990999941 ) ) ;
#46824=DIRECTION ( 'NONE',  ( 0.000000000000000000, 1.000000000000000000, 0.000000000000000000 ) ) ;
#46825=CARTESIAN_POINT ( 'NONE',  ( -0.008395553423636001322, -77.55424564813398547, 11.27412384287999991 ) ) ;
#46836=EDGE_CURVE ( 'NONE', #50939, #54943, #7395, .T. ) ;
#46844=ORIENTED_EDGE ( 'NONE', *, *, #22695, .T. ) ;
#46850=EDGE_LOOP ( 'NONE', ( #9295, #28496, #31233, #9770 ) ) ;
#46861=CARTESIAN_POINT ( 'NONE',  ( -9.022250383429000209, -78.78001047183876437, -3.573472734901999903 ) ) ;
#46864=CARTESIAN_POINT ( 'NONE',  ( 9.655991824031183057, -79.60868651084126668, 1.080275738811528718 ) ) ;
#46867=CARTESIAN_POINT ( 'NONE',  ( -2.116425671828475519, -78.70676334617536440, -9.010145557416606721 ) ) ;
#46886=CARTESIAN_POINT ( 'NONE',  ( -1.148062820858973154, -78.06710658568482586, -10.77713783125740044 ) ) ;
#46888=CARTESIAN_POINT ( 'NONE',  ( 10.71556987377000070, -79.61735645562259833, 2.374990294079000197 ) ) ;
#46895=CARTESIAN_POINT ( 'NONE',  ( 8.278135427829594661, -78.31322909081512762, -4.127880705928267169 ) ) ;
#46899=CARTESIAN_POINT ( 'NONE',  ( 4.561861969681999973, -77.66539556192998361, 8.605179316909000065 ) ) ;
#46906=CARTESIAN_POINT ( 'NONE',  ( -9.250000000000000000, -79.09999999999999432, 1.813240672189999963E-14 ) ) ;
#46911=ORIENTED_EDGE ( 'NONE', *, *, #27540, .T. ) ;
#46913=CARTESIAN_POINT ( 'NONE',  ( -1.359921359492999970, -78.00530199648000007, 11.35132765128000010 ) ) ;
#46920=CARTESIAN_POINT ( 'NONE',  ( -9.687172913667000174, -80.26021482710652322, -1.248753675804000096 ) ) ;
#46925=ORIENTED_EDGE ( 'NONE', *, *, #17552, .T. ) ;
#46929=CARTESIAN_POINT ( 'NONE',  ( 0.000000000000000000, -75.19999999999998863, 0.000000000000000000 ) ) ;
#46933=CARTESIAN_POINT ( 'NONE',  ( -6.089781427445000617, -77.04533417779047966, 7.498689922205000080 ) ) ;
#46940=CARTESIAN_POINT ( 'NONE',  ( 2.905710011617722355, -77.07499999989397566, -8.943793187339698747 ) ) ;
#46949=ORIENTED_EDGE ( 'NONE', *, *, #500, .T. ) ;
#46951=CARTESIAN_POINT ( 'NONE',  ( -3.802343155576000111, -76.98502847823358763, -8.627496936359001722 ) ) ;
#46952=DIRECTION ( 'NONE',  ( 1.000000000000000000, 0.000000000000000000, 0.000000000000000000 ) ) ;
#46956=CARTESIAN_POINT ( 'NONE',  ( -7.735308924444000311, -77.32278449298998169, -5.918161214274000770 ) ) ;
#46963=CARTESIAN_POINT ( 'NONE',  ( -7.396685970965884316, -78.04807098620916861, 5.684396067267562636 ) ) ;
#46967=CARTESIAN_POINT ( 'NONE',  ( -2.801260334388999684, -79.18052108146299872, -9.140240961675001330 ) ) ;
#46978=VECTOR ( 'NONE', #12546, 1000.000000000000000 ) ;
#46985=CARTESIAN_POINT ( 'NONE',  ( -8.758933146614412024, -79.90041885450349923, 6.307249761326839455 ) ) ;
#47004=CARTESIAN_POINT ( 'NONE',  ( 8.796548128639548381, -77.37506330577387814, 2.860527516076478260 ) ) ;
#47005=CARTESIAN_POINT ( 'NONE',  ( 8.680753609988000719, -77.79345393914999818, 6.821192461343000168 ) ) ;
#47007=LINE ( 'NONE', #6537, #48502 ) ;
#47013=CARTESIAN_POINT ( 'NONE',  ( 10.62704985177000161, -78.72100192322298540, -3.023855997759000047 ) ) ;
#47019=CARTESIAN_POINT ( 'NONE',  ( -9.993863819922085057, -77.19999999999998863, 4.482211430344825054 ) ) ;
#47028=CARTESIAN_POINT ( 'NONE',  ( -5.574784109570000368, -78.21829086006698617, -7.719595738358999704 ) ) ;
#47039=CARTESIAN_POINT ( 'NONE',  ( 0.1291013223160000223, -79.18360955475999674, 10.97485077029999978 ) ) ;
#47048=CARTESIAN_POINT ( 'NONE',  ( 2.421167930323324224, -78.14583333333331439, -9.009247259181924150 ) ) ;
#47051=CARTESIAN_POINT ( 'NONE',  ( 7.410162453131999172, -78.99706562342599625, 8.486367113423000319 ) ) ;
#47075=CARTESIAN_POINT ( 'NONE',  ( 3.541191267721896185, -78.25630510186675792, -8.545282945131162933 ) ) ;
#47080=CARTESIAN_POINT ( 'NONE',  ( -8.814863682110420484, -77.57551665829541321, 2.803737005584837849 ) ) ;
#47082=EDGE_CURVE ( 'NONE', #45667, #15896, #47405, .T. ) ;
#47084=CARTESIAN_POINT ( 'NONE',  ( 0.8618009059429999619, -78.40192492588099071, -9.665816497589000633 ) ) ;
#47093=CARTESIAN_POINT ( 'NONE',  ( -10.69999999997999929, -81.80000000002199556, 2.760601855093000384E-10 ) ) ;
#47096=AXIS2_PLACEMENT_3D ( 'NONE', #17266, #21695, #30833 ) ;
#47099=CARTESIAN_POINT ( 'NONE',  ( -10.83098670370000072, -80.42828225638099582, 0.1115786215289999994 ) ) ;
#47104=ORIENTED_EDGE ( 'NONE', *, *, #7570, .T. ) ;
#47109=CARTESIAN_POINT ( 'NONE',  ( 6.321655259472999333, -79.77424914560899083, 7.136321001271999975 ) ) ;
#47114=EDGE_CURVE ( 'NONE', #22275, #53170, #47587, .T. ) ;
#47119=CARTESIAN_POINT ( 'NONE',  ( 9.730158407969000223, -77.59631800370499377, 5.250919032787999541 ) ) ;
#47122=CARTESIAN_POINT ( 'NONE',  ( -5.190928442694000111, -77.94229427166699509, 7.852735600434000318 ) ) ;
#47135=ORIENTED_EDGE ( 'NONE', *, *, #6048, .T. ) ;
#47150=AXIS2_PLACEMENT_3D ( 'NONE', #26586, #39887, #53474 ) ;
#47153=AXIS2_PLACEMENT_3D ( 'NONE', #20467, #25460, #56766 ) ;
#47155=CARTESIAN_POINT ( 'NONE',  ( 5.417083560472998549, -78.92212961748376188, -8.051455326762999576 ) ) ;
#47158=CARTESIAN_POINT ( 'NONE',  ( -2.935661446561999899, -76.94999999999998863, -9.035036904803998681 ) ) ;
#47160=CARTESIAN_POINT ( 'NONE',  ( -7.373862043355542184, -78.65167919242699668, -5.586005179260620679 ) ) ;
#47162=CARTESIAN_POINT ( 'NONE',  ( -10.90052211673698324, -80.11089183211095133, -1.475228759022814584 ) ) ;
#47178=CARTESIAN_POINT ( 'NONE',  ( -9.726444407485992372, -77.91415937600359598, 4.784104274147578550 ) ) ;
#47180=CARTESIAN_POINT ( 'NONE',  ( -0.6514878906251001522, -79.72972587295357982, 10.95625855609000077 ) ) ;
#47186=CARTESIAN_POINT ( 'NONE',  ( 0.000000000000000000, -79.99999999999998579, 0.000000000000000000 ) ) ;
#47190=CARTESIAN_POINT ( 'NONE',  ( 3.260206397764000119, -78.17702448625199452, 9.177731198418999981 ) ) ;
#47196=VECTOR ( 'NONE', #41368, 1000.000000000000000 ) ;
#47203=DIRECTION ( 'NONE',  ( -0.7071067811865474617, -0.7071067811865474617, 9.259177001912613574E-10 ) ) ;
#47207=CARTESIAN_POINT ( 'NONE',  ( -8.741845958662000982, -77.56508549249599582, 7.367642417069999894 ) ) ;
#47212=CARTESIAN_POINT ( 'NONE',  ( 5.411006671257999834, -79.45843616023900324, 8.131518144102999557 ) ) ;
#47216=CIRCLE ( 'NONE', #9474, 10.69999999999999929 ) ;
#47224=CARTESIAN_POINT ( 'NONE',  ( -9.489900988576000174, -77.27852983129099584, -0.9230819386030000295 ) ) ;
#47226=CARTESIAN_POINT ( 'NONE',  ( 1.439896632895333539, -79.73541666666666572, -10.99999999999999822 ) ) ;
#47229=AXIS2_PLACEMENT_3D ( 'NONE', #9398, #24722, #37123 ) ;
#47231=CARTESIAN_POINT ( 'NONE',  ( 3.595196481342544548, -77.09062499990726280, -8.672428026956840341 ) ) ;
#47244=CARTESIAN_POINT ( 'NONE',  ( 6.263319273733999992, -78.09022787947299094, 7.458587492396000052 ) ) ;
#47246=CARTESIAN_POINT ( 'NONE',  ( -7.412025882568599400, -77.76672174443258712, -8.233944902729593451 ) ) ;
#47256=CARTESIAN_POINT ( 'NONE',  ( -10.96076829013453136, -80.09369723771236238, 0.9252934957875924571 ) ) ;
#47257=CARTESIAN_POINT ( 'NONE',  ( 9.526202310737001966, -79.87930701263098854, -1.663220358726000159 ) ) ;
#47273=CONICAL_SURFACE ( 'NONE', #11440, 1.099999997149000430, 0.7853981633972997312 ) ;
#47277=CARTESIAN_POINT ( 'NONE',  ( -5.726462542197000793, -79.78469283625899777, -7.912542777261000637 ) ) ;
#47291=VERTEX_POINT ( 'NONE', #38686 ) ;
#47295=CARTESIAN_POINT ( 'NONE',  ( 4.201985891154212283, -77.26254768197554768, -8.240472212907164362 ) ) ;
#47299=UNCERTAINTY_MEASURE_WITH_UNIT (LENGTH_MEASURE( 1.000000000000000082E-05 ), #5710, 'distance_accuracy_value', 'NONE');
#47305=CARTESIAN_POINT ( 'NONE',  ( 6.124581921013000141, -78.66481721455799914, -9.196052954390001588 ) ) ;
#47308=CARTESIAN_POINT ( 'NONE',  ( 0.2063173652470433606, -77.19999999999998863, 10.79676918780386075 ) ) ;
#47318=CARTESIAN_POINT ( 'NONE',  ( 3.187402732789999860, -77.99090022703498448, 8.972783294553000388 ) ) ;
#47331=CARTESIAN_POINT ( 'NONE',  ( 0.1291013223160000223, -79.24391248043099267, 10.97485077029999978 ) ) ;
#47332=DIRECTION ( 'NONE',  ( -1.000000000000000000, 0.000000000000000000, 0.000000000000000000 ) ) ;
#47339=CARTESIAN_POINT ( 'NONE',  ( 11.00000000000000000, -77.94999999999998863, 0.000000000000000000 ) ) ;
#47342=CARTESIAN_POINT ( 'NONE',  ( -10.93895610016999953, -78.65995737143398969, 2.695955081989000135 ) ) ;
#47351=CARTESIAN_POINT ( 'NONE',  ( 11.00000000000000000, -79.34999999999999432, -1.064824513673000067E-14 ) ) ;
#47357=CARTESIAN_POINT ( 'NONE',  ( -0.05512383893429553122, -79.87451577342567077, -9.559639413446380019 ) ) ;
#47359=CONICAL_SURFACE ( 'NONE', #52980, 1.099999997148999986, 0.7853981633972997312 ) ;
#47364=CARTESIAN_POINT ( 'NONE',  ( 0.6905870083389051839, -78.23098341495615671, -9.225493071672193679 ) ) ;
#47367=VERTEX_POINT ( 'NONE', #3061 ) ;
#47372=CARTESIAN_POINT ( 'NONE',  ( -1.565122400816999937, -78.71804231371298499, 9.577113408380000692 ) ) ;
#47378=DIRECTION ( 'NONE',  ( 0.000000000000000000, -1.000000000000000000, 0.000000000000000000 ) ) ;
#47382=CARTESIAN_POINT ( 'NONE',  ( -8.111819378804783653, -80.34583333334180111, -7.301249762614178351 ) ) ;
#47387=CARTESIAN_POINT ( 'NONE',  ( -10.61587359353999993, -80.44003597815999740, -1.456403148199000075 ) ) ;
#47397=CARTESIAN_POINT ( 'NONE',  ( -9.280666835437999751, -79.91493201263098456, -2.616774452598999989 ) ) ;
#47400=CARTESIAN_POINT ( 'NONE',  ( 3.031642507359964878, -79.19956947028450145, 9.231160939620027150 ) ) ;
#47403=CARTESIAN_POINT ( 'NONE',  ( 11.00000000000000711, -77.43958333333331723, -1.439896632895300010 ) ) ;
#47405=CIRCLE ( 'NONE', #53954, 9.549999999999998934 ) ;
#47406=CARTESIAN_POINT ( 'NONE',  ( -10.84896630757000047, -77.86011170514498758, 1.467873659019000021 ) ) ;
#47412=CARTESIAN_POINT ( 'NONE',  ( 5.491552160713999875, -77.09679918850338254, 7.961786551375001686 ) ) ;
#47413=CARTESIAN_POINT ( 'NONE',  ( 2.421167930323344653, -78.35416666666665719, 9.009247259181915268 ) ) ;
#47417=CARTESIAN_POINT ( 'NONE',  ( 0.000000000000000000, -75.09999999979599750, 0.000000000000000000 ) ) ;
#47434=VERTEX_POINT ( 'NONE', #28377 ) ;
#47451=CONICAL_SURFACE ( 'NONE', #18186, 4.199999999630000147, 0.7853981633972997312 ) ;
#47453=CARTESIAN_POINT ( 'NONE',  ( -5.007122319500682650, -78.67959078829761665, -7.777765833668380147 ) ) ;
#47473=CARTESIAN_POINT ( 'NONE',  ( -10.67274964942681414, -77.93965057761698745, 1.462407073126524848 ) ) ;
#47475=DIRECTION ( 'NONE',  ( 0.000000000000000000, -1.000000000000000000, 0.000000000000000000 ) ) ;
#47483=CARTESIAN_POINT ( 'NONE',  ( 8.393017115181999444, -79.24276232907497786, 4.056188317180000169 ) ) ;
#47488=ORIENTED_EDGE ( 'NONE', *, *, #12887, .T. ) ;
#47493=CARTESIAN_POINT ( 'NONE',  ( 9.250000000000003553, -77.73965344036420788, -1.202673002443502170 ) ) ;
#47495=ORIENTED_EDGE ( 'NONE', *, *, #10797, .F. ) ;
#47497=CARTESIAN_POINT ( 'NONE',  ( 10.83522510763000035, -77.34497724050399370, -3.646917633351999921 ) ) ;
#47506=CARTESIAN_POINT ( 'NONE',  ( 5.411006671257999834, -79.33858331678850107, 8.131518144102999557 ) ) ;
#47510=ORIENTED_EDGE ( 'NONE', *, *, #25068, .T. ) ;
#47523=CARTESIAN_POINT ( 'NONE',  ( 7.396918292183153554, -77.80208333333332860, 5.684557159767984480 ) ) ;
#47526=DIRECTION ( 'NONE',  ( 1.000000000000000000, 0.000000000000000000, 0.000000000000000000 ) ) ;
#47527=CARTESIAN_POINT ( 'NONE',  ( 0.000000000000000000, -80.39687500001899423, 0.000000000000000000 ) ) ;
#47530=AXIS2_PLACEMENT_3D ( 'NONE', #15742, #53488, #26322 ) ;
#47531=ADVANCED_FACE ( 'NONE', ( #2705 ), #12415, .F. ) ;
#47537=CARTESIAN_POINT ( 'NONE',  ( 0.000000000000000000, -78.49999999999998579, 0.000000000000000000 ) ) ;
#47544=CARTESIAN_POINT ( 'NONE',  ( -9.312499999988999022, -77.13750000001088836, -2.050180145195999796E-09 ) ) ;
#47546=DIRECTION ( 'NONE',  ( 0.000000000000000000, -1.000000000000000000, 0.000000000000000000 ) ) ;
#47549=CARTESIAN_POINT ( 'NONE',  ( 7.257622347668946539, -79.44361411732418787, -6.227379948060659309 ) ) ;
#47552=CARTESIAN_POINT ( 'NONE',  ( -10.47624881337006109, -80.07551940951682923, 3.353468735377274079 ) ) ;
#47553=CARTESIAN_POINT ( 'NONE',  ( 6.970637445331999693, -79.95400232914698790, 6.702596717548000349 ) ) ;
#47555=CARTESIAN_POINT ( 'NONE',  ( 4.658475568430830549, -79.16666666666665719, -8.082524092276877070 ) ) ;
#47570=CIRCLE ( 'NONE', #37168, 1.199999999999999734 ) ;
#47571=CARTESIAN_POINT ( 'NONE',  ( -8.396223008680999911, -79.75222017800098229, -4.990405176070999538 ) ) ;
#47579=CARTESIAN_POINT ( 'NONE',  ( 0.000000000000000000, -76.19999999999998863, 0.000000000000000000 ) ) ;
#47587=B_SPLINE_CURVE_WITH_KNOTS ( 'NONE', 3,
 ( #15280, #6718, #2019, #38000, #19427, #32978, #24726, #32686, #51608, #14397, #11165, #56026, #15575, #28257, #19718, #9991, #55439, #42739, #33570, #50439, #51315, #10276, #23842, #37419, #2302, #10873, #37714, #27970, #20299, #38293, #51024, #33273, #46020, #5541, #55139, #23551, #41566, #46895, #1148, #28556, #50736, #46311, #46604, #5836, #41859, #1436, #14980, #24137, #6422, #42156, #24437, #46493, #24325, #41455, #28737, #19901, #46199, #42040, #42341, #10457, #28147, #24027, #1907, #37893, #1609, #6603, #19601, #37307, #1040, #33160, #51206, #41159, #14579, #10758, #45903, #55617, #46787, #6311, #37018, #36726, #55917, #50620, #32572, #32282, #37601, #5435, #15468, #51497, #10170, #33459, #50325, #5724, #23443, #55323, #15165, #9877, #23734, #41748, #28444, #19025, #11054, #29036, #6017, #47075, #753, #18732, #54740, #14286, #27857, #55032, #1323, #19317, #14867, #32864, #50909, #20762, #7761, #7475, #47364, #39049, #25765, #56205, #16624, #12472, #42920, #43785, #47658, #38185, #34609, #39343, #57350, #24615, #15753, #29602, #2764, #51787, #20479, #11337, #29315, #16047, #52070, #11628, #7184, #25184, #34320, #52357, #11908, #54092, #36070, #9214, #3897, #17481, #13039, #390, #44941, #53799, #26042, #27200, #13630, #26608, #13333, #45238, #31037, #26330, #31627, #49669, #35468, #48786, #18367, #44645, #4785, #40208, #22787, #40795, #36360, #54387, #57924, #40506, #12756, #30752, #31328, #21900, #13924, #17187, #31919, #35177, #8044, #44066, #3614, #49373, #21620, #4497, #39624, #57632, #39910, #22197, #53208, #8331, #44344, #22495 ),
 .UNSPECIFIED., .F., .F.,
 ( 4, 2, 2, 2, 1, 1, 2, 2, 2, 2, 2, 2, 2, 2, 1, 2, 2, 1, 2, 2, 1, 1, 2, 2, 2, 2, 2, 2, 1, 2, 2, 2, 2, 1, 2, 1, 1, 1, 2, 2, 2, 1, 1, 1, 2, 2, 2, 2, 1, 1, 1, 1, 2, 2, 2, 2, 2, 1, 1, 1, 1, 1, 2, 2, 2, 2, 1, 1, 1, 1, 2, 2, 2, 2, 1, 1, 2, 2, 2, 2, 1, 1, 1, 1, 1, 2, 2, 2, 2, 2, 1, 1, 1, 1, 1, 2, 2, 2, 2, 2, 1, 1, 1, 1, 2, 2, 2, 1, 1, 1, 1, 2, 2, 2, 2, 1, 1, 1, 1, 1, 2, 2, 2, 2, 2, 4 ),
 ( 0.000000000000000000, 0.03125000000000939526, 0.03515625000001058181, 0.03613281250001086631, 0.03710937500001114386, 0.03906250000001169898, 0.04687500000001394718, 0.06250000000001841582, 0.07031250000002067790, 0.07812500000002293998, 0.09375000000002757516, 0.1015625000000298650, 0.1054687500000310307, 0.1074218750000315997, 0.1093750000000321687, 0.1250000000000367206, 0.1406250000000412725, 0.1425781250000418277, 0.1428222656250419109, 0.1430664062500419942, 0.1435546875000421330, 0.1445312500000424105, 0.1484375000000435485, 0.1562500000000458245, 0.1875000000000551503, 0.1953125000000574818, 0.1962890625000577871, 0.1972656250000581202, 0.1992187500000587586, 0.2031250000000600631, 0.2187500000000654476, 0.2226562500000668077, 0.2265625000000681399, 0.2343750000000707490, 0.2421875000000733025, 0.2460937500000746070, 0.2480468750000752176, 0.2490234375000754674, 0.2495117187500755784, 0.2500000000000756617, 0.2656250000000759393, 0.2734375000000760503, 0.2773437500000761058, 0.2792968750000762168, 0.2802734375000762723, 0.2812500000000763278, 0.2968750000000785483, 0.3046875000000796585, 0.3085937500000802136, 0.3105468750000805467, 0.3115234375000806577, 0.3120117187500807687, 0.3122558593750808242, 0.3125000000000808797, 0.3437500000000918154, 0.3593750000000973110, 0.3671875000001000866, 0.3710937500001014189, 0.3730468750001020295, 0.3740234375001024736, 0.3745117187501025291, 0.3747558593751025846, 0.3748779296876025846, 0.3750000000001026401, 0.4062500000001136868, 0.4218750000001192380, 0.4296875000001220135, 0.4335937500001234013, 0.4355468750001241229, 0.4365234375001244560, 0.4370117187501246780, 0.4375000000001248446, 0.4687500000001362799, 0.4843750000001419420, 0.4921875000001448286, 0.4960937500001462164, 0.4980468750001468825, 0.5000000000001475486, 0.5312500000001589839, 0.5468750000001646461, 0.5546875000001674216, 0.5585937500001688649, 0.5605468750001695311, 0.5615234375001699751, 0.5620117187501700862, 0.5622558593751701972, 0.5625000000001701972, 0.5937500000001844080, 0.6093750000001915135, 0.6171875000001950662, 0.6210937500001968425, 0.6230468750001977307, 0.6240234375001981748, 0.6245117187501982858, 0.6247558593751983969, 0.6248779296876983969, 0.6250000000001985079, 0.6562500000001916245, 0.6718750000001881828, 0.6796875000001866285, 0.6835937500001857403, 0.6855468750001852962, 0.6865234375001851852, 0.6870117187501850742, 0.6872558593751850742, 0.6875000000001850742, 0.7031250000001876277, 0.7109375000001888489, 0.7148437500001895151, 0.7167968750001898481, 0.7177734375001900702, 0.7182617187501900702, 0.7187500000001900702, 0.7343750000001922906, 0.7421875000001932898, 0.7460937500001938449, 0.7480468750001942890, 0.7490234375001942890, 0.7495117187501944001, 0.7497558593751944001, 0.7498779296876944001, 0.7500000000001942890, 0.8125000000001457723, 0.8750000000000971445, 0.9375000000000486278, 1.000000000000000000 ),
 .UNSPECIFIED. ) ;
#47591=CARTESIAN_POINT ( 'NONE',  ( 4.346385276184861368, -77.26393889505689572, -8.165376318784744569 ) ) ;
#47596=CARTESIAN_POINT ( 'NONE',  ( 0.000000000000000000, -76.30000000005068728, 0.000000000000000000 ) ) ;
#47600=CARTESIAN_POINT ( 'NONE',  ( 10.34967326289000056, -78.27152425389999735, 3.868085496227999798 ) ) ;
#47606=CARTESIAN_POINT ( 'NONE',  ( -5.496145386621526185, -77.20000000000000284, 9.413364287384716533 ) ) ;
#47608=FACE_OUTER_BOUND ( 'NONE', #16111, .T. ) ;
#47612=CARTESIAN_POINT ( 'NONE',  ( 0.000000000000000000, -80.99999999999998579, -7.000000000000000000 ) ) ;
#47614=CARTESIAN_POINT ( 'NONE',  ( 8.286539809994000194, -77.93405256877699117, 4.690803151849999963 ) ) ;
#47626=CARTESIAN_POINT ( 'NONE',  ( 7.318097147681000614, -79.55292837808998740, -8.179820946710000484 ) ) ;
#47631=CARTESIAN_POINT ( 'NONE',  ( 0.000000000000000000, -74.64999999999999147, 0.000000000000000000 ) ) ;
#47635=CARTESIAN_POINT ( 'NONE',  ( -4.658475568430826996, -78.08333333333330017, -8.082524092276880623 ) ) ;
#47636=CARTESIAN_POINT ( 'NONE',  ( 11.15746894976000014, -77.99343189956698552, 0.05185606496389000286 ) ) ;
#47657=CIRCLE ( 'NONE', #20285, 2.600000000000000089 ) ;
#47658=CARTESIAN_POINT ( 'NONE',  ( -0.2780177897949673294, -78.22274903711796412, -9.249907059576116808 ) ) ;
#47663=CARTESIAN_POINT ( 'NONE',  ( -4.013128615792370901, -77.51086162448915218, 8.336612707408551870 ) ) ;
#47666=CARTESIAN_POINT ( 'NONE',  ( -4.475245744599999576, -78.91700911761597581, -8.610626265545000990 ) ) ;
#47670=CARTESIAN_POINT ( 'NONE',  ( -7.179058446792000225, -79.87950005142698728, -8.667882172381000672 ) ) ;
#47682=CARTESIAN_POINT ( 'NONE',  ( 10.67969489444999986, -80.15794665545099917, -2.920153015311000022 ) ) ;
#47689=AXIS2_PLACEMENT_3D ( 'NONE', #49086, #57365, #36086 ) ;
#47690=CARTESIAN_POINT ( 'NONE',  ( -6.734246782101999784, -79.39435458825498415, 6.748357038843000311 ) ) ;
#47696=CARTESIAN_POINT ( 'NONE',  ( -3.852910167356999871, -77.77443257914897856, 10.24742925129999982 ) ) ;
#47701=CARTESIAN_POINT ( 'NONE',  ( -8.324924863653999196, -77.28764894901499360, 4.923709561474999497 ) ) ;
#47702=CARTESIAN_POINT ( 'NONE',  ( -9.250000000000005329, -78.48958333333331439, 1.210822168571030977 ) ) ;
#47704=CARTESIAN_POINT ( 'NONE',  ( 0.000000000000000000, -76.39999999999999147, 0.000000000000000000 ) ) ;
#47721=CARTESIAN_POINT ( 'NONE',  ( 9.250000000000000000, -77.84999999999999432, 0.000000000000000000 ) ) ;
#47734=CARTESIAN_POINT ( 'NONE',  ( 8.796335266379964324, -78.50208333333334565, 6.760013919724087827 ) ) ;
#47737=CARTESIAN_POINT ( 'NONE',  ( -3.506546898566349935, -78.69415870367357968, -8.559525909970664870 ) ) ;
#47749=CARTESIAN_POINT ( 'NONE',  ( 9.250000000000000000, -78.24999999999998579, -1.152201742116999973E-14 ) ) ;
#47763=CARTESIAN_POINT ( 'NONE',  ( 8.982692273745001899, -77.67242364445598923, 3.473391639513999429 ) ) ;
#47767=VERTEX_POINT ( 'NONE', #45179 ) ;
#47771=CARTESIAN_POINT ( 'NONE',  ( -11.00000000000000000, -78.69999999999998863, 0.000000000000000000 ) ) ;
#47776=CARTESIAN_POINT ( 'NONE',  ( 1.678937288468000055, -78.23355279846498433, 10.81059606312000021 ) ) ;
#47778=CARTESIAN_POINT ( 'NONE',  ( 11.17912310309000112, -80.04393697167898836, -1.842803918785000272 ) ) ;
#47785=CARTESIAN_POINT ( 'NONE',  ( 9.767191983224998708, -79.88058071758803180, 0.05162932631433000269 ) ) ;
#47798=ADVANCED_FACE ( 'NONE', ( #15028 ), #6879, .T. ) ;
#47802=VECTOR ( 'NONE', #19755, 1000.000000000000000 ) ;
#47804=CARTESIAN_POINT ( 'NONE',  ( -4.658475568430852753, -77.91666666666665719, 8.082524092276868188 ) ) ;
#47808=DIRECTION ( 'NONE',  ( 0.000000000000000000, -1.000000000000000000, 0.000000000000000000 ) ) ;
#47820=CARTESIAN_POINT ( 'NONE',  ( 1.265244864176999995, -77.63544661340898756, 9.657062241701000360 ) ) ;
#47826=ORIENTED_EDGE ( 'NONE', *, *, #46593, .T. ) ;
#47829=CARTESIAN_POINT ( 'NONE',  ( -8.483652677471663850, -79.28772561977511657, -4.355244364560813430 ) ) ;
#47833=CARTESIAN_POINT ( 'NONE',  ( 7.920804980698999742, -79.96971083593997776, -5.924224909051000409 ) ) ;
#47835=CARTESIAN_POINT ( 'NONE',  ( 6.760013919724077169, -78.77708333333333712, -8.796335266379973206 ) ) ;
#47840=EDGE_CURVE ( 'NONE', #10899, #29444, #18595, .T. ) ;
#47846=DIRECTION ( 'NONE',  ( 0.000000000000000000, -1.000000000000000000, 0.000000000000000000 ) ) ;
#47850=CARTESIAN_POINT ( 'NONE',  ( -0.5483576180056000116, -79.33007562064699414, -9.751923335751000010 ) ) ;
#47858=CARTESIAN_POINT ( 'NONE',  ( 1.882211411147126867, -78.70937264597593241, 9.520037184477153858 ) ) ;
#47866=CARTESIAN_POINT ( 'NONE',  ( -0.7330981857557979930, -79.98140777903502396, 9.220843587065861158 ) ) ;
#47869=EDGE_LOOP ( 'NONE', ( #33304, #46949, #31741, #14751 ) ) ;
#47870=CARTESIAN_POINT ( 'NONE',  ( 7.511900341590999730, -79.80389345209998453, -8.396444939682998765 ) ) ;
#47871=CARTESIAN_POINT ( 'NONE',  ( 9.249996494687895421, -77.35002555369160859, 0.002770370553531230698 ) ) ;
#47882=CARTESIAN_POINT ( 'NONE',  ( 2.567527713034000403, -78.63672486022498731, -10.74642708485000142 ) ) ;
#47896=CARTESIAN_POINT ( 'NONE',  ( -7.921993249237998747, -78.18986703093798951, -5.283218639336999978 ) ) ;
#47904=CARTESIAN_POINT ( 'NONE',  ( -2.421167930323375295, -78.89583333333332860, 9.009247259181911716 ) ) ;
#47910=CARTESIAN_POINT ( 'NONE',  ( -10.90760146693999921, -78.87871187410598850, -1.219937219691999974 ) ) ;
#47912=CARTESIAN_POINT ( 'NONE',  ( -1.417398247622813079, -80.37838541666540948, 10.82161458338522841 ) ) ;
#47918=CARTESIAN_POINT ( 'NONE',  ( -0.9999999970599000587, -81.20000000293998710, -7.000000017349999659 ) ) ;
#47919=CARTESIAN_POINT ( 'NONE',  ( 6.760013919724038978, -78.02291666666666003, 8.796335266380001627 ) ) ;
#47920=EDGE_CURVE ( 'NONE', #1043, #409, #38959, .T. ) ;
#47921=CARTESIAN_POINT ( 'NONE',  ( 6.895942029498000281, -78.85660385176299769, -8.909260232556000858 ) ) ;
#47933=ORIENTED_EDGE ( 'NONE', *, *, #54218, .F. ) ;
#47947=CARTESIAN_POINT ( 'NONE',  ( -2.925878650339476472, -77.50071622641024760, 8.775276054172831408 ) ) ;
#47948=CARTESIAN_POINT ( 'NONE',  ( 8.680753609988000719, -77.61254516213799093, 6.821192461343000168 ) ) ;
#47951=CARTESIAN_POINT ( 'NONE',  ( 8.898653440358000211, -78.54749933893899083, -3.871004561473999850 ) ) ;
#47956=CARTESIAN_POINT ( 'NONE',  ( -10.55592303174000079, -79.89804181175900055, -3.904632140253000205 ) ) ;
#47964=CARTESIAN_POINT ( 'NONE',  ( -10.55482845722999841, -80.40477481282198369, 3.343238611526999637 ) ) ;
#47977=CARTESIAN_POINT ( 'NONE',  ( -11.00000000000000000, -77.21041666666667425, -1.439896632895322881 ) ) ;
#47981=CARTESIAN_POINT ( 'NONE',  ( -10.15589153752000051, -77.33928062571699513, -4.371041081978999543 ) ) ;
#47988=CARTESIAN_POINT ( 'NONE',  ( 5.491552160713999875, -77.03649626283258556, 7.961786551375001686 ) ) ;
#47989=CARTESIAN_POINT ( 'NONE',  ( -5.684557159767977375, -78.42708333333332860, 7.396918292183154442 ) ) ;
#47990=CARTESIAN_POINT ( 'NONE',  ( 1.439896632895286466, -77.46458333333332291, 11.00000000000000711 ) ) ;
#48000=ORIENTED_EDGE ( 'NONE', *, *, #54164, .F. ) ;
#48003=ORIENTED_EDGE ( 'NONE', *, *, #31148, .F. ) ;
#48010=ORIENTED_EDGE ( 'NONE', *, *, #5504, .T. ) ;
#48011=CARTESIAN_POINT ( 'NONE',  ( -5.684557159767956058, -79.57291666666664298, -7.396918292183169541 ) ) ;
#48018=CARTESIAN_POINT ( 'NONE',  ( 9.250000000000000000, -77.74999999999998579, 0.000000000000000000 ) ) ;
#48023=CARTESIAN_POINT ( 'NONE',  ( -11.00000000000000000, -78.69999999999998863, 0.000000000000000000 ) ) ;
#48025=CARTESIAN_POINT ( 'NONE',  ( -9.134711892043656078, -78.61273296005398947, -1.455512071036835220 ) ) ;
#48028=AXIS2_PLACEMENT_3D ( 'NONE', #28183, #5761, #1357 ) ;
#48029=CARTESIAN_POINT ( 'NONE',  ( -10.99959862783280506, -80.10247156894594411, -0.2778054206351758815 ) ) ;
#48044=CARTESIAN_POINT ( 'NONE',  ( -2.169167664939000151, -78.20037715311599413, 10.75912301088999889 ) ) ;
#48056=CARTESIAN_POINT ( 'NONE',  ( -4.391285525405000278, -79.04379552517198704, -8.449082048777999177 ) ) ;
#48060=EDGE_LOOP ( 'NONE', ( #57913, #55454, #21116, #10009 ) ) ;
#48062=CARTESIAN_POINT ( 'NONE',  ( 8.566298481405405951, -78.88243973942240927, 3.641100821265425669 ) ) ;
#48063=AXIS2_PLACEMENT_3D ( 'NONE', #32025, #5180, #13144 ) ;
#48066=CARTESIAN_POINT ( 'NONE',  ( 4.619608356761999879, -78.71112282211998945, 9.917007359391000421 ) ) ;
#48068=ADVANCED_FACE ( 'NONE', ( #43052 ), #39756, .T. ) ;
#48069=CARTESIAN_POINT ( 'NONE',  ( -7.171416948513999579, -80.31415055360498911, -8.914771748833000942 ) ) ;
#48077=CARTESIAN_POINT ( 'NONE',  ( -9.358268528169000788, -79.65327210978701089, -2.797054701638000296 ) ) ;
#48088=CARTESIAN_POINT ( 'NONE',  ( 8.646211292720670016, -78.82120266248546159, -3.287401068500848567 ) ) ;
#48090=CARTESIAN_POINT ( 'NONE',  ( -10.75000000000000000, -80.44999999999899387, 2.612557432076000154E-10 ) ) ;
#48092=CARTESIAN_POINT ( 'NONE',  ( -7.396918292183192634, -77.94791666666667140, 5.684557159767932077 ) ) ;
#48109=FACE_OUTER_BOUND ( 'NONE', #40493, .T. ) ;
#48113=CARTESIAN_POINT ( 'NONE',  ( 2.925805176656314899, -79.39985491316186028, -9.059708552875285648 ) ) ;
#48115=CARTESIAN_POINT ( 'NONE',  ( 1.491917775262641577, -79.99999999999997158, -9.368459166867951993 ) ) ;
#48118=CARTESIAN_POINT ( 'NONE',  ( -1.318181353051000038, -80.15644912722899562, 9.802870741655000941 ) ) ;
#48122=DIRECTION ( 'NONE',  ( 0.000000000000000000, 1.000000000000000000, 0.000000000000000000 ) ) ;
#48130=CARTESIAN_POINT ( 'NONE',  ( -8.613561821356000792, -77.48351239614198960, -7.003728345069999861 ) ) ;
#48135=CARTESIAN_POINT ( 'NONE',  ( -10.69999999999999929, -81.79999999999998295, 0.000000000000000000 ) ) ;
#48142=ORIENTED_EDGE ( 'NONE', *, *, #4950, .F. ) ;
#48144=CIRCLE ( 'NONE', #52842, 10.50000000000000000 ) ;
#48145=CARTESIAN_POINT ( 'NONE',  ( -1.439896632895359962, -77.58541666666667425, 10.99999999999999645 ) ) ;
#48150=DIRECTION ( 'NONE',  ( 1.000000000000000000, 0.000000000000000000, 0.000000000000000000 ) ) ;
#48153=CARTESIAN_POINT ( 'NONE',  ( 1.225466286858300391, -79.96494772406065010, 9.168303427177114884 ) ) ;
#48154=ORIENTED_EDGE ( 'NONE', *, *, #3416, .F. ) ;
#48157=CARTESIAN_POINT ( 'NONE',  ( 11.02792952375000013, -79.35441578277699648, -2.305147454016000186 ) ) ;
#48158=CARTESIAN_POINT ( 'NONE',  ( 8.300692004267670399, -77.31357384288631351, -4.110348182662033167 ) ) ;
#48165=CARTESIAN_POINT ( 'NONE',  ( -8.796335266380006956, -78.54791666666665151, 6.760013919724027431 ) ) ;
#48169=CARTESIAN_POINT ( 'NONE',  ( 0.1312417595986999919, -79.43100181365798562, 11.15680847095000061 ) ) ;
#48177=CARTESIAN_POINT ( 'NONE',  ( 0.000000000000000000, -74.64999999999999147, 0.000000000000000000 ) ) ;
#48183=CARTESIAN_POINT ( 'NONE',  ( 8.875952806245999582, -78.91941197858199075, 3.056903470501999731 ) ) ;
#48192=CARTESIAN_POINT ( 'NONE',  ( 0.000000000000000000, -74.99999999999998579, -4.799999999999999822 ) ) ;
#48195=CARTESIAN_POINT ( 'NONE',  ( 4.634563706678000550, -78.71015774810999233, 9.949112313689999709 ) ) ;
#48197=CARTESIAN_POINT ( 'NONE',  ( -8.623051981844785274, -80.41744791666556580, 6.625779411460311685 ) ) ;
#48204=CARTESIAN_POINT ( 'NONE',  ( 6.026835113838189706, -77.31868998740377208, 7.054302318249272119 ) ) ;
#48205=CARTESIAN_POINT ( 'NONE',  ( 8.082524092276869965, -78.20833333333330017, -4.658475568430838543 ) ) ;
#48206=CARTESIAN_POINT ( 'NONE',  ( -11.07910306079999962, -79.19371210375499004, -2.045094064781999954 ) ) ;
#48222=CARTESIAN_POINT ( 'NONE',  ( 9.494981342583157513, -79.50754469819568726, 0.9006174050536093212 ) ) ;
#48231=CARTESIAN_POINT ( 'NONE',  ( -6.574272315842624614, -77.53807528016541539, 6.506900208772002259 ) ) ;
#48232=CARTESIAN_POINT ( 'NONE',  ( 9.507661145905998978, -77.51711603614198509, -5.611464101879999333 ) ) ;
#48234=CARTESIAN_POINT ( 'NONE',  ( -7.456816947376000648, -78.77488997197099252, 6.210200510404999541 ) ) ;
#48238=CARTESIAN_POINT ( 'NONE',  ( -7.054457466615000172, -80.38063403548999020, -8.769379688592000122 ) ) ;
#48239=EDGE_CURVE ( 'NONE', #13840, #21227, #49514, .T. ) ;
#48247=CARTESIAN_POINT ( 'NONE',  ( 2.980315163536433332, -78.44898908488615064, 8.777200079706965141 ) ) ;
#48252=CARTESIAN_POINT ( 'NONE',  ( -4.659120039122103485, -79.68376931176990752, -8.083663002107071449 ) ) ;
#48253=CARTESIAN_POINT ( 'NONE',  ( 8.796335266379964324, -80.00208333333898736, 6.760013919724087827 ) ) ;
#48255=LINE ( 'NONE', #15785, #37623 ) ;
#48256=EDGE_CURVE ( 'NONE', #47291, #27444, #4033, .T. ) ;
#48258=DIRECTION ( 'NONE',  ( -0.3090169943750105119, 0.000000000000000000, -0.9510565162951329921 ) ) ;
#48262=CARTESIAN_POINT ( 'NONE',  ( 8.365650024713001898, -79.80890222813398793, 4.340751507912000484 ) ) ;
#48264=CARTESIAN_POINT ( 'NONE',  ( 5.766697267524079962, -77.26874999999996874, -9.406996941509154553 ) ) ;
#48268=CARTESIAN_POINT ( 'NONE',  ( 6.760013919724077169, -77.37708333333333144, -8.796335266379971429 ) ) ;
#48269=CARTESIAN_POINT ( 'NONE',  ( -2.946080165379000082, -77.91047479902398720, -10.65686345704000004 ) ) ;
#48274=CARTESIAN_POINT ( 'NONE',  ( -9.467475792354999697, -77.19315246464168467, 1.978357023055999919 ) ) ;
#48276=CARTESIAN_POINT ( 'NONE',  ( -2.879226727952121756, -77.49583333333333712, 10.71369944335146407 ) ) ;
#48284=ORIENTED_EDGE ( 'NONE', *, *, #11379, .T. ) ;
#48294=CARTESIAN_POINT ( 'NONE',  ( -2.421167930323333106, -79.60416666666665719, -9.009247259181917045 ) ) ;
#48304=CARTESIAN_POINT ( 'NONE',  ( 2.879226727952050258, -78.55416666666667425, 10.71369944335148361 ) ) ;
#48305=B_SPLINE_CURVE_WITH_KNOTS ( 'NONE', 3,
 ( #8353, #44370, #16647, #8067, #16361, #3356, #8649, #21924, #2782, #53230, #34631, #11931, #48247, #26635, #39367, #52659, #57374, #52377, #29908, #25493 ),
 .UNSPECIFIED., .F., .F.,
 ( 4, 2, 2, 2, 2, 2, 2, 2, 2, 4 ),
 ( 0.000000000000000000, 0.1250000000000000555, 0.2500000000000000555, 0.3750000000000001665, 0.5000000000000002220, 0.5625000000000002220, 0.6250000000000002220, 0.7500000000000002220, 0.8750000000000001110, 1.000000000000000000 ),
 .UNSPECIFIED. ) ;
#48310=CARTESIAN_POINT ( 'NONE',  ( -10.29238134969365959, -80.12908025125918243, -3.880928803044727982 ) ) ;
#48324=CARTESIAN_POINT ( 'NONE',  ( 6.760013919724077169, -79.87708333333333144, -8.796335266379971429 ) ) ;
#48329=CARTESIAN_POINT ( 'NONE',  ( -9.497662397991334160, -77.28501590207432059, -0.2008463566140032963 ) ) ;
#48330=CARTESIAN_POINT ( 'NONE',  ( 4.999999999872000167, -80.49999999987198862, -4.857398774947999725E-10 ) ) ;
#48333=CARTESIAN_POINT ( 'NONE',  ( 8.875952806245999582, -79.23328771936498072, 3.056903470501999731 ) ) ;
#48337=ADVANCED_FACE ( 'NONE', ( #19918 ), #21277, .F. ) ;
#48343=CARTESIAN_POINT ( 'NONE',  ( 6.064331118019999245, -78.54256869612397907, -9.105586440592000841 ) ) ;
#48345=CARTESIAN_POINT ( 'NONE',  ( -10.46536824075000105, -80.40014086983299535, -4.041474877054999304 ) ) ;
#48355=DIRECTION ( 'NONE',  ( -1.000000000000000000, 0.000000000000000000, 0.000000000000000000 ) ) ;
#48367=CARTESIAN_POINT ( 'NONE',  ( 8.548480318118429011, -78.81895703212624937, -3.533306059048998637 ) ) ;
#48373=CARTESIAN_POINT ( 'NONE',  ( 2.879226727952049814, -77.95416666666666572, 10.71369944335148183 ) ) ;
#48375=CARTESIAN_POINT ( 'NONE',  ( 8.018769647075153273, -79.91052682219850567, 7.624166446277077291 ) ) ;
#48376=DIRECTION ( 'NONE',  ( -3.342748300494999961E-11, -1.000000000000000000, -3.127658994406000054E-09 ) ) ;
#48380=CARTESIAN_POINT ( 'NONE',  ( 5.326985168515999902, -77.34776426251399073, 7.723193303612999827 ) ) ;
#48395=CARTESIAN_POINT ( 'NONE',  ( -7.645247686219181382, -79.19858867851458228, 5.772722378017828504 ) ) ;
#48399=CARTESIAN_POINT ( 'NONE',  ( -1.303463199981000020, -80.09257338644599145, 9.693416794543999515 ) ) ;
#48407=AXIS2_PLACEMENT_3D ( 'NONE', #48975, #3800, #35073 ) ;
#48411=CARTESIAN_POINT ( 'NONE',  ( 10.52161952788999955, -77.15335001815408589, -3.541364337751999880 ) ) ;
#48417=CARTESIAN_POINT ( 'NONE',  ( 1.841371367509999857, -79.84963815277498611, -9.592189096167999196 ) ) ;
#48431=CARTESIAN_POINT ( 'NONE',  ( 1.441608637993120112, -79.96304127600662071, 9.136664121622990464 ) ) ;
#48435=CARTESIAN_POINT ( 'NONE',  ( 5.473581026676259675, -77.27553049482349934, -7.456605559097626568 ) ) ;
#48445=CARTESIAN_POINT ( 'NONE',  ( 0.2656919276500000482, -79.68383300265197988, -11.15441650005999996 ) ) ;
#48449=ADVANCED_FACE ( 'NONE', ( #23026 ), #47451, .F. ) ;
#48469=CARTESIAN_POINT ( 'NONE',  ( -4.399243655502999673, -79.77766721275199302, 10.05537673064999815 ) ) ;
#48476=CARTESIAN_POINT ( 'NONE',  ( -2.164532541486328565, -77.39366991027993947, 9.022216075546257485 ) ) ;
#48479=VECTOR ( 'NONE', #21738, 1000.000000000000000 ) ;
#48480=CARTESIAN_POINT ( 'NONE',  ( -2.977158780993999887, -78.63955604921899578, 10.75305190397999944 ) ) ;
#48487=CARTESIAN_POINT ( 'NONE',  ( 10.75000000000000000, -77.19999999999998863, -6.141891925717000695E-13 ) ) ;
#48490=( LENGTH_UNIT ( ) NAMED_UNIT ( * ) SI_UNIT ( .MILLI., .METRE. ) );
#48496=CARTESIAN_POINT ( 'NONE',  ( -6.961488625003511288, -79.69021735228992043, 6.501630528635893747 ) ) ;
#48502=VECTOR ( 'NONE', #24547, 1000.000000000000000 ) ;
#48505=CARTESIAN_POINT ( 'NONE',  ( -7.498854895474774906, -77.55022293857352622, 5.415685297931227993 ) ) ;
#48506=CARTESIAN_POINT ( 'NONE',  ( 6.393001003723999709, -77.19570245782817608, 9.000752526674000720 ) ) ;
#48507=CARTESIAN_POINT ( 'NONE',  ( 9.045658679128999680, -79.10650131180899791, 3.115350657311999782 ) ) ;
#48511=CARTESIAN_POINT ( 'NONE',  ( 11.10498291493000167, -80.10684763845199541, -1.830582403018000015 ) ) ;
#48516=EDGE_CURVE ( 'NONE', #24529, #49672, #7804, .T. ) ;
#48517=ORIENTED_EDGE ( 'NONE', *, *, #32159, .T. ) ;
#48536=CARTESIAN_POINT ( 'NONE',  ( 0.2539499232592060118, -78.07730306633010287, -10.83454063274043300 ) ) ;
#48537=CARTESIAN_POINT ( 'NONE',  ( 9.350230382969998644, -79.19953686653599334, -0.8778377520234000864 ) ) ;
#48539=CARTESIAN_POINT ( 'NONE',  ( 8.925548456419079457, -77.29999999999999716, -6.486984937931281614 ) ) ;
#48541=CARTESIAN_POINT ( 'NONE',  ( 0.000000000000000000, -74.64999999999999147, 0.000000000000000000 ) ) ;
#48544=CARTESIAN_POINT ( 'NONE',  ( -5.539808784079887083, -77.28333333333333144, -9.611650271896841957 ) ) ;
#48552=CARTESIAN_POINT ( 'NONE',  ( -6.294203684166999935, -77.20123665637598265, 7.343715272572999275 ) ) ;
#48558=ORIENTED_EDGE ( 'NONE', *, *, #29345, .T. ) ;
#48591=CARTESIAN_POINT ( 'NONE',  ( -9.236754519813018760, -78.60432763383623467, -0.5006253770964849137 ) ) ;
#48608=CARTESIAN_POINT ( 'NONE',  ( 10.31626776183999894, -78.03182302711998375, -3.746764721243999841 ) ) ;
#48610=CARTESIAN_POINT ( 'NONE',  ( 0.000000000000000000, -80.99999999999998579, -7.000000000000000000 ) ) ;
#48614=CARTESIAN_POINT ( 'NONE',  ( -9.326075088887810338, -79.75741750814056275, 5.512176992475737336 ) ) ;
#48617=CARTESIAN_POINT ( 'NONE',  ( 8.177883213696999221, -78.09878108138998698, -5.086790354254000057 ) ) ;
#48622=DIRECTION ( 'NONE',  ( 0.000000000000000000, 1.000000000000000000, 0.000000000000000000 ) ) ;
#48623=CARTESIAN_POINT ( 'NONE',  ( 7.307999405654648228, -78.90319446237640477, 5.704134542545350683 ) ) ;
#48628=CARTESIAN_POINT ( 'NONE',  ( -0.6558374186847000242, -79.68666419164598835, 11.02940581592999969 ) ) ;
#48630=CARTESIAN_POINT ( 'NONE',  ( -8.889114177306000286, -80.18886705758899325, 7.203513103890000657 ) ) ;
#48632=B_SPLINE_CURVE_WITH_KNOTS ( 'NONE', 3,
 ( #23715, #18133, #40855, #18426, #36128, #41726, #50018, #54144, #36416, #31682, #49728, #9271, #27549, #45592, #23136, #734, #18714, #33849, #19711, #37122, #19128, #33268, #46598, #6125, #42446, #1141, #55432, #55134, #14679, #24131, #29133, #42149, #37995, #20294, #28550, #1719, #10271, #15863, #9983, #38286, #15275, #2014, #6417, #2297, #37709, #55731, #56309, #56020, #32677, #15569, #33563, #51309, #28252, #10868, #27963, #28839, #46888, #1431, #11160, #24430, #47180, #20012, #46306, #51601, #37411 ),
 .UNSPECIFIED., .F., .F.,
 ( 4, 1, 1, 1, 1, 1, 1, 1, 1, 1, 1, 1, 1, 1, 1, 1, 1, 1, 1, 1, 1, 1, 1, 1, 1, 1, 1, 1, 1, 1, 1, 1, 1, 1, 1, 1, 1, 1, 1, 1, 1, 1, 1, 1, 1, 1, 1, 1, 1, 1, 1, 1, 1, 1, 1, 1, 1, 1, 1, 1, 1, 1, 4 ),
 ( 0.000000000000000000, 0.01249974716340015654, 0.02874975559081316412, 0.04499976401822616823, 0.06124977244563917234, 0.07749978087305219032, 0.09374978930046519443, 0.1099997977278781985, 0.1262498061552911888, 0.1424998145827041929, 0.1587498230101172247, 0.1749998314375302011, 0.1912498398649432330, 0.2074998482923562093, 0.2237498567197692412, 0.2399998651471822453, 0.2562498735745952216, 0.2724998820020082535, 0.2887498904294212854, 0.3049998988568342617, 0.3212499072842472381, 0.3374999157116603254, 0.3537499241390733018, 0.3699999325664862782, 0.3862499409938993100, 0.4024999494213123419, 0.4187499578487253182, 0.4349999662761383501, 0.4512499747035513264, 0.4674999831309643583, 0.4837499915583773902, 0.4999999999857903665, 0.5162500084132033429, 0.5325000168406163192, 0.5487500252680292956, 0.5650000336954423830, 0.5812500421228554703, 0.5975000505502684467, 0.6137500589776814230, 0.6300000674050943994, 0.6462500758325073758, 0.6625000842599203521, 0.6787500926873334395, 0.6950001011147464158, 0.7112501095421595032, 0.7275001179695724796, 0.7437501263969854559, 0.7600001348243984323, 0.7762501432518115196, 0.7925001516792244960, 0.8087501601066374723, 0.8250001685340504487, 0.8412501769614635361, 0.8575001853888765124, 0.8737501938162895998, 0.8900002022437025762, 0.9062502106711155525, 0.9225002190985285289, 0.9387502275259415052, 0.9550002359533544816, 0.9712502443807674579, 0.9875002528081806563, 1.000000000000000000 ),
 .UNSPECIFIED. ) ;
#48651=CARTESIAN_POINT ( 'NONE',  ( 9.238076819936575035, -78.84538428185697967, -0.5563267852515336731 ) ) ;
#48652=DIRECTION ( 'NONE',  ( 1.000000000000000000, 0.000000000000000000, 0.000000000000000000 ) ) ;
#48659=CARTESIAN_POINT ( 'NONE',  ( -9.469606800734000629, -80.05752053325198858, 5.597012331546999953 ) ) ;
#48663=CARTESIAN_POINT ( 'NONE',  ( -0.4913431507998999859, -77.39998299644997815, 9.369261706097999465 ) ) ;
#48664=DIRECTION ( 'NONE',  ( 0.000000000000000000, -1.000000000000000000, 0.000000000000000000 ) ) ;
#48678=CARTESIAN_POINT ( 'NONE',  ( 1.012474343122873544, -79.38347396807189682, -9.467961831871633649 ) ) ;
#48679=CARTESIAN_POINT ( 'NONE',  ( 9.468749999988999022, -76.98125000001098783, 2.084568677130999610E-09 ) ) ;
#48680=CARTESIAN_POINT ( 'NONE',  ( -2.879226727952121756, -78.99583333333333712, 10.71369944335146407 ) ) ;
#48682=CARTESIAN_POINT ( 'NONE',  ( 4.335968019780999327, -79.86848743689799335, -8.767120549026998333 ) ) ;
#48688=FACE_OUTER_BOUND ( 'NONE', #1313, .T. ) ;
#48694=CARTESIAN_POINT ( 'NONE',  ( -1.514723870011999818, -77.04329589215798535, -10.99769645839000098 ) ) ;
#48701=CARTESIAN_POINT ( 'NONE',  ( 3.366547962069000199, -79.42285120457597714, -9.168809063548000182 ) ) ;
#48718=CARTESIAN_POINT ( 'NONE',  ( 4.044174147134872221, -79.93931354737067352, 8.336790591702616382 ) ) ;
#48721=ORIENTED_EDGE ( 'NONE', *, *, #31004, .T. ) ;
#48722=CARTESIAN_POINT ( 'NONE',  ( 2.863093780795163745, -77.25021378612967737, -8.795631279814358550 ) ) ;
#48724=VECTOR ( 'NONE', #51254, 1000.000000000000000 ) ;
#48728=CARTESIAN_POINT ( 'NONE',  ( 0.000000000000000000, -80.74999999986198418, 0.000000000000000000 ) ) ;
#48731=CARTESIAN_POINT ( 'NONE',  ( -1.319038368507000181, -78.67250824667499387, -11.07933831235000177 ) ) ;
#48735=B_SPLINE_CURVE_WITH_KNOTS ( 'NONE', 3,
 ( #43677, #20373, #38367, #2941, #56389, #15939, #20658, #33927, #11523, #29500, #56676, #38942, #47835, #16520, #34501, #13827, #31825, #36266 ),
 .UNSPECIFIED., .F., .F.,
 ( 4, 2, 2, 2, 2, 2, 2, 2, 4 ),
 ( 0.000000000000000000, 0.1250000000000000000, 0.2500000000000000000, 0.3750000000000000000, 0.5000000000000000000, 0.6250000000000000000, 0.7500000000000000000, 0.8750000000000000000, 1.000000000000000000 ),
 .UNSPECIFIED. ) ;
#48754=CARTESIAN_POINT ( 'NONE',  ( 2.550499813263000348, -78.57381419345199447, -10.67515654612000020 ) ) ;
#48766=CARTESIAN_POINT ( 'NONE',  ( 11.04877620194000087, -78.05730764035098446, 0.05135089858452999978 ) ) ;
#48773=CARTESIAN_POINT ( 'NONE',  ( 7.137508353459040222, -79.51917351108399146, 8.454853940648140664 ) ) ;
#48780=ORIENTED_EDGE ( 'NONE', *, *, #12574, .T. ) ;
#48781=CARTESIAN_POINT ( 'NONE',  ( 1.102440175093327257, -79.61576928092233629, 9.466448183039451791 ) ) ;
#48786=CARTESIAN_POINT ( 'NONE',  ( -5.137220513087188856, -78.17816639323106642, -7.692279124526338663 ) ) ;
#48790=CARTESIAN_POINT ( 'NONE',  ( -4.333990198683386197, -77.51391215394883716, 8.171957043909507945 ) ) ;
#48791=CARTESIAN_POINT ( 'NONE',  ( -4.789974786805000662, -77.89883254012598002, -9.946872946892002076 ) ) ;
#48793=CARTESIAN_POINT ( 'NONE',  ( 9.583411031200000707, -78.15302099854598339, 1.526087275887999972 ) ) ;
#48797=CARTESIAN_POINT ( 'NONE',  ( -1.870137171474999915, -80.10216999377799141, -11.09839649295000008 ) ) ;
#48801=CARTESIAN_POINT ( 'NONE',  ( 8.082524092276891281, -78.70833333333332860, -4.658475568430806568 ) ) ;
#48811=AXIS2_PLACEMENT_3D ( 'NONE', #35668, #35075, #8822 ) ;
#48813=CARTESIAN_POINT ( 'NONE',  ( -10.82681686033000013, -80.56778745972700051, -1.485342682486999966 ) ) ;
#48826=CARTESIAN_POINT ( 'NONE',  ( 2.574080585026614187, -77.24375000000003411, -10.72942207085831079 ) ) ;
#48831=CARTESIAN_POINT ( 'NONE',  ( 9.499157866768639380, -79.10080562451891240, 0.1004279358040388037 ) ) ;
#48837=CARTESIAN_POINT ( 'NONE',  ( 5.212684961665999595, -77.06074883803579212, -8.147089634514999901 ) ) ;
#48863=DIRECTION ( 'NONE',  ( 0.7071067811865474617, 0.7071067811865474617, -1.168837077090079199E-09 ) ) ;
#48873=CARTESIAN_POINT ( 'NONE',  ( 0.000000000000000000, -81.99999999999998579, 0.000000000000000000 ) ) ;
#48877=CARTESIAN_POINT ( 'NONE',  ( -9.102064877486805372, -78.61442264338772645, -1.647833208901029689 ) ) ;
#48890=VERTEX_POINT ( 'NONE', #7691 ) ;
#48893=CARTESIAN_POINT ( 'NONE',  ( -11.00000000000000000, -79.19999999999998863, 0.000000000000000000 ) ) ;
#48902=CARTESIAN_POINT ( 'NONE',  ( -9.397814129314344456, -79.70741671815727614, 5.554578354712478294 ) ) ;
#48905=CARTESIAN_POINT ( 'NONE',  ( 5.254748191175000471, -79.19294275334198119, -7.810174947890000219 ) ) ;
#48915=CARTESIAN_POINT ( 'NONE',  ( 2.542269563431000190, -78.51447634179098145, -10.64070870773999822 ) ) ;
#48918=CARTESIAN_POINT ( 'NONE',  ( -10.62639753186000036, -79.83513114498597929, -3.930700632546999529 ) ) ;
#48921=ORIENTED_EDGE ( 'NONE', *, *, #46836, .T. ) ;
#48925=VERTEX_POINT ( 'NONE', #24834 ) ;
#48937=CARTESIAN_POINT ( 'NONE',  ( 9.086237931134723667, -78.83508176315426397, -1.732778305792737283 ) ) ;
#48942=CARTESIAN_POINT ( 'NONE',  ( -2.879226727952121756, -77.99583333333333712, 10.71369944335146407 ) ) ;
#48961=ORIENTED_EDGE ( 'NONE', *, *, #21888, .T. ) ;
#48969=AXIS2_PLACEMENT_3D ( 'NONE', #48610, #47475, #25290 ) ;
#48971=CARTESIAN_POINT ( 'NONE',  ( -6.912870113367000080, -79.64440148735099001, 6.919194171953000350 ) ) ;
#48975=CARTESIAN_POINT ( 'NONE',  ( 0.000000000000000000, -79.99999999999998579, 0.000000000000000000 ) ) ;
#48988=CARTESIAN_POINT ( 'NONE',  ( 8.249323304235000265, -80.03518932063198577, -5.229696851825000437 ) ) ;
#49004=CARTESIAN_POINT ( 'NONE',  ( -8.128721809369904960, -80.39067905721536533, 7.570748975258281277 ) ) ;
#49006=CARTESIAN_POINT ( 'NONE',  ( 6.895942029498000281, -79.29823107411199601, -8.909260232556000858 ) ) ;
#49007=CARTESIAN_POINT ( 'NONE',  ( 2.096143898794329274, -77.24324615902062874, -9.044846050601076826 ) ) ;
#49009=AXIS2_PLACEMENT_3D ( 'NONE', #56758, #2740, #52332 ) ;
#49016=CARTESIAN_POINT ( 'NONE',  ( 11.15746894976000014, -78.30730764035098446, 0.05185606496389000286 ) ) ;
#49033=CARTESIAN_POINT ( 'NONE',  ( 9.521438313890000060, -77.39399981532699258, 0.1121992162086000028 ) ) ;
#49043=AXIS2_PLACEMENT_3D ( 'NONE', #7911, #43649, #3208 ) ;
#49044=CARTESIAN_POINT ( 'NONE',  ( -8.058638732054999920, -78.48953713045399638, -7.451332657186999775 ) ) ;
#49054=CARTESIAN_POINT ( 'NONE',  ( 6.829411927397999627, -78.92047959254598766, -8.823306204757001225 ) ) ;
#49056=DIRECTION ( 'NONE',  ( -1.000000000000000000, 0.000000000000000000, 0.000000000000000000 ) ) ;
#49078=EDGE_LOOP ( 'NONE', ( #21180, #25949, #25304, #43140 ) ) ;
#49079=CARTESIAN_POINT ( 'NONE',  ( 2.855190675867043115, -77.45020626835986377, 8.798204014871961576 ) ) ;
#49080=CARTESIAN_POINT ( 'NONE',  ( -10.84202097104999929, -77.29444807548399865, 2.082001701158999740 ) ) ;
#49081=CARTESIAN_POINT ( 'NONE',  ( -9.702231720816998362, -78.89204055589898701, -0.1934140619087000024 ) ) ;
#49086=CARTESIAN_POINT ( 'NONE',  ( 0.000000000000000000, -81.79999999999998295, 0.000000000000000000 ) ) ;
#49089=DIRECTION ( 'NONE',  ( 0.000000000000000000, 1.000000000000000000, 0.000000000000000000 ) ) ;
#49113=CARTESIAN_POINT ( 'NONE',  ( -8.960380918909999437, -79.54589830381199533, -2.921951021776999724 ) ) ;
#49125=CARTESIAN_POINT ( 'NONE',  ( -9.555818165766000405, -77.39146748629899264, -0.1257991660602000017 ) ) ;
#49129=DIRECTION ( 'NONE',  ( 0.000000000000000000, -1.000000000000000000, 0.000000000000000000 ) ) ;
#49132=CARTESIAN_POINT ( 'NONE',  ( 11.00000000000000000, -79.34999999999999432, -1.064824513673000067E-14 ) ) ;
#49138=VECTOR ( 'NONE', #18371, 1000.000000000000000 ) ;
#49139=ORIENTED_EDGE ( 'NONE', *, *, #47082, .F. ) ;
#49141=ORIENTED_EDGE ( 'NONE', *, *, #27294, .T. ) ;
#49158=CARTESIAN_POINT ( 'NONE',  ( 8.240135455977000589, -77.91526456327599703, -5.125512367919999868 ) ) ;
#49174=VERTEX_POINT ( 'NONE', #28232 ) ;
#49183=CIRCLE ( 'NONE', #9619, 4.100000000000000533 ) ;
#49191=CARTESIAN_POINT ( 'NONE',  ( -8.968424590936999508, -77.43311187452998468, 2.773906523901999766 ) ) ;
#49196=ORIENTED_EDGE ( 'NONE', *, *, #50332, .F. ) ;
#49199=ADVANCED_FACE ( 'NONE', ( #50708 ), #1696, .F. ) ;
#49203=CARTESIAN_POINT ( 'NONE',  ( -10.66249531825000041, -79.86290934975998823, 1.062579819291000094 ) ) ;
#49230=CARTESIAN_POINT ( 'NONE',  ( 9.249824806346651940, -77.84496366503705644, -0.6054522768334679172 ) ) ;
#49235=CARTESIAN_POINT ( 'NONE',  ( 9.250000000000000000, -79.84999999999999432, 0.000000000000000000 ) ) ;
#49260=CARTESIAN_POINT ( 'NONE',  ( -9.737659524074000927, -78.83077255621898871, -0.1941203154314999901 ) ) ;
#49262=DIRECTION ( 'NONE',  ( 0.000000000000000000, 1.000000000000000000, 0.000000000000000000 ) ) ;
#49269=EDGE_CURVE ( 'NONE', #45083, #54465, #50334, .T. ) ;
#49276=CARTESIAN_POINT ( 'NONE',  ( -4.598873869541999504, -77.52019710480799120, -10.10425737566999871 ) ) ;
#49284=CARTESIAN_POINT ( 'NONE',  ( -0.6514213267380000172, -79.65015981238198606, 9.745581310452999801 ) ) ;
#49292=CARTESIAN_POINT ( 'NONE',  ( 7.406085232244485894, -77.54399565168795050, -6.270863524971103331 ) ) ;
#49300=CARTESIAN_POINT ( 'NONE',  ( 8.864563766897090247, -79.87323291346528720, 2.649389835334180709 ) ) ;
#49303=CARTESIAN_POINT ( 'NONE',  ( -10.98029981754000062, -80.11290934975998823, 1.094250890400999987 ) ) ;
#49304=CARTESIAN_POINT ( 'NONE',  ( 1.379774402751460238, -77.23701117038012853, -9.169337788885616902 ) ) ;
#49306=AXIS2_PLACEMENT_3D ( 'NONE', #29478, #2074, #2921 ) ;
#49310=CARTESIAN_POINT ( 'NONE',  ( -9.358624512280380614, -80.44999999999998863, -5.407950800341189357 ) ) ;
#49311=CARTESIAN_POINT ( 'NONE',  ( 9.791822688510999129, -79.34672475065998754, 5.349000663092000174 ) ) ;
#49317=B_SPLINE_SURFACE_WITH_KNOTS ( 'NONE', 3, 3, ( 
 ( #37870, #1585, #5411, #14844, #33436, #55297, #32838, #37282, #1297, #55890, #51472, #5131, #728, #19574, #18708, #50596, #32256, #41431, #18998, #36990, #55006, #32546, #33726, #52618, #43472, #29012, #52333, #11604, #43188, #47342, #3029, #21025, #11029, #42895, #20458, #6579, #47921, #34012, #39031, #6869, #24592, #47051, #38158, #57043, #52047, #24879, #21310, #16602, #48206, #16023, #29292, #34589, #12170, #38451, #29579, #42606, #2169, #20170, #56181, #7453, #34301, #15729, #30156, #25452, #2454, #7739, #56468 ),
 ( #25737, #57328, #39320, #47636, #2741, #7160, #25164, #11889, #20741, #38740, #43765, #3315, #16891, #34873, #51761, #11312, #56760, #16318, #29867, #4179, #40777, #53779, #4766, #58197, #36049, #22766, #48480, #27178, #39604, #12735, #22175, #26589, #44623, #53189, #17760, #31017, #49054, #26892, #44047, #39888, #3594, #21600, #8602, #13611, #26018, #369, #40184, #8312, #13018, #30730, #18350, #52903, #35747, #13313, #17169, #57609, #31308, #57904, #21881, #53477, #12452, #17458, #8899, #35446, #49351, #44916, #4473 ),
 ( #30447, #22473, #35154, #48766, #8023, #45217, #40484, #31606, #26311, #79, #18057, #44325, #3881, #54072, #49647, #9195, #2031, #11464, #32188, #33866, #51623, #55751, #23056, #20031, #50231, #15881, #19733, #6731, #45513, #41071, #38017, #54366, #15296, #56040, #9777, #36340, #15588, #51906, #7019, #658, #25021, #43042, #13905, #2603, #33289, #10886, #27767, #31900, #49942, #5059, #45809, #5343, #18644, #36634, #28861, #24154, #16461, #16173, #17316, #26452, #56905, #48628, #3178, #25596, #53332, #56614, #39749 ),
 ( #43909, #16751, #34731, #12598, #11746, #43616, #29725, #47776, #52759, #57759, #52190, #44475, #12314, #34442, #39172, #20881, #20600, #48915, #48343, #7881, #43327, #25308, #30302, #21168, #48066, #25883, #34151, #3455, #30596, #21461, #39468, #57472, #17033, #8175, #26177, #52475, #44195, #2885, #3742, #21745, #12880, #35303, #38885, #12033, #30011, #17614, #26745, #9640, #522, #50095, #13167, #49505, #31165, #32051, #58054, #45078, #36780, #23210, #40934, #58352, #235, #27626, #27337, #4025, #45668, #22030, #49203 ) ),
 .UNSPECIFIED., .F., .F., .F.,
 ( 4, 4 ),
 ( 4, 1, 1, 1, 1, 1, 1, 1, 1, 1, 1, 1, 1, 1, 1, 1, 1, 1, 1, 1, 1, 1, 1, 1, 1, 1, 1, 1, 1, 1, 1, 1, 1, 1, 1, 1, 1, 1, 1, 1, 1, 1, 1, 1, 1, 1, 1, 1, 1, 1, 1, 1, 1, 1, 1, 1, 1, 1, 1, 1, 1, 1, 1, 1, 4 ),
 ( -0.1387574078320999993, 1.138757407831999968 ),
 ( -0.02000000000000000042, -0.003749999999999999861, 0.01250000000000000069, 0.02875000000000000125, 0.04499999999999999833, 0.06124999999999999889, 0.07749999999999999944, 0.09375000000000000000, 0.1100000000000000006, 0.1262500000000000011, 0.1424999999999999878, 0.1587500000000000022, 0.1749999999999999889, 0.1912500000000000033, 0.2074999999999999900, 0.2237500000000000044, 0.2399999999999999911, 0.2562499999999999778, 0.2725000000000000200, 0.2887500000000000067, 0.3049999999999999933, 0.3212499999999999800, 0.3375000000000000222, 0.3537500000000000089, 0.3699999999999999956, 0.3862499999999999822, 0.4025000000000000244, 0.4187500000000000111, 0.4349999999999999978, 0.4512499999999999845, 0.4675000000000000266, 0.4837500000000000133, 0.5000000000000000000, 0.5162499999999999867, 0.5324999999999999734, 0.5487499999999999600, 0.5649999999999999467, 0.5812500000000000444, 0.5975000000000000311, 0.6137500000000000178, 0.6300000000000000044, 0.6462499999999999911, 0.6624999999999999778, 0.6787499999999999645, 0.6949999999999999512, 0.7112500000000000488, 0.7275000000000000355, 0.7437500000000000222, 0.7600000000000000089, 0.7762499999999999956, 0.7924999999999999822, 0.8087499999999999689, 0.8249999999999999556, 0.8412500000000000533, 0.8575000000000000400, 0.8737500000000000266, 0.8900000000000000133, 0.9062500000000000000, 0.9224999999999999867, 0.9387499999999999734, 0.9549999999999999600, 0.9712499999999999467, 0.9875000000000000444, 1.003749999999999920, 1.020000000000000018 ),
 .UNSPECIFIED. ) ;
#49329=CARTESIAN_POINT ( 'NONE',  ( 7.120006596302999924, -77.45084747358500010, 6.322648361264000094 ) ) ;
#49340=CARTESIAN_POINT ( 'NONE',  ( 10.87588596538000019, -79.66941601242598381, -1.476184626237000197 ) ) ;
#49341=CARTESIAN_POINT ( 'NONE',  ( -8.796335266379985640, -79.15208333333333712, -6.760013919724054965 ) ) ;
#49347=CARTESIAN_POINT ( 'NONE',  ( 9.021848782386655330, -77.26870337215281381, 2.167559314716497987 ) ) ;
#49351=CARTESIAN_POINT ( 'NONE',  ( -10.03539896543000154, -79.70706551386098226, 4.876675511606999969 ) ) ;
#49354=CARTESIAN_POINT ( 'NONE',  ( 9.549999999999998934, -79.99999999999998579, 0.000000000000000000 ) ) ;
#49356=LINE ( 'NONE', #57335, #14151 ) ;
#49365=CARTESIAN_POINT ( 'NONE',  ( 9.499549289235639904, -79.50042064254546403, 0.05021470316550929319 ) ) ;
#49373=CARTESIAN_POINT ( 'NONE',  ( -6.539788562102244462, -78.16268306815329936, -6.541533809854823467 ) ) ;
#49379=CARTESIAN_POINT ( 'NONE',  ( 1.180810718627301803, -77.46484884203415788, 9.175185427096824498 ) ) ;
#49380=CARTESIAN_POINT ( 'NONE',  ( 10.74764839381999870, -78.17848693479398037, -0.2248421733643000131 ) ) ;
#49382=CARTESIAN_POINT ( 'NONE',  ( -9.626984307556000431, -78.38041163157799929, 1.221426423741999834 ) ) ;
#49407=CARTESIAN_POINT ( 'NONE',  ( 1.439896632895284911, -80.06458333334573751, 11.00000000000000355 ) ) ;
#49417=DIRECTION ( 'NONE',  ( 0.000000000000000000, 1.000000000000000000, 0.000000000000000000 ) ) ;
#49421=CARTESIAN_POINT ( 'NONE',  ( 0.000000000000000000, -81.99999999999998579, -7.000000000000000000 ) ) ;
#49432=VERTEX_POINT ( 'NONE', #38481 ) ;
#49435=CARTESIAN_POINT ( 'NONE',  ( 1.439896632895317552, -79.46458333333332291, 11.00000000000000000 ) ) ;
#49447=CARTESIAN_POINT ( 'NONE',  ( 0.000000000000000000, -81.19999999999998863, 6.000000000000000000 ) ) ;
#49449=B_SPLINE_CURVE_WITH_KNOTS ( 'NONE', 3,
 ( #30289, #48329, #8160, #7868 ),
 .UNSPECIFIED., .F., .F.,
 ( 4, 4 ),
 ( 0.000000000000000000, 1.000000000000000000 ),
 .UNSPECIFIED. ) ;
#49455=CARTESIAN_POINT ( 'NONE',  ( -9.177034484502000211, -77.30309342897207614, 6.137278520473000043 ) ) ;
#49457=EDGE_CURVE ( 'NONE', #36425, #5025, #33936, .T. ) ;
#49460=DIRECTION ( 'NONE',  ( 1.000000000000000000, 0.000000000000000000, 0.000000000000000000 ) ) ;
#49463=CARTESIAN_POINT ( 'NONE',  ( 9.662203867310999783, -78.96694624104797811, 0.9012207007054000574 ) ) ;
#49494=CARTESIAN_POINT ( 'NONE',  ( -2.523869816676000077, -78.56059042997900121, -9.181528052588999955 ) ) ;
#49503=EDGE_LOOP ( 'NONE', ( #38358, #10099, #15459, #9938, #27269 ) ) ;
#49505=CARTESIAN_POINT ( 'NONE',  ( -3.536853559812999759, -79.46961638910198644, -10.35270415072999839 ) ) ;
#49514=LINE ( 'NONE', #4639, #27601 ) ;
#49522=CYLINDRICAL_SURFACE ( 'NONE', #170, 10.69999999999999929 ) ;
#49530=CARTESIAN_POINT ( 'NONE',  ( 0.06586989957135422347, -78.72571929582086625, -9.249708549591806772 ) ) ;
#49533=CARTESIAN_POINT ( 'NONE',  ( 6.760013919724039866, -78.42291666666669414, 8.796335266379998075 ) ) ;
#49548=CARTESIAN_POINT ( 'NONE',  ( 0.000000000000000000, -74.64999999999999147, 0.000000000000000000 ) ) ;
#49553=CARTESIAN_POINT ( 'NONE',  ( -9.146956334765604879, -78.14765838888041571, -6.250533269645468515 ) ) ;
#49554=DIRECTION ( 'NONE',  ( 0.000000000000000000, 0.000000000000000000, -1.000000000000000000 ) ) ;
#49556=LINE ( 'NONE', #45129, #23769 ) ;
#49563=CARTESIAN_POINT ( 'NONE',  ( -9.185039845617701815, -80.00000000000001421, -1.456806635703324915 ) ) ;
#49567=CARTESIAN_POINT ( 'NONE',  ( 9.725848778082999857, -78.57495809405799037, -0.5172632330995999839 ) ) ;
#49570=CARTESIAN_POINT ( 'NONE',  ( -3.399186938124999724, -77.19999999999998863, -10.46162167925000119 ) ) ;
#49582=CARTESIAN_POINT ( 'NONE',  ( 11.07931224411999871, -77.73081168025198906, -1.719192531530000068 ) ) ;
#49584=EDGE_LOOP ( 'NONE', ( #50733, #50623, #25177, #17179, #14795 ) ) ;
#49587=CARTESIAN_POINT ( 'NONE',  ( 9.202039358297998461, -80.03983171147699238, 2.360608321670000453 ) ) ;
#49600=CARTESIAN_POINT ( 'NONE',  ( -9.669247687117000112, -77.75675262319563785, -0.8224101967608998809 ) ) ;
#49602=CARTESIAN_POINT ( 'NONE',  ( 8.989019320876588282, -79.86904670615129476, 2.181506882885325904 ) ) ;
#49605=CARTESIAN_POINT ( 'NONE',  ( -9.512853590378179902, -77.34556464508717966, 0.5183098463306959891 ) ) ;
#49624=CARTESIAN_POINT ( 'NONE',  ( -8.000000000000000000, -81.99999999999998579, 0.000000000000000000 ) ) ;
#49631=ADVANCED_FACE ( 'NONE', ( #11725 ), #52899, .F. ) ;
#49632=CARTESIAN_POINT ( 'NONE',  ( 0.000000000000000000, -74.64999999999999147, 0.000000000000000000 ) ) ;
#49635=CARTESIAN_POINT ( 'NONE',  ( 0.2613587267741000475, -79.55704659509599708, -10.97249781033000104 ) ) ;
#49640=B_SPLINE_CURVE_WITH_KNOTS ( 'NONE', 3,
 ( #4645, #35618, #22646, #53644, #13185, #18230, #13775, #19977, #6384, #24098, #41525, #41818, #33233, #10533, #45683, #15241, #5223, #14356, #51278, #28515, #23802 ),
 .UNSPECIFIED., .F., .F.,
 ( 4, 2, 2, 2, 1, 2, 2, 2, 2, 2, 4 ),
 ( 0.000000000000000000, 0.1249999999999999167, 0.2499999999999998890, 0.3124999999999998335, 0.3749999999999998335, 0.4374999999999998890, 0.4999999999999998890, 0.6249999999999998890, 0.7499999999999998890, 0.8750000000000000000, 1.000000000000000000 ),
 .UNSPECIFIED. ) ;
#49644=CARTESIAN_POINT ( 'NONE',  ( 10.61050599188999932, -77.92876026662598576, -2.901234667509999809 ) ) ;
#49647=CARTESIAN_POINT ( 'NONE',  ( -8.112440615085001028, -78.36632353800997919, -7.501079983178001065 ) ) ;
#49652=CARTESIAN_POINT ( 'NONE',  ( -5.684557159767995138, -79.92708333333332860, 7.396918292183145560 ) ) ;
#49669=CARTESIAN_POINT ( 'NONE',  ( -5.126676588143355140, -78.17827689695096183, -7.699309493463673881 ) ) ;
#49672=VERTEX_POINT ( 'NONE', #16148 ) ;
#49675=CARTESIAN_POINT ( 'NONE',  ( 1.444433356061864737, -77.46253582747604582, 9.136518341544702437 ) ) ;
#49676=CARTESIAN_POINT ( 'NONE',  ( 6.393001003723999709, -77.31630830916999741, 9.000752526674000720 ) ) ;
#49678=CARTESIAN_POINT ( 'NONE',  ( 2.260091721765999928, -79.03415970154399872, -9.437303113984999214 ) ) ;
#49684=CARTESIAN_POINT ( 'NONE',  ( 10.52250585264000016, -78.65712618243998122, -2.994108701640999737 ) ) ;
#49698=CARTESIAN_POINT ( 'NONE',  ( 8.646554484075000602, -80.31431271246199799, -7.432130245983000094 ) ) ;
#49707=FACE_BOUND ( 'NONE', #29099, .T. ) ;
#49708=AXIS2_PLACEMENT_3D ( 'NONE', #21062, #47378, #20207 ) ;
#49711=CARTESIAN_POINT ( 'NONE',  ( -2.879226727952071574, -79.80416666666666003, -10.71369944335147473 ) ) ;
#49725=CARTESIAN_POINT ( 'NONE',  ( 9.208615812369000508, -77.10488338023777999, 2.957800710608999850 ) ) ;
#49728=CARTESIAN_POINT ( 'NONE',  ( -10.44304457033000055, -78.32510815631960099, 3.377400876517000050 ) ) ;
#49740=VERTEX_POINT ( 'NONE', #22896 ) ;
#49745=CARTESIAN_POINT ( 'NONE',  ( -9.914363537814757876, -79.81715790035769942, 4.347490629219784353 ) ) ;
#49759=CARTESIAN_POINT ( 'NONE',  ( 1.487026788147999934, -77.34678798069599281, -9.589549613196998834 ) ) ;
#49774=CARTESIAN_POINT ( 'NONE',  ( -3.399186938124999724, -77.19999999999998863, -10.46162167925000119 ) ) ;
#49775=EDGE_LOOP ( 'NONE', ( #43040, #41004, #4870, #55608 ) ) ;
#49776=CARTESIAN_POINT ( 'NONE',  ( 11.00000000000000711, -78.43958333333333144, -1.439896632895300010 ) ) ;
#49777=ADVANCED_FACE ( 'NONE', ( #498 ), #14031, .F. ) ;
#49780=CARTESIAN_POINT ( 'NONE',  ( -8.739412744344001283, -79.79261095533199466, 4.325800834547999685 ) ) ;
#49787=DIRECTION ( 'NONE',  ( 0.000000000000000000, -1.000000000000000000, 0.000000000000000000 ) ) ;
#49792=CARTESIAN_POINT ( 'NONE',  ( -1.518219907972000016, -78.90870446205198618, 9.290113175764000530 ) ) ;
#49816=ORIENTED_EDGE ( 'NONE', *, *, #46109, .F. ) ;
#49826=CARTESIAN_POINT ( 'NONE',  ( 8.209582066784916421, -78.81200429033071941, -4.264407347131307091 ) ) ;
#49829=CARTESIAN_POINT ( 'NONE',  ( -1.210856240595359790, -77.71471340245162196, -9.250524551649785820 ) ) ;
#49849=CARTESIAN_POINT ( 'NONE',  ( 10.42062934545543840, -77.22079869211786729, 2.728807196244066535 ) ) ;
#49850=CARTESIAN_POINT ( 'NONE',  ( 2.600000000000000089, -77.49999999999998579, 0.000000000000000000 ) ) ;
#49877=CARTESIAN_POINT ( 'NONE',  ( 6.923622142245000610, -78.17102818423599331, -8.818797536904998680 ) ) ;
#49881=CONICAL_SURFACE ( 'NONE', #51782, 4.899999999795999983, 0.7853981633972997312 ) ;
#49883=CARTESIAN_POINT ( 'NONE',  ( 1.739862777674999972, -79.13059728025397987, 9.611119481339999382 ) ) ;
#49894=CARTESIAN_POINT ( 'NONE',  ( 4.186942200393000135, -78.41050069316224835, -8.754440266352000677 ) ) ;
#49895=CARTESIAN_POINT ( 'NONE',  ( 8.197317322123611305, -79.88882380982184372, 4.285112605895506022 ) ) ;
#49922=CARTESIAN_POINT ( 'NONE',  ( 9.440269692223999698, -77.94108065130299678, -1.906441214165000009 ) ) ;
#49930=CARTESIAN_POINT ( 'NONE',  ( 0.2613587267741000475, -79.61734952076598404, -10.97249781033000104 ) ) ;
#49933=CARTESIAN_POINT ( 'NONE',  ( -10.99980394231345926, -80.10023817985064909, 1.711188753626703361E-06 ) ) ;
#49938=CARTESIAN_POINT ( 'NONE',  ( -8.571485855526580266, -77.46864983315596476, 3.552044476763973613 ) ) ;
#49942=CARTESIAN_POINT ( 'NONE',  ( -10.86532694299999946, -79.32146358532099839, -2.005633084294999868 ) ) ;
#49961=EDGE_CURVE ( 'NONE', #21244, #5115, #51648, .T. ) ;
#49969=ORIENTED_EDGE ( 'NONE', *, *, #6348, .F. ) ;
#49970=CARTESIAN_POINT ( 'NONE',  ( 2.734482912475208582, -77.45129537202082304, 8.836507949619202051 ) ) ;
#49971=CARTESIAN_POINT ( 'NONE',  ( -10.47078769031000078, -77.89551604846599275, -3.499536356729999742 ) ) ;
#49973=CARTESIAN_POINT ( 'NONE',  ( -8.592320330817999618, -78.35198780244898842, 4.510292750937000328 ) ) ;
#49978=CARTESIAN_POINT ( 'NONE',  ( -10.10513987668000091, -78.46047970211098743, -4.192131248929999998 ) ) ;
#49983=EDGE_LOOP ( 'NONE', ( #48154, #53772 ) ) ;
#49993=CARTESIAN_POINT ( 'NONE',  ( -7.233356275331999541, -78.52392489796099539, 6.024097567370000128 ) ) ;
#50015=CARTESIAN_POINT ( 'NONE',  ( -6.294203684166999935, -77.32184250771798872, 7.343715272572999275 ) ) ;
#50018=CARTESIAN_POINT ( 'NONE',  ( 1.684372618195999927, -78.21273873898907425, 10.84559388857000073 ) ) ;
#50033=CARTESIAN_POINT ( 'NONE',  ( -1.870137171474999915, -79.96171613058454852, -11.09839649295000008 ) ) ;
#50042=DIRECTION ( 'NONE',  ( 0.000000000000000000, 1.000000000000000000, 0.000000000000000000 ) ) ;
#50047=CARTESIAN_POINT ( 'NONE',  ( 9.259046916275000427, -78.48374114585499228, 2.905298533503999803 ) ) ;
#50070=DIRECTION ( 'NONE',  ( 0.000000000000000000, -1.000000000000000000, 0.000000000000000000 ) ) ;
#50073=CARTESIAN_POINT ( 'NONE',  ( 9.690945690674999113, -79.58805234752598778, 1.084186244826999879 ) ) ;
#50080=CARTESIAN_POINT ( 'NONE',  ( 7.408857453855000053, -77.49712623080398544, 8.497927402505000671 ) ) ;
#50084=CARTESIAN_POINT ( 'NONE',  ( -6.351606481687999128, -78.39004745520499284, 7.094185741421999758 ) ) ;
#50089=EDGE_LOOP ( 'NONE', ( #31772, #46844, #11502, #48284 ) ) ;
#50095=CARTESIAN_POINT ( 'NONE',  ( -9.408410525920000822, -79.41343168043698597, -5.582976599613999724 ) ) ;
#50103=EDGE_CURVE ( 'NONE', #10301, #43339, #28349, .T. ) ;
#50114=CARTESIAN_POINT ( 'NONE',  ( 0.000000000000000000, -81.79999999999998295, 0.000000000000000000 ) ) ;
#50118=CARTESIAN_POINT ( 'NONE',  ( -1.686463579793599399, -78.71046731272916475, -9.094966459575084983 ) ) ;
#50122=VECTOR ( 'NONE', #1833, 1000.000000000000114 ) ;
#50126=AXIS2_PLACEMENT_3D ( 'NONE', #7589, #2876, #44187 ) ;
#50143=DIRECTION ( 'NONE',  ( 0.7071067811865470176, -0.7071067811865470176, 3.680441518142245308E-08 ) ) ;
#50165=CARTESIAN_POINT ( 'NONE',  ( -6.086064908458999945, -77.85035948279599438, 9.284690194605000002 ) ) ;
#50169=VERTEX_POINT ( 'NONE', #40360 ) ;
#50172=CARTESIAN_POINT ( 'NONE',  ( -0.6514213267380000172, -79.89061850717349955, 9.745581310452999801 ) ) ;
#50183=CARTESIAN_POINT ( 'NONE',  ( 7.032282396509031308, -79.90637039191506119, 6.009017827964323821 ) ) ;
#50204=CARTESIAN_POINT ( 'NONE',  ( 1.492218263521933874, -76.94999999999998863, -9.411694429295081932 ) ) ;
#50206=CARTESIAN_POINT ( 'NONE',  ( 9.630178197611998669, -77.45787555610998254, 0.1134805908625000082 ) ) ;
#50216=CARTESIAN_POINT ( 'NONE',  ( 9.233664981878000333, -79.78590364676199442, 5.933249305785000871 ) ) ;
#50217=CARTESIAN_POINT ( 'NONE',  ( -11.00000000000000000, -79.09999999999999432, 0.000000000000000000 ) ) ;
#50221=CARTESIAN_POINT ( 'NONE',  ( 9.250000000000000000, -77.74999999999998579, 0.000000000000000000 ) ) ;
#50225=CARTESIAN_POINT ( 'NONE',  ( -8.824831950807848102, -77.47489816006239494, 2.865719031100893321 ) ) ;
#50231=CARTESIAN_POINT ( 'NONE',  ( 4.665505440478000310, -78.64724708133699949, 10.01553556391000122 ) ) ;
#50232=DIRECTION ( 'NONE',  ( 0.000000000000000000, 1.000000000000000000, 0.000000000000000000 ) ) ;
#50236=CARTESIAN_POINT ( 'NONE',  ( 9.304647597727065289, -79.15561160917410177, -5.821627946328172598 ) ) ;
#50238=ORIENTED_EDGE ( 'NONE', *, *, #1131, .F. ) ;
#50239=ORIENTED_EDGE ( 'NONE', *, *, #44488, .F. ) ;
#50257=CARTESIAN_POINT ( 'NONE',  ( 2.837648390166478407, -77.45036520058170026, 8.803880890672857618 ) ) ;
#50258=CARTESIAN_POINT ( 'NONE',  ( 8.680753609988000719, -77.73315101347900224, 6.821192461343000168 ) ) ;
#50260=CARTESIAN_POINT ( 'NONE',  ( -8.680270256945998852, -77.35715378293498645, 3.860428508128000313 ) ) ;
#50265=CARTESIAN_POINT ( 'NONE',  ( 7.117135278674999732, -80.31097582047098626, 8.718833803912000135 ) ) ;
#50267=CARTESIAN_POINT ( 'NONE',  ( -2.162167942093999873, -78.32001793044798887, 10.72440421974000024 ) ) ;
#50280=CARTESIAN_POINT ( 'NONE',  ( -5.190928442694000111, -77.50066704931698780, 7.852735600434000318 ) ) ;
#50286=PLANE ( 'NONE',  #53251 ) ;
#50289=CARTESIAN_POINT ( 'NONE',  ( 7.788493169598000421, -78.62176246810599878, 7.733265204867000087 ) ) ;
#50317=EDGE_LOOP ( 'NONE', ( #6530, #50650, #15229, #22300 ) ) ;
#50325=CARTESIAN_POINT ( 'NONE',  ( 4.312078000770541486, -78.26364788450446497, -8.189147600941369731 ) ) ;
#50332=EDGE_CURVE ( 'NONE', #48890, #21042, #5734, .T. ) ;
#50334=LINE ( 'NONE', #18740, #17275 ) ;
#50335=CARTESIAN_POINT ( 'NONE',  ( 8.444976262095000408, -78.00053605066298701, 4.780490068936999570 ) ) ;
#50353=CARTESIAN_POINT ( 'NONE',  ( 8.275552136666096459, -79.99999999999998579, -4.772006449322993227 ) ) ;
#50355=CARTESIAN_POINT ( 'NONE',  ( 10.65482429239385098, -77.19999999999998863, -1.623674524292790133 ) ) ;
#50357=CARTESIAN_POINT ( 'NONE',  ( 2.879226727952094222, -78.34583333333331723, -10.71369944335146940 ) ) ;
#50360=CARTESIAN_POINT ( 'NONE',  ( 2.064412114960999745, -79.47116171449498268, -9.530377264972001328 ) ) ;
#50363=DIRECTION ( 'NONE',  ( 0.000000000000000000, 1.000000000000000000, -4.137348672605999941E-14 ) ) ;
#50365=ORIENTED_EDGE ( 'NONE', *, *, #27540, .F. ) ;
#50367=DIRECTION ( 'NONE',  ( 0.000000000000000000, 0.000000000000000000, -1.000000000000000000 ) ) ;
#50368=CARTESIAN_POINT ( 'NONE',  ( 5.517529752410999855, -77.13936266505909600, 9.309542203537999328 ) ) ;
#50369=AXIS2_PLACEMENT_3D ( 'NONE', #29811, #2693, #48150 ) ;
#50373=CARTESIAN_POINT ( 'NONE',  ( 7.184025905720999639, -77.71490363863499340, -6.082841960620999799 ) ) ;
#50398=DIRECTION ( 'NONE',  ( 0.000000000000000000, 1.000000000000000000, 0.000000000000000000 ) ) ;
#50401=CARTESIAN_POINT ( 'NONE',  ( 7.658986946679876340, -78.65252498771793910, 5.959341133100068966 ) ) ;
#50403=DIRECTION ( 'NONE',  ( 0.000000000000000000, -1.000000000000000000, 0.000000000000000000 ) ) ;
#50409=CARTESIAN_POINT ( 'NONE',  ( -1.793454718549643445, -78.70954372627176099, -9.074418929172219705 ) ) ;
#50412=CARTESIAN_POINT ( 'NONE',  ( -9.331000443659689836, -80.14465528251990634, -5.825445497097998526 ) ) ;
#50424=CARTESIAN_POINT ( 'NONE',  ( 5.683913069336140822, -79.77753931263904974, -7.396130091655648719 ) ) ;
#50430=CARTESIAN_POINT ( 'NONE',  ( -7.722615280105806335, -77.38904062276650109, 7.510299681650742798 ) ) ;
#50431=DIRECTION ( 'NONE',  ( 0.000000000000000000, -1.000000000000000000, 0.000000000000000000 ) ) ;
#50439=CARTESIAN_POINT ( 'NONE',  ( 8.847929224218546551, -78.32657344890409945, -2.698424406155022659 ) ) ;
#50448=DIRECTION ( 'NONE',  ( 1.000000000000000000, 0.000000000000000000, 0.000000000000000000 ) ) ;
#50459=CARTESIAN_POINT ( 'NONE',  ( 9.361729212764000607, -77.35447091705098899, 6.367909160671999302 ) ) ;
#50465=CARTESIAN_POINT ( 'NONE',  ( 8.193575559979001000, -79.12595488940898747, 5.316613930189999948 ) ) ;
#50466=ORIENTED_EDGE ( 'NONE', *, *, #53848, .T. ) ;
#50475=FACE_OUTER_BOUND ( 'NONE', #27283, .T. ) ;
#50494=CARTESIAN_POINT ( 'NONE',  ( 9.705842814688999454, -77.07780893925938415, -0.1680204891633000075 ) ) ;
#50495=CARTESIAN_POINT ( 'NONE',  ( -9.372147444698367025, -77.17635552105011243, -0.1981913680696959501 ) ) ;
#50499=CARTESIAN_POINT ( 'NONE',  ( -5.120069445942999842, -77.28733258133598838, -8.157089945504001349 ) ) ;
#50504=ADVANCED_FACE ( 'NONE', ( #55993 ), #33535, .T. ) ;
#50509=CARTESIAN_POINT ( 'NONE',  ( -10.13785388426000011, -78.52174770179199470, -4.205702700205000255 ) ) ;
#50515=ORIENTED_EDGE ( 'NONE', *, *, #3561, .T. ) ;
#50526=CARTESIAN_POINT ( 'NONE',  ( 8.082524092276875294, -79.79166666666665719, 4.658475568430836766 ) ) ;
#50527=CARTESIAN_POINT ( 'NONE',  ( 10.85747675193891304, -79.21179631784005437, 1.607176855388187331 ) ) ;
#50535=EDGE_CURVE ( 'NONE', #56968, #24330, #21770, .T. ) ;
#50538=AXIS2_PLACEMENT_3D ( 'NONE', #13243, #44256, #26819 ) ;
#50547=CARTESIAN_POINT ( 'NONE',  ( 9.249208706614014730, -77.35106389758399814, 0.1238019141922536842 ) ) ;
#50548=CARTESIAN_POINT ( 'NONE',  ( 1.160587285869999929, -77.73646750513898951, 10.97894289003999901 ) ) ;
#50551=CARTESIAN_POINT ( 'NONE',  ( 1.487026788147999934, -77.52769675770798585, -9.589549613196998834 ) ) ;
#50556=CARTESIAN_POINT ( 'NONE',  ( -0.6493855936264999462, -79.80891271007898524, 10.92090362500000111 ) ) ;
#50560=ORIENTED_EDGE ( 'NONE', *, *, #32747, .F. ) ;
#50561=CARTESIAN_POINT ( 'NONE',  ( -10.80510142227721282, -77.19999999999998863, 1.932663460688196500 ) ) ;
#50570=CARTESIAN_POINT ( 'NONE',  ( 8.774584709929998283, -78.85553623779898658, 3.021992008916999595 ) ) ;
#50582=CARTESIAN_POINT ( 'NONE',  ( 3.303001513109999898, -78.95887072009900010, -10.46681410869999951 ) ) ;
#50583=DIRECTION ( 'NONE',  ( -1.000000000000000000, 0.000000000000000000, 0.000000000000000000 ) ) ;
#50596=CARTESIAN_POINT ( 'NONE',  ( -5.117553686986000550, -78.26666441077600211, -10.03691081092000026 ) ) ;
#50601=DIRECTION ( 'NONE',  ( 0.000000000000000000, -1.000000000000000000, -1.718649962392999796E-13 ) ) ;
#50602=DIRECTION ( 'NONE',  ( -1.000000000000000000, 0.000000000000000000, 0.000000000000000000 ) ) ;
#50620=CARTESIAN_POINT ( 'NONE',  ( 5.314949332417438832, -78.27388777455939817, -7.570571360755021573 ) ) ;
#50623=ORIENTED_EDGE ( 'NONE', *, *, #31148, .T. ) ;
#50624=CARTESIAN_POINT ( 'NONE',  ( -8.697226998145453081, -77.57235979624698530, 3.151704567404991053 ) ) ;
#50627=EDGE_CURVE ( 'NONE', #49672, #43122, #29324, .T. ) ;
#50629=CARTESIAN_POINT ( 'NONE',  ( -8.592320330817999618, -78.23138195110698234, 4.510292750937000328 ) ) ;
#50632=CIRCLE ( 'NONE', #51560, 4.100000000000000533 ) ;
#50643=CARTESIAN_POINT ( 'NONE',  ( -4.399010402408173093, -80.42916666666943115, -9.895799249887454963 ) ) ;
#50649=CARTESIAN_POINT ( 'NONE',  ( 10.59040229099152874, -77.20000000000000284, -2.027287110957618932 ) ) ;
#50650=ORIENTED_EDGE ( 'NONE', *, *, #12879, .T. ) ;
#50652=CARTESIAN_POINT ( 'NONE',  ( -11.40562379108000002, -78.11535612247598692, 0.7834358085291999174 ) ) ;
#50661=CARTESIAN_POINT ( 'NONE',  ( -11.15274311834000009, -77.24684517626799618, -0.5305918353390000064 ) ) ;
#50666=CARTESIAN_POINT ( 'NONE',  ( -9.379486438909999890, -78.02756575905399927, -0.7977647835019999745 ) ) ;
#50669=CARTESIAN_POINT ( 'NONE',  ( -1.150280981678749370, -80.21041666702008399, -10.98958334528740899 ) ) ;
#50695=CARTESIAN_POINT ( 'NONE',  ( -8.771572603219439657, -77.88508160123497248, -4.151306042262981499 ) ) ;
#50706=CARTESIAN_POINT ( 'NONE',  ( 7.406672800339156204, -78.79889337847342290, -5.541606015867000856 ) ) ;
#50708=FACE_OUTER_BOUND ( 'NONE', #56613, .T. ) ;
#50709=CARTESIAN_POINT ( 'NONE',  ( -10.24927991466481458, -80.12999227341786934, -3.994845400455109719 ) ) ;
#50711=CIRCLE ( 'NONE', #13898, 1.000000000000000000 ) ;
#50718=CARTESIAN_POINT ( 'NONE',  ( 5.821064686149081346, -79.99999999999998579, 7.358320351470873710 ) ) ;
#50727=CARTESIAN_POINT ( 'NONE',  ( -7.319319664381377599, -77.51649663083381370, -7.993250365100486476 ) ) ;
#50733=ORIENTED_EDGE ( 'NONE', *, *, #23041, .F. ) ;
#50736=CARTESIAN_POINT ( 'NONE',  ( 8.112428353360469302, -78.31019145401509718, -4.445158527088241662 ) ) ;
#50740=CARTESIAN_POINT ( 'NONE',  ( 5.949632932387999951, -78.00648151147798615, -7.711132450962999485 ) ) ;
#50753=CARTESIAN_POINT ( 'NONE',  ( 2.255546383061999727, -78.07046773478798229, -10.87004418268000094 ) ) ;
#50755=ORIENTED_EDGE ( 'NONE', *, *, #2161, .T. ) ;
#50761=CARTESIAN_POINT ( 'NONE',  ( 8.944729675425000082, -79.67334768894899355, 3.923329690209000908 ) ) ;
#50765=ORIENTED_EDGE ( 'NONE', *, *, #41128, .F. ) ;
#50771=EDGE_CURVE ( 'NONE', #33815, #2535, #28392, .T. ) ;
#50772=CARTESIAN_POINT ( 'NONE',  ( 7.267042919475000140, -76.96477995979998354, -6.172551194186000068 ) ) ;
#50785=DIRECTION ( 'NONE',  ( 0.000000000000000000, -1.000000000000000000, 0.000000000000000000 ) ) ;
#50794=CARTESIAN_POINT ( 'NONE',  ( 7.350012343602999820, -77.40102789785198922, -6.223385617129999936 ) ) ;
#50803=CARTESIAN_POINT ( 'NONE',  ( -0.5193979750644999172, -79.11168714277798131, -10.96331347381999954 ) ) ;
#50806=CARTESIAN_POINT ( 'NONE',  ( -7.858535633446000368, -79.69256872134099012, -5.635447047609000393 ) ) ;
#50820=CARTESIAN_POINT ( 'NONE',  ( 1.210822168571035418, -79.86458333333334281, 9.250000000000007105 ) ) ;
#50821=CARTESIAN_POINT ( 'NONE',  ( 10.03798773386740706, -79.48458675554202557, 4.654823617294058025 ) ) ;
#50829=DIRECTION ( 'NONE',  ( 0.000000000000000000, -1.000000000000000000, 0.000000000000000000 ) ) ;
#50840=CARTESIAN_POINT ( 'NONE',  ( 9.110268537203129569, -77.36402492828145228, 1.602260397345456333 ) ) ;
#50841=CIRCLE ( 'NONE', #8500, 9.549999999999998934 ) ;
#50843=CARTESIAN_POINT ( 'NONE',  ( 9.051070938631999852, -77.66981590335299757, 3.499832029064999794 ) ) ;
#50850=CARTESIAN_POINT ( 'NONE',  ( -6.384381598444999639, -78.85377266276799446, 8.884114358872000849 ) ) ;
#50852=EDGE_CURVE ( 'NONE', #50169, #3901, #55700, .T. ) ;
#50853=B_SPLINE_CURVE_WITH_KNOTS ( 'NONE', 3,
 ( #21931, #53830, #8656, #35801, #43818, #3646, #34638, #31363, #17217, #49407, #8360, #30208, #8075, #48253, #26642, #52666, #21649, #13365 ),
 .UNSPECIFIED., .F., .F.,
 ( 4, 2, 2, 2, 2, 2, 2, 2, 4 ),
 ( 0.000000000000000000, 0.1250000000000000278, 0.2500000000000000000, 0.3750000000000001110, 0.5000000000000001110, 0.6250000000000001110, 0.7500000000000002220, 0.8750000000000001110, 1.000000000000000000 ),
 .UNSPECIFIED. ) ;
#50865=CARTESIAN_POINT ( 'NONE',  ( -1.518219907972000016, -78.46707723970298787, 9.290113175764000530 ) ) ;
#50875=CARTESIAN_POINT ( 'NONE',  ( 8.212410987726999068, -78.06403359845799628, -6.936771999183999782 ) ) ;
#50900=ORIENTED_EDGE ( 'NONE', *, *, #27746, .F. ) ;
#50905=FACE_OUTER_BOUND ( 'NONE', #55610, .T. ) ;
#50909=CARTESIAN_POINT ( 'NONE',  ( 1.811390969245943783, -78.24081207420749706, -9.070829909341801667 ) ) ;
#50914=CARTESIAN_POINT ( 'NONE',  ( -9.136563440606458641, -77.58766556716409468, 1.443667254356420404 ) ) ;
#50918=CARTESIAN_POINT ( 'NONE',  ( -9.139898499914998808, -77.18571961563208106, 2.826942883852999966 ) ) ;
#50924=EDGE_CURVE ( 'NONE', #45083, #16241, #55771, .T. ) ;
#50938=CARTESIAN_POINT ( 'NONE',  ( 9.739528811734443181, -77.20000000000001705, -4.689215945816418873 ) ) ;
#50939=VERTEX_POINT ( 'NONE', #5995 ) ;
#50940=CARTESIAN_POINT ( 'NONE',  ( 1.439896632895334649, -78.33541666666666003, -10.99999999999999822 ) ) ;
#50949=CARTESIAN_POINT ( 'NONE',  ( 0.9943957917579000494, -77.87515876690598304, -11.12098945592000021 ) ) ;
#50950=( GEOMETRIC_REPRESENTATION_CONTEXT ( 3 ) GLOBAL_UNCERTAINTY_ASSIGNED_CONTEXT ( ( #15398 ) ) GLOBAL_UNIT_ASSIGNED_CONTEXT ( ( #35539, #53568, #44132 ) ) REPRESENTATION_CONTEXT ( 'NONE', 'WORKASPACE' ) );
#50957=FACE_BOUND ( 'NONE', #28065, .T. ) ;
#50977=EDGE_LOOP ( 'NONE', ( #3523, #44649, #40574, #13182 ) ) ;
#50983=CARTESIAN_POINT ( 'NONE',  ( 3.248398814366682430, -78.19774372165396414, 9.144491945039828096 ) ) ;
#50987=CARTESIAN_POINT ( 'NONE',  ( -7.456816947376000648, -78.69473898445177440, 6.210200510404997765 ) ) ;
#50992=ADVANCED_FACE ( 'NONE', ( #52905 ), #14281, .F. ) ;
#50993=CARTESIAN_POINT ( 'NONE',  ( -6.532098792667899723, -78.66264509723824006, -6.549319641915878343 ) ) ;
#50999=CARTESIAN_POINT ( 'NONE',  ( -6.333048277618449795, -80.17656323135794594, -8.998749364487563795 ) ) ;
#51020=VERTEX_POINT ( 'NONE', #30449 ) ;
#51024=CARTESIAN_POINT ( 'NONE',  ( 8.350655305475967793, -78.31463735380187074, -3.978570201286235619 ) ) ;
#51028=CARTESIAN_POINT ( 'NONE',  ( -4.441436338936000539, -78.97991978438899707, -8.545575054271999704 ) ) ;
#51040=CARTESIAN_POINT ( 'NONE',  ( -9.222505265117137085, -77.51202912837678127, -1.397969593980213476 ) ) ;
#51041=DIRECTION ( 'NONE',  ( 1.000000000000000000, 0.000000000000000000, 0.000000000000000000 ) ) ;
#51045=CARTESIAN_POINT ( 'NONE',  ( -1.346801222098000128, -77.94142625569698168, 11.24181324638000135 ) ) ;
#51051=CARTESIAN_POINT ( 'NONE',  ( 6.653382217586999658, -79.70582034720699482, 7.150748904218000135 ) ) ;
#51064=CARTESIAN_POINT ( 'NONE',  ( 9.532486246840001343, -76.90082656998458788, -2.044978076835000103 ) ) ;
#51071=DIRECTION ( 'NONE',  ( 0.000000000000000000, 0.000000000000000000, -1.000000000000000000 ) ) ;
#51081=CARTESIAN_POINT ( 'NONE',  ( -9.463706838924000664, -77.33890260894099811, -1.161272537025000107 ) ) ;
#51086=CARTESIAN_POINT ( 'NONE',  ( -0.5506691749702000704, -77.82738533478698173, -9.615090921292999582 ) ) ;
#51089=CARTESIAN_POINT ( 'NONE',  ( 1.229229935955506336, -77.05286458334455801, 9.397135416926557738 ) ) ;
#51092=VERTEX_POINT ( 'NONE', #38743 ) ;
#51094=EDGE_CURVE ( 'NONE', #16896, #44068, #9579, .T. ) ;
#51095=CARTESIAN_POINT ( 'NONE',  ( 9.499549289235639904, -79.50042064254546403, 0.05021470316550929319 ) ) ;
#51097=VECTOR ( 'NONE', #57278, 1000.000000000000000 ) ;
#51098=CARTESIAN_POINT ( 'NONE',  ( 10.85730540529999999, -79.25214891444099408, 1.607151491820999922 ) ) ;
#51100=CARTESIAN_POINT ( 'NONE',  ( -10.68954194898181775, -80.08091480521125050, 2.624713457052874510 ) ) ;
#51101=CARTESIAN_POINT ( 'NONE',  ( 3.185501216392000234, -79.99134998740498759, 9.130619404448999887 ) ) ;
#51116=CARTESIAN_POINT ( 'NONE',  ( 3.303053640057958429, -79.09942690050905867, -10.46697929272314731 ) ) ;
#51134=CARTESIAN_POINT ( 'NONE',  ( 7.827287555285567855, -77.39497157051955867, 4.939251125549445121 ) ) ;
#51135=CARTESIAN_POINT ( 'NONE',  ( -5.876696946710000091, -77.57078597849198331, -9.346046374399000101 ) ) ;
#51141=CARTESIAN_POINT ( 'NONE',  ( 0.000000000000000000, -79.99999999999998579, 0.000000000000000000 ) ) ;
#51143=CARTESIAN_POINT ( 'NONE',  ( 0.2631036358232000105, -79.61995726186898992, -11.04575348828999992 ) ) ;
#51148=ORIENTED_EDGE ( 'NONE', *, *, #28425, .T. ) ;
#51149=CARTESIAN_POINT ( 'NONE',  ( -10.28202908126049664, -77.20000000000000284, 3.778194283757810190 ) ) ;
#51157=CARTESIAN_POINT ( 'NONE',  ( -0.1492691421716000055, -77.95544831538099118, 9.412168359664999429 ) ) ;
#51159=ADVANCED_FACE ( 'NONE', ( #46035 ), #47273, .F. ) ;
#51169=CARTESIAN_POINT ( 'NONE',  ( -4.399243655502999673, -79.71736428708098288, 10.05537673064999815 ) ) ;
#51181=DIRECTION ( 'NONE',  ( 0.000000000000000000, 1.000000000000000000, 1.487781318828000208E-14 ) ) ;
#51195=ORIENTED_EDGE ( 'NONE', *, *, #19257, .T. ) ;
#51197=ORIENTED_EDGE ( 'NONE', *, *, #50535, .T. ) ;
#51206=CARTESIAN_POINT ( 'NONE',  ( 6.153210332247711634, -78.28297894785262656, -6.906877943483819671 ) ) ;
#51209=ORIENTED_EDGE ( 'NONE', *, *, #26606, .F. ) ;
#51210=CARTESIAN_POINT ( 'NONE',  ( -9.137867255240424313, -77.58773879498612303, 1.435393631043841989 ) ) ;
#51214=CARTESIAN_POINT ( 'NONE',  ( -7.843978203195000276, -77.71975302678599462, 5.713380375430999969 ) ) ;
#51225=CARTESIAN_POINT ( 'NONE',  ( -10.97916666637321192, -80.22083333335037025, -1.151917308728376499 ) ) ;
#51233=ORIENTED_EDGE ( 'NONE', *, *, #47920, .T. ) ;
#51238=CARTESIAN_POINT ( 'NONE',  ( 8.462293916759000112, -79.74502648735098376, 4.390897894491000208 ) ) ;
#51244=EDGE_CURVE ( 'NONE', #46717, #1524, #36274, .T. ) ;
#51246=CARTESIAN_POINT ( 'NONE',  ( -6.629376284316999879, -77.75416360879198407, -9.119063026537000738 ) ) ;
#51250=CARTESIAN_POINT ( 'NONE',  ( -0.5382333298950999767, -78.14126107556998591, -9.397951872088000869 ) ) ;
#51254=DIRECTION ( 'NONE',  ( 0.000000000000000000, -1.000000000000000000, -1.567610190497999989E-13 ) ) ;
#51266=ORIENTED_EDGE ( 'NONE', *, *, #36869, .T. ) ;
#51267=EDGE_LOOP ( 'NONE', ( #19387, #56617, #20258, #22126 ) ) ;
#51269=ORIENTED_EDGE ( 'NONE', *, *, #22853, .T. ) ;
#51276=CARTESIAN_POINT ( 'NONE',  ( 11.00000000000000000, -77.34999999999999432, 0.000000000000000000 ) ) ;
#51278=CARTESIAN_POINT ( 'NONE',  ( -9.010298068253861814, -79.12116754975356514, -2.421818492791191879 ) ) ;
#51283=CARTESIAN_POINT ( 'NONE',  ( 3.248345031020999585, -78.09783857274324248, 9.144340540792999406 ) ) ;
#51285=CARTESIAN_POINT ( 'NONE',  ( 2.510256491861835748, -79.99607450634006511, -9.173255752048776301 ) ) ;
#51287=CARTESIAN_POINT ( 'NONE',  ( -7.969114183967002774, -78.64255665622569325, -4.697662469176757227 ) ) ;
#51295=EDGE_CURVE ( 'NONE', #34022, #29378, #17171, .T. ) ;
#51307=CARTESIAN_POINT ( 'NONE',  ( 3.132406251486010262, -77.80199808890452573, 10.30751908724726462 ) ) ;
#51309=CARTESIAN_POINT ( 'NONE',  ( 0.2613587267741000475, -79.47689468395957135, -10.97249781033000282 ) ) ;
#51315=CARTESIAN_POINT ( 'NONE',  ( 8.822708684726574546, -78.32582670471354902, -2.780085958306391269 ) ) ;
#51319=CARTESIAN_POINT ( 'NONE',  ( 9.617254819657999221, -78.63883383484099454, -0.5114877307952000463 ) ) ;
#51321=CARTESIAN_POINT ( 'NONE',  ( 2.872516177058867193, -80.22864583377563008, -10.68547302994066506 ) ) ;
#51324=ORIENTED_EDGE ( 'NONE', *, *, #45373, .T. ) ;
#51330=CARTESIAN_POINT ( 'NONE',  ( 7.305616453585000336, -79.99970782078999321, 8.949732329072000780 ) ) ;
#51333=CARTESIAN_POINT ( 'NONE',  ( 8.223067162435999222, -77.93193257914899164, 7.942492809189998226 ) ) ;
#51339=CARTESIAN_POINT ( 'NONE',  ( -8.396223008680999911, -80.29268748536451028, -4.990405176070999538 ) ) ;
#51351=CARTESIAN_POINT ( 'NONE',  ( 6.969509891012999780, -76.97926403785729121, 6.817479844763999708 ) ) ;
#51353=B_SPLINE_CURVE_WITH_KNOTS ( 'NONE', 3,
 ( #14625, #32617, #50669, #37354 ),
 .UNSPECIFIED., .F., .F.,
 ( 4, 4 ),
 ( 0.000000000000000000, 0.1666666723472590150 ),
 .UNSPECIFIED. ) ;
#51362=FACE_OUTER_BOUND ( 'NONE', #8265, .T. ) ;
#51366=CARTESIAN_POINT ( 'NONE',  ( 0.000000000000000000, -80.99999999999998579, 0.000000000000000000 ) ) ;
#51369=CARTESIAN_POINT ( 'NONE',  ( 9.139046933839001241, -77.16779404701080125, 2.935455237353000069 ) ) ;
#51374=CARTESIAN_POINT ( 'NONE',  ( -8.803456334546002182, -77.80598958818299593, -4.166395597179999299 ) ) ;
#51379=ORIENTED_EDGE ( 'NONE', *, *, #12772, .F. ) ;
#51387=CARTESIAN_POINT ( 'NONE',  ( -9.189896052897999823, -79.61787340482499076, 3.010092405580000019 ) ) ;
#51404=EDGE_CURVE ( 'NONE', #44068, #56968, #24156, .T. ) ;
#51415=EDGE_CURVE ( 'NONE', #35917, #14347, #6793, .T. ) ;
#51422=CONICAL_SURFACE ( 'NONE', #54234, 4.199999999676998996, 0.7853981633972997312 ) ;
#51426=CARTESIAN_POINT ( 'NONE',  ( 8.143624268315699410, -77.38946596373423858, 4.387306811431966658 ) ) ;
#51431=AXIS2_PLACEMENT_3D ( 'NONE', #15350, #23906, #29487 ) ;
#51436=CARTESIAN_POINT ( 'NONE',  ( 7.366954953549999630, -79.67614197053399039, -8.234431878459000487 ) ) ;
#51442=CARTESIAN_POINT ( 'NONE',  ( -10.72633970217810173, -77.20000000000001705, 2.335726820744686183 ) ) ;
#51450=CARTESIAN_POINT ( 'NONE',  ( -8.852983674280999082, -78.67307212613098955, -3.506430706099999739 ) ) ;
#51461=CARTESIAN_POINT ( 'NONE',  ( 8.867070753125000593, -78.50939305077599784, -6.468312982590000537 ) ) ;
#51472=CARTESIAN_POINT ( 'NONE',  ( -8.859962374443000499, -78.12620263911298935, 6.959166695099000322 ) ) ;
#51489=CARTESIAN_POINT ( 'NONE',  ( 9.401479492988663367, -79.98662458792078667, -1.597696805283046917 ) ) ;
#51492=CARTESIAN_POINT ( 'NONE',  ( -11.11771682179999843, -80.33756661863206716, 1.751409206030000165 ) ) ;
#51493=PRODUCT_CONTEXT ( 'NONE', #55283, 'mechanical' ) ;
#51497=CARTESIAN_POINT ( 'NONE',  ( 5.143522193159038025, -78.27208594951937926, -7.687965448588824913 ) ) ;
#51501=CARTESIAN_POINT ( 'NONE',  ( -8.840280758047018850, -77.57624239855847748, 2.722759996602876598 ) ) ;
#51502=CARTESIAN_POINT ( 'NONE',  ( 11.00000000000000000, -77.84999999999999432, 0.000000000000000000 ) ) ;
#51504=CARTESIAN_POINT ( 'NONE',  ( -0.1538805260928999830, -78.14611046371997816, 9.702939253146000809 ) ) ;
#51513=CARTESIAN_POINT ( 'NONE',  ( -5.427146848547155678, -80.40833333333752364, -9.396180599229785102 ) ) ;
#51527=ADVANCED_FACE ( 'NONE', ( #15884 ), #53735, .F. ) ;
#51531=CARTESIAN_POINT ( 'NONE',  ( 1.659133085963000021, -80.03182264566298443, -9.498693983952000153 ) ) ;
#51537=CARTESIAN_POINT ( 'NONE',  ( 10.81029799801000024, -78.05327334234998204, -0.4981644331059998931 ) ) ;
#51540=CARTESIAN_POINT ( 'NONE',  ( -0.1492691421716000055, -78.39707553773099846, 9.412168359664999429 ) ) ;
#51546=ADVANCED_FACE ( 'NONE', ( #3457 ), #47359, .F. ) ;
#51556=VECTOR ( 'NONE', #28923, 1000.000000000000000 ) ;
#51560=AXIS2_PLACEMENT_3D ( 'NONE', #43078, #24773, #20632 ) ;
#51572=DIRECTION ( 'NONE',  ( -1.000000000000000000, 0.000000000000000000, 0.000000000000000000 ) ) ;
#51574=CARTESIAN_POINT ( 'NONE',  ( -8.592320330817999618, -78.21153388925924332, 4.510292750937000328 ) ) ;
#51576=CARTESIAN_POINT ( 'NONE',  ( 9.400053674151607197, -79.57946385258328803, -2.458488295831327441 ) ) ;
#51578=CARTESIAN_POINT ( 'NONE',  ( 10.99999999999999822, -78.46041666666668846, 1.439896632895345086 ) ) ;
#51581=CARTESIAN_POINT ( 'NONE',  ( -7.279424256080870848, -78.65297865939129451, -5.707278038144436572 ) ) ;
#51584=CARTESIAN_POINT ( 'NONE',  ( -5.645349303483418346, -80.18225419666993048, -9.440761718514824707 ) ) ;
#51599=CARTESIAN_POINT ( 'NONE',  ( 4.421533069776005576, -77.79180160825917767, 9.823367980291944690 ) ) ;
#51601=CARTESIAN_POINT ( 'NONE',  ( -8.758795259761319230, -79.80031661833969281, 6.307149791603988476 ) ) ;
#51608=CARTESIAN_POINT ( 'NONE',  ( 9.184444922356584939, -78.34058259241612632, -1.099429577161610938 ) ) ;
#51612=CARTESIAN_POINT ( 'NONE',  ( -6.791097082272000485, -77.89278619496199951, -6.981453725808999700 ) ) ;
#51623=CARTESIAN_POINT ( 'NONE',  ( 10.62704985177000161, -78.53487766400598957, -3.023855997759000047 ) ) ;
#51628=CARTESIAN_POINT ( 'NONE',  ( -11.04512294322999999, -77.57457916904299111, -2.489477414621999785 ) ) ;
#51632=ORIENTED_EDGE ( 'NONE', *, *, #17478, .T. ) ;
#51635=CARTESIAN_POINT ( 'NONE',  ( -5.809791519574999619, -79.43600129156250489, 7.851562197947999699 ) ) ;
#51639=ORIENTED_EDGE ( 'NONE', *, *, #267, .F. ) ;
#51642=CIRCLE ( 'NONE', #53506, 1.000000000000000000 ) ;
#51648=B_SPLINE_CURVE_WITH_KNOTS ( 'NONE', 3,
 ( #12154, #56745, #52033, #16305, #11588, #34282, #29851, #47904, #7436, #25437, #52602, #30140, #8881, #18037, #31000, #21866, #26876, #44902 ),
 .UNSPECIFIED., .F., .F.,
 ( 4, 2, 2, 2, 2, 2, 2, 2, 4 ),
 ( 0.000000000000000000, 0.1250000000000000555, 0.2500000000000001110, 0.3750000000000001665, 0.5000000000000001110, 0.6250000000000001110, 0.7500000000000002220, 0.8750000000000001110, 1.000000000000000000 ),
 .UNSPECIFIED. ) ;
#51649=CARTESIAN_POINT ( 'NONE',  ( 7.070456480284000200, -76.81002177417249754, -6.005572703287999303 ) ) ;
#51652=CARTESIAN_POINT ( 'NONE',  ( -5.539808784079886195, -79.68333333333332291, -9.611650271896841957 ) ) ;
#51653=EDGE_CURVE ( 'NONE', #15394, #1613, #236, .T. ) ;
#51664=ADVANCED_FACE ( 'NONE', ( #32053 ), #45670, .F. ) ;
#51667=CARTESIAN_POINT ( 'NONE',  ( 2.317704416658000088, -76.97337147138669877, -9.426556171238999582 ) ) ;
#51672=CARTESIAN_POINT ( 'NONE',  ( -7.484045594489000308, -78.71555212030999371, 6.232877124219999843 ) ) ;
#51674=CARTESIAN_POINT ( 'NONE',  ( 5.790379962074457154, -77.02682291667791503, 7.536004869419408614 ) ) ;
#51679=CARTESIAN_POINT ( 'NONE',  ( -2.421407277241032219, -77.99599274655952286, 9.009652519855267272 ) ) ;
#51682=CARTESIAN_POINT ( 'NONE',  ( -10.48173540582233976, -80.07564442187884879, 3.336307010942487938 ) ) ;
#51683=CARTESIAN_POINT ( 'NONE',  ( -7.869048196118999527, -79.03113044843098578, 5.428549196144000000 ) ) ;
#51700=CARTESIAN_POINT ( 'NONE',  ( 9.647254834573999460, -79.94705612754898993, -1.526580663425000095 ) ) ;
#51710=DIRECTION ( 'NONE',  ( 0.000000000000000000, -1.000000000000000000, 0.000000000000000000 ) ) ;
#51715=EDGE_LOOP ( 'NONE', ( #46326, #47104 ) ) ;
#51717=CARTESIAN_POINT ( 'NONE',  ( 8.640831906552849162, -77.37907852117427865, 3.303617862035461261 ) ) ;
#51718=CARTESIAN_POINT ( 'NONE',  ( -10.47078769031000078, -78.01612189980698986, -3.499536356729999742 ) ) ;
#51726=CARTESIAN_POINT ( 'NONE',  ( 3.941639820121999094, -79.33903371854199804, 10.32188786877999931 ) ) ;
#51729=EDGE_CURVE ( 'NONE', #11813, #55607, #35605, .T. ) ;
#51735=EDGE_CURVE ( 'NONE', #16241, #44715, #3907, .T. ) ;
#51741=CARTESIAN_POINT ( 'NONE',  ( 1.846868607710999921, -78.50252915135698117, 9.341276817324001058 ) ) ;
#51751=CARTESIAN_POINT ( 'NONE',  ( 5.330173052271000245, -78.26479829579199077, 9.594439332582000546 ) ) ;
#51757=ORIENTED_EDGE ( 'NONE', *, *, #29220, .T. ) ;
#51760=CARTESIAN_POINT ( 'NONE',  ( -11.00000000000000000, -78.19999999999998863, 0.000000000000000000 ) ) ;
#51761=CARTESIAN_POINT ( 'NONE',  ( -8.192247052095000370, -78.30244779722698922, -7.574872137178000564 ) ) ;
#51770=ORIENTED_EDGE ( 'NONE', *, *, #17071, .T. ) ;
#51774=DIRECTION ( 'NONE',  ( 0.000000000000000000, 1.000000000000000000, 0.000000000000000000 ) ) ;
#51778=ORIENTED_EDGE ( 'NONE', *, *, #51729, .F. ) ;
#51782=AXIS2_PLACEMENT_3D ( 'NONE', #19907, #20484, #11344 ) ;
#51787=CARTESIAN_POINT ( 'NONE',  ( -1.787026317784608631, -78.20960545061939229, -9.075693917138710987 ) ) ;
#51788=CARTESIAN_POINT ( 'NONE',  ( -7.409043029364259958, -79.44809193424394778, 5.667876244604902247 ) ) ;
#51794=CARTESIAN_POINT ( 'NONE',  ( -0.1538805260929999863, -78.20641338939098830, 9.702939253146000809 ) ) ;
#51809=CARTESIAN_POINT ( 'NONE',  ( -4.124900980777000292, -80.39812822292799410, 10.39307513819000128 ) ) ;
#51818=CARTESIAN_POINT ( 'NONE',  ( -8.807539493945000686, -79.35970150572998705, 3.924989019749000274 ) ) ;
#51821=DIRECTION ( 'NONE',  ( 0.000000000000000000, 1.000000000000000000, 0.000000000000000000 ) ) ;
#51828=CARTESIAN_POINT ( 'NONE',  ( -0.008152559635135000343, -77.74587287048397855, 10.94781514982000203 ) ) ;
#51833=CARTESIAN_POINT ( 'NONE',  ( -1.210822168571075830, -78.38541666666668561, 9.250000000000000000 ) ) ;
#51834=CARTESIAN_POINT ( 'NONE',  ( -10.71369944335148183, -77.57916666666665151, 2.879226727952040932 ) ) ;
#51837=LINE ( 'NONE', #1961, #262 ) ;
#51838=EDGE_CURVE ( 'NONE', #33222, #2177, #49183, .T. ) ;
#51852=ORIENTED_EDGE ( 'NONE', *, *, #2432, .F. ) ;
#51863=CARTESIAN_POINT ( 'NONE',  ( -3.574427999287489222, -79.75479980213101783, 9.034856847799710877 ) ) ;
#51864=CARTESIAN_POINT ( 'NONE',  ( -0.5175072279577125345, -76.97066086130449492, -9.610596997971313726 ) ) ;
#51866=CARTESIAN_POINT ( 'NONE',  ( -3.532846115401338860, -78.69390980651986922, -8.548707026569838163 ) ) ;
#51884=CARTESIAN_POINT ( 'NONE',  ( -9.429661037469928786, -77.99063298084412565, -5.207437231424048463 ) ) ;
#51894=CARTESIAN_POINT ( 'NONE',  ( -9.721291027688000241, -77.32430961238299005, 0.5965459135820000425 ) ) ;
#51900=CARTESIAN_POINT ( 'NONE',  ( 0.000000000000000000, -81.10000000285099020, -7.000000000000000000 ) ) ;
#51906=CARTESIAN_POINT ( 'NONE',  ( 9.366620387600999464, -79.01244768766198945, -5.860402389062000061 ) ) ;
#51907=CARTESIAN_POINT ( 'NONE',  ( 10.90625000000000000, -80.29374999999798490, -5.301077343649000152E-10 ) ) ;
#51911=CARTESIAN_POINT ( 'NONE',  ( 8.143733331677999843, -77.86805683836598746, 7.865865880590998671 ) ) ;
#51917=CARTESIAN_POINT ( 'NONE',  ( -2.116314338179000387, -80.35763280188051283, -9.535298106756000536 ) ) ;
#51930=CARTESIAN_POINT ( 'NONE',  ( 6.905509799642000068, -76.92767797598149571, 6.754875825283999546 ) ) ;
#51936=CARTESIAN_POINT ( 'NONE',  ( 0.000000000000000000, -81.10000000285099020, -8.099999997149000208 ) ) ;
#51937=AXIS2_PLACEMENT_3D ( 'NONE', #541, #27058, #54535 ) ;
#51938=CARTESIAN_POINT ( 'NONE',  ( 7.069026039852619014, -77.18437499998694307, -6.033943155702938377 ) ) ;
#51947=CARTESIAN_POINT ( 'NONE',  ( -3.484330481557000425, -77.42609236341799317, 8.711138713857000226 ) ) ;
#51952=CARTESIAN_POINT ( 'NONE',  ( -0.1544424224854999972, -78.14707553773099846, 9.738369639964998825 ) ) ;
#51966=CARTESIAN_POINT ( 'NONE',  ( -8.082524092276882399, -79.04166666666665719, -4.658475568430820779 ) ) ;
#51991=CARTESIAN_POINT ( 'NONE',  ( -5.539808784079931492, -77.61666666666667425, 9.611650271896815312 ) ) ;
#52002=CARTESIAN_POINT ( 'NONE',  ( 5.510598863588248797, -77.27593132977736445, -7.429347641380793732 ) ) ;
#52003=CARTESIAN_POINT ( 'NONE',  ( -3.203604947276999848, -77.88888306514598980, 10.56508708803000118 ) ) ;
#52012=CARTESIAN_POINT ( 'NONE',  ( 9.696433660856000003, -79.28284900987598860, 5.296892287724999981 ) ) ;
#52023=VECTOR ( 'NONE', #38020, 1000.000000000000000 ) ;
#52027=CARTESIAN_POINT ( 'NONE',  ( 9.191740907676001271, -78.87203893003398036, -2.486449962426000138 ) ) ;
#52033=CARTESIAN_POINT ( 'NONE',  ( -9.009247259181927703, -78.97916666666665719, 2.421167930323307793 ) ) ;
#52037=CARTESIAN_POINT ( 'NONE',  ( 9.632126701410999914, -79.15963541743298038, 5.261763182588000021 ) ) ;
#52038=FACE_OUTER_BOUND ( 'NONE', #20666, .T. ) ;
#52041=CARTESIAN_POINT ( 'NONE',  ( 0.000000000000000000, -74.64999999999999147, 0.000000000000000000 ) ) ;
#52047=CARTESIAN_POINT ( 'NONE',  ( -3.770495512267000304, -79.08134268642398013, 10.61660482251999937 ) ) ;
#52070=CARTESIAN_POINT ( 'NONE',  ( -2.195394413746336593, -78.20598208360085835, -8.990872906390226404 ) ) ;
#52074=CARTESIAN_POINT ( 'NONE',  ( -5.331231741419041548, -77.52388645747066676, 7.560242739789973854 ) ) ;
#52077=CARTESIAN_POINT ( 'NONE',  ( -9.626984307556000431, -78.32010870590698914, 1.221426423741999834 ) ) ;
#52082=DIRECTION ( 'NONE',  ( 0.000000000000000000, 0.000000000000000000, -1.000000000000000000 ) ) ;
#52090=DIRECTION ( 'NONE',  ( -1.000000000000000000, 0.000000000000000000, 0.000000000000000000 ) ) ;
#52092=CARTESIAN_POINT ( 'NONE',  ( 9.250000000000000000, -79.34999999999999432, 0.000000000000000000 ) ) ;
#52093=CARTESIAN_POINT ( 'NONE',  ( 4.491149118889000036, -80.08742432477399120, -10.11991891289999934 ) ) ;
#52102=CARTESIAN_POINT ( 'NONE',  ( -8.544252929325999446, -79.92036243689798880, 4.229201381545000693 ) ) ;
#52107=CYLINDRICAL_SURFACE ( 'NONE', #54008, 11.00000000000000000 ) ;
#52110=CARTESIAN_POINT ( 'NONE',  ( 4.742897571346999186, -78.03146995713699141, -9.867095245577001350 ) ) ;
#52115=CARTESIAN_POINT ( 'NONE',  ( -9.429275737370000243, -77.33986768295099523, -1.157047565421999824 ) ) ;
#52130=ORIENTED_EDGE ( 'NONE', *, *, #47082, .T. ) ;
#52150=CARTESIAN_POINT ( 'NONE',  ( 1.439896632895284911, -78.56458333333330302, 11.00000000000000355 ) ) ;
#52153=CARTESIAN_POINT ( 'NONE',  ( -5.137582680770506727, -78.67826736333080362, -7.691962846148583388 ) ) ;
#52182=CARTESIAN_POINT ( 'NONE',  ( -3.509962959857999554, -78.29774788529299201, 8.968465308258000590 ) ) ;
#52187=CARTESIAN_POINT ( 'NONE',  ( 9.549999999953000085, -76.40000000004698677, -5.125981083096999748E-10 ) ) ;
#52190=CARTESIAN_POINT ( 'NONE',  ( -8.603527126503999867, -78.31782986146299663, 6.757746467621000619 ) ) ;
#52193=CARTESIAN_POINT ( 'NONE',  ( -11.16546426881000009, -79.79336997964799139, 1.922701916112000031 ) ) ;
#52201=CARTESIAN_POINT ( 'NONE',  ( 6.653382217586999658, -79.94552603410404856, 7.150748904218000135 ) ) ;
#52223=EDGE_CURVE ( 'NONE', #3961, #31318, #49556, .T. ) ;
#52227=CARTESIAN_POINT ( 'NONE',  ( -6.105583392804999399, -77.45220173038597977, 7.123643952372000321 ) ) ;
#52232=CARTESIAN_POINT ( 'NONE',  ( 9.292856425461000214, -78.54500914553598534, 2.915907262279999745 ) ) ;
#52241=EDGE_CURVE ( 'NONE', #40940, #37542, #6665, .T. ) ;
#52242=CARTESIAN_POINT ( 'NONE',  ( -1.053982531448302229, -79.36617011479219741, -9.467004606927948984 ) ) ;
#52243=CARTESIAN_POINT ( 'NONE',  ( -2.194599507562917218, -80.00000000000001421, -9.198212786487998116 ) ) ;
#52246=CARTESIAN_POINT ( 'NONE',  ( -4.668381075099000022, -79.12153427173898024, 8.594720803921001462 ) ) ;
#52248=CARTESIAN_POINT ( 'NONE',  ( 2.421167930323352646, -79.14583333333334281, -9.009247259181915268 ) ) ;
#52264=CARTESIAN_POINT ( 'NONE',  ( 9.767191983224998708, -79.45996625367898503, 0.05162932631433000269 ) ) ;
#52265=ORIENTED_EDGE ( 'NONE', *, *, #30039, .T. ) ;
#52276=CYLINDRICAL_SURFACE ( 'NONE', #17337, 4.100000000000000533 ) ;
#52279=CARTESIAN_POINT ( 'NONE',  ( -0.8787709177018370177, -79.98266234880088632, 9.208350210453216889 ) ) ;
#52283=CARTESIAN_POINT ( 'NONE',  ( -11.10294551207000069, -79.60724697177198550, 1.911422329490000127 ) ) ;
#52284=CARTESIAN_POINT ( 'NONE',  ( 5.650948687534441461, -77.27745941166017474, -7.323274689015353722 ) ) ;
#52293=CARTESIAN_POINT ( 'NONE',  ( -8.112440615085001028, -78.55244779722698922, -7.501079983178001065 ) ) ;
#52296=CARTESIAN_POINT ( 'NONE',  ( 0.000000000000000000, -78.59999999921299718, 0.000000000000000000 ) ) ;
#52311=CARTESIAN_POINT ( 'NONE',  ( -3.833926501619000060, -77.73508576487398614, -8.716156481626001096 ) ) ;
#52316=VERTEX_POINT ( 'NONE', #45650 ) ;
#52318=CIRCLE ( 'NONE', #14618, 9.549999999999998934 ) ;
#52323=CARTESIAN_POINT ( 'NONE',  ( 10.87588596538000019, -79.60911308675498788, -1.476184626237000197 ) ) ;
#52324=DIRECTION ( 'NONE',  ( 0.000000000000000000, -1.000000000000000000, 0.000000000000000000 ) ) ;
#52327=DIRECTION ( 'NONE',  ( -1.000000000000000000, 0.000000000000000000, 0.000000000000000000 ) ) ;
#52332=DIRECTION ( 'NONE',  ( 1.000000000000000000, 0.000000000000000000, 0.000000000000000000 ) ) ;
#52333=CARTESIAN_POINT ( 'NONE',  ( -3.006161377376999955, -78.57568030843599161, 10.85780494109000038 ) ) ;
#52341=( NAMED_UNIT ( * ) PLANE_ANGLE_UNIT ( ) SI_UNIT ( $, .RADIAN. ) );
#52348=ORIENTED_EDGE ( 'NONE', *, *, #7679, .T. ) ;
#52351=ADVANCED_FACE ( 'NONE', ( #41199 ), #789, .T. ) ;
#52357=CARTESIAN_POINT ( 'NONE',  ( -3.292086955815877847, -78.19615833579152309, -8.644430884715466945 ) ) ;
#52358=CARTESIAN_POINT ( 'NONE',  ( -1.255625495614115295, -79.38580225533669932, 9.243491999774299472 ) ) ;
#52361=CARTESIAN_POINT ( 'NONE',  ( -3.114065545470247276, -77.50245480038890378, 8.710212348931921866 ) ) ;
#52362=CARTESIAN_POINT ( 'NONE',  ( 6.393001003723999709, -77.13539953215739331, 9.000752526674000720 ) ) ;
#52363=CARTESIAN_POINT ( 'NONE',  ( 11.00000000000000178, -78.34292008887531722, -0.9786566581934403874 ) ) ;
#52364=CARTESIAN_POINT ( 'NONE',  ( 6.240531904507999883, -78.14956573113299498, 7.431451467605000083 ) ) ;
#52367=CARTESIAN_POINT ( 'NONE',  ( 11.10498291493000167, -80.16715056412299134, -1.830582403018000015 ) ) ;
#52369=ADVANCED_FACE ( 'NONE', ( #25155 ), #11598, .F. ) ;
#52377=CARTESIAN_POINT ( 'NONE',  ( 9.009514222719491983, -78.37087597555611751, 2.421282354168349471 ) ) ;
#52380=CARTESIAN_POINT ( 'NONE',  ( -10.81434145419000181, -79.94637966341998947, -2.373591376386999574 ) ) ;
#52392=CARTESIAN_POINT ( 'NONE',  ( 3.858758824815000210, -80.05130441783499862, -8.679482335691000472 ) ) ;
#52398=CARTESIAN_POINT ( 'NONE',  ( -8.664714296349000477, -77.25360149971999135, 6.868106230948000324 ) ) ;
#52404=CARTESIAN_POINT ( 'NONE',  ( -9.009247259181929479, -78.47916666666665719, 2.421167930323313566 ) ) ;
#52434=CARTESIAN_POINT ( 'NONE',  ( -6.760013919724102038, -78.62708333333333144, 8.796335266379953666 ) ) ;
#52438=CARTESIAN_POINT ( 'NONE',  ( -10.69668321983107973, -80.11953358945446269, -2.665761377985893077 ) ) ;
#52449=EDGE_CURVE ( 'NONE', #17089, #18212, #41649, .T. ) ;
#52454=CARTESIAN_POINT ( 'NONE',  ( 5.330173052271000245, -78.14419244445099366, 9.594439332582000546 ) ) ;
#52463=CARTESIAN_POINT ( 'NONE',  ( -4.724527880064000485, -78.87325255039799288, 8.267358256580001452 ) ) ;
#52468=CIRCLE ( 'NONE', #3450, 1.000000000000000000 ) ;
#52469=CARTESIAN_POINT ( 'NONE',  ( -8.796335266379989193, -78.75208333333333144, -6.760013919724055853 ) ) ;
#52474=VECTOR ( 'NONE', #53437, 1000.000000000000114 ) ;
#52475=CARTESIAN_POINT ( 'NONE',  ( 3.292343003156000147, -79.02013871977898418, -10.43303857396000112 ) ) ;
#52477=CARTESIAN_POINT ( 'NONE',  ( -3.551539514618999860, -80.34199133049699526, -10.51033889552999945 ) ) ;
#52479=ORIENTED_EDGE ( 'NONE', *, *, #27937, .T. ) ;
#52486=CARTESIAN_POINT ( 'NONE',  ( 5.496668217546000434, -80.30272527494601320, -8.073860231047000013 ) ) ;
#52493=DIRECTION ( 'NONE',  ( 0.000000000000000000, 1.000000000000000000, 0.000000000000000000 ) ) ;
#52497=CARTESIAN_POINT ( 'NONE',  ( 8.733346097342675307, -78.82335531160738640, -3.049546898630470348 ) ) ;
#52516=CARTESIAN_POINT ( 'NONE',  ( -3.549595971449000409, -78.17549936685999512, 9.069733410961998032 ) ) ;
#52520=FACE_OUTER_BOUND ( 'NONE', #1350, .T. ) ;
#52524=CARTESIAN_POINT ( 'NONE',  ( 0.3341971779677385679, -79.37780856233311511, -9.519315069472982671 ) ) ;
#52528=CARTESIAN_POINT ( 'NONE',  ( -9.775952618636999603, -79.78297254464997934, -1.505437160947000086 ) ) ;
#52546=CARTESIAN_POINT ( 'NONE',  ( 9.630577183392999174, -78.97287637980998909, 1.628483183780000010 ) ) ;
#52549=ORIENTED_EDGE ( 'NONE', *, *, #267, .T. ) ;
#52556=DIRECTION ( 'NONE',  ( 0.000000000000000000, 1.000000000000000000, 0.000000000000000000 ) ) ;
#52570=CARTESIAN_POINT ( 'NONE',  ( -10.71960490440000058, -78.59592221579498528, 3.466843673432000283 ) ) ;
#52571=CARTESIAN_POINT ( 'NONE',  ( 7.535862037907478772, -77.30086240167952383, -5.364085342277994606 ) ) ;
#52581=CARTESIAN_POINT ( 'NONE',  ( -4.348661115406000199, -79.15007827033099375, -10.27524920185999946 ) ) ;
#52586=CARTESIAN_POINT ( 'NONE',  ( -2.166177946181000902, -80.00000000000000000, 9.033216284371517801 ) ) ;
#52592=LINE ( 'NONE', #39863, #44791 ) ;
#52596=CARTESIAN_POINT ( 'NONE',  ( 4.603815134758999505, -77.24485258715699842, -8.210729597153999748 ) ) ;
#52597=CARTESIAN_POINT ( 'NONE',  ( -11.00000000000000000, -79.19999999999998863, 0.000000000000000000 ) ) ;
#52602=CARTESIAN_POINT ( 'NONE',  ( 2.421167930323313566, -78.85416666666664298, 9.009247259181924150 ) ) ;
#52608=CARTESIAN_POINT ( 'NONE',  ( 2.550499813263000348, -78.51351126778098433, -10.67515654612000020 ) ) ;
#52614=ORIENTED_EDGE ( 'NONE', *, *, #51404, .F. ) ;
#52618=CARTESIAN_POINT ( 'NONE',  ( 7.994753734545000157, -78.49140324543799352, 7.938063182512999916 ) ) ;
#52626=EDGE_CURVE ( 'NONE', #38602, #46260, #36826, .T. ) ;
#52638=CARTESIAN_POINT ( 'NONE',  ( -4.686723500388265684, -79.41694709479033065, 8.065566475210284025 ) ) ;
#52642=CARTESIAN_POINT ( 'NONE',  ( -5.179006628193274508, -77.52228172415060214, 7.668103985437277004 ) ) ;
#52643=CARTESIAN_POINT ( 'NONE',  ( 10.07768261906999996, -78.02607137478699428, -4.508174471003999706 ) ) ;
#52645=CARTESIAN_POINT ( 'NONE',  ( -9.346518596363001308, -77.80847978158598721, 2.610229778083999808 ) ) ;
#52650=CARTESIAN_POINT ( 'NONE',  ( -7.054457466615000172, -80.50123988683198206, -8.769379688592000122 ) ) ;
#52658=B_SPLINE_CURVE_WITH_KNOTS ( 'NONE', 3,
 ( #8151, #3717, #36466, #13440, #18187, #54493, #39725, #44450, #30855, #9323, #45346, #13145, #26428, #27315, #22895, #17590, #26723, #48893 ),
 .UNSPECIFIED., .F., .F.,
 ( 4, 2, 2, 2, 2, 2, 2, 2, 4 ),
 ( 0.000000000000000000, 0.1250000000000000000, 0.2500000000000000000, 0.3750000000000000000, 0.5000000000000000000, 0.6250000000000000000, 0.7500000000000000000, 0.8750000000000000000, 1.000000000000000000 ),
 .UNSPECIFIED. ) ;
#52659=CARTESIAN_POINT ( 'NONE',  ( 7.396983374551519219, -78.40212121928816202, 5.684573788064898103 ) ) ;
#52662=CARTESIAN_POINT ( 'NONE',  ( -5.049388770360000223, -80.08077773488000162, -9.976713590530000175 ) ) ;
#52666=CARTESIAN_POINT ( 'NONE',  ( 10.71369944335147117, -79.97083333333559096, 2.879226727952105769 ) ) ;
#52673=CARTESIAN_POINT ( 'NONE',  ( -2.577533092820055494, -77.20624999999999716, -10.72859319707154668 ) ) ;
#52675=FACE_OUTER_BOUND ( 'NONE', #55733, .T. ) ;
#52677=CIRCLE ( 'NONE', #41379, 1.000000000000000000 ) ;
#52680=CARTESIAN_POINT ( 'NONE',  ( 7.265900323201000433, -77.62487771236999379, 8.333956192971999855 ) ) ;
#52685=CARTESIAN_POINT ( 'NONE',  ( 7.764258067048000811, -77.07068982153518277, 5.767450660628000492 ) ) ;
#52722=CARTESIAN_POINT ( 'NONE',  ( 6.760013919724038978, -78.52291666666666003, 8.796335266380001627 ) ) ;
#52742=CARTESIAN_POINT ( 'NONE',  ( 1.439896632895334649, -79.83541666666666003, -10.99999999999999822 ) ) ;
#52750=CARTESIAN_POINT ( 'NONE',  ( -7.648940337505000464, -77.44503301142398755, -5.852081988952999581 ) ) ;
#52759=CARTESIAN_POINT ( 'NONE',  ( -2.162167942093999873, -78.26164515279698719, 10.72440421974000024 ) ) ;
#52761=CARTESIAN_POINT ( 'NONE',  ( -1.645926171036000030, -80.41978745972699016, -10.69587012110999780 ) ) ;
#52762=EDGE_LOOP ( 'NONE', ( #9904, #53339, #39978, #1447 ) ) ;
#52764=ORIENTED_EDGE ( 'NONE', *, *, #18223, .T. ) ;
#52791=CARTESIAN_POINT ( 'NONE',  ( 11.00000000000000000, -79.84999999999999432, 0.000000000000000000 ) ) ;
#52795=CARTESIAN_POINT ( 'NONE',  ( -9.289856196000998878, -77.44054472353899143, 1.941241007807000152 ) ) ;
#52808=ADVANCED_FACE ( 'NONE', ( #33643 ), #34, .F. ) ;
#52811=CARTESIAN_POINT ( 'NONE',  ( -9.226371719725817044, -79.26948592758979828, -2.305846157194820112 ) ) ;
#52812=CARTESIAN_POINT ( 'NONE',  ( -8.454756037848037309, -79.99999999999997158, -3.909103053904156688 ) ) ;
#52815=CARTESIAN_POINT ( 'NONE',  ( -5.346700182771000343, -80.12992104470397692, 7.765585233270999588 ) ) ;
#52817=CARTESIAN_POINT ( 'NONE',  ( 9.009247259181924150, -79.22916666666665719, -2.421167930323326001 ) ) ;
#52826=CARTESIAN_POINT ( 'NONE',  ( 10.97031909684999995, -77.66693593946899909, -1.702279910903999882 ) ) ;
#52832=B_SPLINE_CURVE_WITH_KNOTS ( 'NONE', 3,
 ( #28919, #37485, #46672, #6784, #46963, #5612, #33637, #51679, #42229, #18911, #29206, #1214, #931, #36904, #54918, #6197, #37197, #1501 ),
 .UNSPECIFIED., .F., .F.,
 ( 4, 2, 2, 2, 2, 2, 2, 2, 4 ),
 ( 0.000000000000000000, 0.1249999999999999167, 0.2499999999999998335, 0.3749999999999998335, 0.4999999999999998890, 0.6249999999999998890, 0.7499999999999998890, 0.8750000000000000000, 1.000000000000000000 ),
 .UNSPECIFIED. ) ;
#52834=VERTEX_POINT ( 'NONE', #27977 ) ;
#52835=VERTEX_POINT ( 'NONE', #32115 ) ;
#52842=AXIS2_PLACEMENT_3D ( 'NONE', #7094, #43116, #11246 ) ;
#52843=CARTESIAN_POINT ( 'NONE',  ( 2.260129142450393758, -78.99361093726523109, -9.437459368857011199 ) ) ;
#52844=AXIS2_PLACEMENT_3D ( 'NONE', #47704, #7234, #25238 ) ;
#52851=CARTESIAN_POINT ( 'NONE',  ( 1.161006248771640159, -79.96550791624770227, 9.176744600133316609 ) ) ;
#52852=CARTESIAN_POINT ( 'NONE',  ( -8.781071604798297514, -80.00280623849064909, -6.803245145519296599 ) ) ;
#52854=CARTESIAN_POINT ( 'NONE',  ( -3.006161377376999955, -79.01730753078498992, 10.85780494109000038 ) ) ;
#52855=CARTESIAN_POINT ( 'NONE',  ( 6.151869538368270440, -77.28303250187612150, -6.911824961258240307 ) ) ;
#52863=CARTESIAN_POINT ( 'NONE',  ( 9.250000000000000000, -77.84999999999999432, 0.000000000000000000 ) ) ;
#52866=CARTESIAN_POINT ( 'NONE',  ( 2.592785862636999727, -78.70060060100799149, -10.85214546196000107 ) ) ;
#52872=CARTESIAN_POINT ( 'NONE',  ( 1.571010256693058382, -77.20000000000000284, 10.69622524930801610 ) ) ;
#52873=B_SPLINE_CURVE_WITH_KNOTS ( 'NONE', 3,
 ( #16833, #30387, #11546, #34237, #34815, #52843, #53132, #12681, #30673, #56412, #15961, #33953, #11826, #29523, #29804, #47858, #22116, #50401, #10534, #32357, #9950, #1111, #27930, #35385, #32644, #19096, #40126, #14649, #31250, #46274, #5224, #39831, #28217, #50983, #32939, #23230, #36798, #35693, #41234, #45980, #54816, #14357, #58139, #55104, #50695, #3826, #53721, #13259, #57843, #41526, #26834, #10238, #17706, #17401, #1394, #28516, #49292, #5798, #45684, #5506, #21826, #55395, #37381, #23515, #4116 ),
 .UNSPECIFIED., .F., .F.,
 ( 4, 1, 1, 1, 1, 1, 1, 1, 1, 1, 1, 1, 1, 1, 1, 1, 1, 1, 1, 1, 1, 1, 1, 1, 1, 1, 1, 1, 1, 1, 1, 1, 1, 1, 1, 1, 1, 1, 1, 1, 1, 1, 1, 1, 1, 1, 1, 1, 1, 1, 1, 1, 1, 1, 1, 1, 1, 1, 1, 1, 1, 1, 4 ),
 ( 1.368866741782499985E-09, 0.01249973857914446311, 0.02874974741936314054, 0.04499975625958181624, 0.06124976509980049194, 0.07749977394001916764, 0.09374978278023785028, 0.1099997916204565329, 0.1262498004606752156, 0.1424998093008938704, 0.1587498181411125531, 0.1749998269813312357, 0.1912498358215499183, 0.2074998446617686010, 0.2237498535019872836, 0.2399998623422059385, 0.2562498711824245934, 0.2724998800226433593, 0.2887498888628620142, 0.3049998977030806691, 0.3212499065432993239, 0.3374999153835180898, 0.3537499242237367447, 0.3699999330639553996, 0.3862499419041740545, 0.4024999507443927649, 0.4187499595846114753, 0.4349999684248301302, 0.4512499772650487850, 0.4674999861052674954, 0.4837499949454861503, 0.5000000037857047497, 0.5162500126259234046, 0.5325000214661420594, 0.5487500303063607143, 0.5650000391465793692, 0.5812500479867981351, 0.5975000568270167900, 0.6137500656672355559, 0.6300000745074542108, 0.6462500833476728657, 0.6625000921878915205, 0.6787501010281101754, 0.6950001098683288303, 0.7112501187085475962, 0.7275001275487662511, 0.7437501363889849060, 0.7600001452292036719, 0.7762501540694223268, 0.7925001629096409816, 0.8087501717498596365, 0.8250001805900781804, 0.8412501894302969463, 0.8575001982705156012, 0.8737502071107342561, 0.8900002159509529109, 0.9062502247911715658, 0.9225002336313903317, 0.9387502424716089866, 0.9550002513118276415, 0.9712502601520462964, 0.9875002689922650623, 1.000000000000000000 ),
 .UNSPECIFIED. ) ;
#52881=CARTESIAN_POINT ( 'NONE',  ( 9.296715471869999803, -78.93591467081699875, -2.514846541900999988 ) ) ;
#52884=B_SPLINE_CURVE_WITH_KNOTS ( 'NONE', 3,
 ( #37916, #55643, #55057, #55941, #50353, #14893, #23182, #6041, #18757, #10483 ),
 .UNSPECIFIED., .F., .F.,
 ( 4, 2, 2, 2, 4 ),
 ( 1.658364595237685148E-07, 0.2500001243773446458, 0.5000000829182297268, 0.7500000414591149189, 1.000000000000000000 ),
 .UNSPECIFIED. ) ;
#52893=CARTESIAN_POINT ( 'NONE',  ( 9.304500756975000897, -79.07535835443499650, -5.821536072646999571 ) ) ;
#52894=CARTESIAN_POINT ( 'NONE',  ( 10.89973958340319449, -80.30026041666515368, 1.427624786073512508 ) ) ;
#52899=CONICAL_SURFACE ( 'NONE', #34960, 1.099999997149000430, 0.7853981633972997312 ) ;
#52901=CARTESIAN_POINT ( 'NONE',  ( 1.476676445040142616, -77.36242827574842806, 9.246657040384873127 ) ) ;
#52903=CARTESIAN_POINT ( 'NONE',  ( -3.607132791900000246, -79.34186490753599230, -10.55841809546000043 ) ) ;
#52905=FACE_OUTER_BOUND ( 'NONE', #46190, .T. ) ;
#52912=CARTESIAN_POINT ( 'NONE',  ( 9.250000000000000000, -79.24999999999998579, 0.000000000000000000 ) ) ;
#52917=ORIENTED_EDGE ( 'NONE', *, *, #2208, .F. ) ;
#52927=CARTESIAN_POINT ( 'NONE',  ( -7.126130270949447620, -77.54504099251572313, 5.897698824246291771 ) ) ;
#52928=CARTESIAN_POINT ( 'NONE',  ( 7.528714304401000312, -77.99426166612198585, -8.074838600060001426 ) ) ;
#52932=CARTESIAN_POINT ( 'NONE',  ( -9.157500079073999544, -78.80331380109998918, 3.211059275314999795 ) ) ;
#52937=CARTESIAN_POINT ( 'NONE',  ( 7.117135278674999732, -80.19036996912898019, 8.718833803912000135 ) ) ;
#52940=CARTESIAN_POINT ( 'NONE',  ( -4.658475568430814562, -78.58333333333332860, -8.082524092276884176 ) ) ;
#52949=CARTESIAN_POINT ( 'NONE',  ( -9.380881115328000064, -79.88761105452199729, 5.414960042740999846 ) ) ;
#52952=CARTESIAN_POINT ( 'NONE',  ( -7.355596411687169045, -79.65251264481355520, -5.642826774240620402 ) ) ;
#52960=CARTESIAN_POINT ( 'NONE',  ( 3.033202772035243910, -77.59806847599675450, -10.38096122863011495 ) ) ;
#52980=AXIS2_PLACEMENT_3D ( 'NONE', #26179, #3744, #21463 ) ;
#52984=DIRECTION ( 'NONE',  ( 0.000000000000000000, 0.7071067811866525998, -0.7071067811864425456 ) ) ;
#52990=VERTEX_POINT ( 'NONE', #46317 ) ;
#53022=AXIS2_PLACEMENT_3D ( 'NONE', #38698, #7694, #34256 ) ;
#53029=FACE_OUTER_BOUND ( 'NONE', #31694, .T. ) ;
#53040=CARTESIAN_POINT ( 'NONE',  ( -8.852983674280999082, -78.98694786691399372, -3.506430706099999739 ) ) ;
#53045=CARTESIAN_POINT ( 'NONE',  ( 9.243118074942941576, -78.85649633572980122, 0.7011782411833578088 ) ) ;
#53048=CARTESIAN_POINT ( 'NONE',  ( 4.007494466573000125, -79.89653890021898519, -10.71665855536000223 ) ) ;
#53056=CARTESIAN_POINT ( 'NONE',  ( 1.739862777674999972, -79.61076166194752091, 9.611119481339999382 ) ) ;
#53060=VERTEX_POINT ( 'NONE', #1442 ) ;
#53068=CARTESIAN_POINT ( 'NONE',  ( 10.36935812844000004, -78.07876026662599145, -2.835297515976000327 ) ) ;
#53072=CARTESIAN_POINT ( 'NONE',  ( 8.496400742388793503, -78.81780298388180483, -3.659025731067179876 ) ) ;
#53073=DIRECTION ( 'NONE',  ( 0.000000000000000000, -1.000000000000000000, 0.000000000000000000 ) ) ;
#53084=CARTESIAN_POINT ( 'NONE',  ( 9.380731069130998634, -77.26943616160899353, -0.1623923911645999696 ) ) ;
#53092=DIRECTION ( 'NONE',  ( 0.000000000000000000, -1.000000000000000000, 0.000000000000000000 ) ) ;
#53096=ORIENTED_EDGE ( 'NONE', *, *, #6348, .T. ) ;
#53100=CARTESIAN_POINT ( 'NONE',  ( 8.982046426857383636, -79.02685948540812433, 3.153244770633860217 ) ) ;
#53103=CARTESIAN_POINT ( 'NONE',  ( -11.00000000000000888, -79.08958333333330870, 1.439896632895276252 ) ) ;
#53105=CARTESIAN_POINT ( 'NONE',  ( -9.692328422619000960, -79.19622958825499381, 1.312170392071000169 ) ) ;
#53108=ORIENTED_EDGE ( 'NONE', *, *, #5184, .T. ) ;
#53124=CARTESIAN_POINT ( 'NONE',  ( 9.767191983224998708, -79.52026917934998096, 0.05162932631433000269 ) ) ;
#53132=CARTESIAN_POINT ( 'NONE',  ( -1.182210496605485606, -78.96518710813624864, -9.632040656990779937 ) ) ;
#53139=CARTESIAN_POINT ( 'NONE',  ( 3.505028940034645046, -79.94415934739535601, 8.560182507365089677 ) ) ;
#53143=CARTESIAN_POINT ( 'NONE',  ( -3.770495512267000304, -79.52296990877398741, 10.61660482251999937 ) ) ;
#53144=CARTESIAN_POINT ( 'NONE',  ( -1.431006885156403508, -77.21271974587020281, -9.151478666840258569 ) ) ;
#53152=CARTESIAN_POINT ( 'NONE',  ( -3.321932689531000182, -80.44999999999998863, -10.22385755016999909 ) ) ;
#53153=CARTESIAN_POINT ( 'NONE',  ( -11.14855507251999889, -78.56013882934497872, -0.4486863643567999826 ) ) ;
#53157=ORIENTED_EDGE ( 'NONE', *, *, #21166, .T. ) ;
#53159=EDGE_CURVE ( 'NONE', #35609, #40455, #41530, .T. ) ;
#53170=VERTEX_POINT ( 'NONE', #5073 ) ;
#53176=CARTESIAN_POINT ( 'NONE',  ( -7.604423127187000198, -79.86606249275499181, 7.914351627518998455 ) ) ;
#53177=ADVANCED_FACE ( 'NONE', ( #54664 ), #23940, .T. ) ;
#53187=CONICAL_SURFACE ( 'NONE', #19276, 1.099999997149000430, 0.7853981633972997312 ) ;
#53189=CARTESIAN_POINT ( 'NONE',  ( -4.348661115406000199, -78.83620252954798957, -10.27524920185999946 ) ) ;
#53202=CARTESIAN_POINT ( 'NONE',  ( -9.067527500126635331, -79.72528127043524648, 2.911084842785973681 ) ) ;
#53208=CARTESIAN_POINT ( 'NONE',  ( -9.121286397524418277, -78.11412521488340133, -1.606255959880608319 ) ) ;
#53213=CARTESIAN_POINT ( 'NONE',  ( -6.342524396040097656, -77.53526462310868794, 6.737273603580285375 ) ) ;
#53214=CARTESIAN_POINT ( 'NONE',  ( -3.203604947276999848, -77.70797428813398255, 10.56508708803000118 ) ) ;
#53216=CARTESIAN_POINT ( 'NONE',  ( -0.1538805260929999863, -78.26671631506198423, 9.702939253146000809 ) ) ;
#53220=CARTESIAN_POINT ( 'NONE',  ( -3.493617039247999934, -80.40847481238299110, -10.33892454317000187 ) ) ;
#53230=CARTESIAN_POINT ( 'NONE',  ( 0.6054113949338107981, -78.46981924737423242, 9.249594591320265735 ) ) ;
#53251=AXIS2_PLACEMENT_3D ( 'NONE', #1001, #18986, #46159 ) ;
#53256=CARTESIAN_POINT ( 'NONE',  ( 9.670530767802999250, -77.01847108759879745, -0.1674091926992999912 ) ) ;
#53290=DIRECTION ( 'NONE',  ( 0.000000000000000000, -1.000000000000000000, 0.000000000000000000 ) ) ;
#53299=CARTESIAN_POINT ( 'NONE',  ( -8.736253822433678096, -78.62667298105303360, -3.039731260859822370 ) ) ;
#53319=CARTESIAN_POINT ( 'NONE',  ( 9.322139347623476624, -76.97083333334067845, -1.984632901571217412 ) ) ;
#53322=CARTESIAN_POINT ( 'NONE',  ( 2.192362874646999860, -79.16451892421298453, -9.154492618432000128 ) ) ;
#53332=CARTESIAN_POINT ( 'NONE',  ( -9.937637090044999510, -79.77094125464398644, 4.829168387547000840 ) ) ;
#53335=CARTESIAN_POINT ( 'NONE',  ( -10.52185994994999874, -79.89900688576899768, -3.892032218524000164 ) ) ;
#53338=CONICAL_SURFACE ( 'NONE', #55242, 10.84999999997999964, 0.7853981633972997312 ) ;
#53339=ORIENTED_EDGE ( 'NONE', *, *, #27593, .T. ) ;
#53340=CIRCLE ( 'NONE', #35405, 4.799999999999999822 ) ;
#53356=CARTESIAN_POINT ( 'NONE',  ( 9.143727524999398781, -78.83803687086303569, -1.399743652968158836 ) ) ;
#53363=CARTESIAN_POINT ( 'NONE',  ( -8.084233020759592492, -80.04022715548097722, 7.554717540679545706 ) ) ;
#53368=CARTESIAN_POINT ( 'NONE',  ( 0.000000000000000000, -78.69999999999998863, 0.000000000000000000 ) ) ;
#53371=CIRCLE ( 'NONE', #35450, 5.000000000000000000 ) ;
#53387=CARTESIAN_POINT ( 'NONE',  ( 9.354045381180000618, -79.98053041167199240, 2.857433141267999854 ) ) ;
#53391=DIRECTION ( 'NONE',  ( 0.000000000000000000, 0.000000000000000000, -1.000000000000000000 ) ) ;
#53403=CARTESIAN_POINT ( 'NONE',  ( 8.249323304235000265, -79.97488639496098983, -5.229696851825000437 ) ) ;
#53404=ORIENTED_EDGE ( 'NONE', *, *, #23023, .T. ) ;
#53423=CARTESIAN_POINT ( 'NONE',  ( -1.719802448987169274, -79.99009311709434655, 9.096255206201579568 ) ) ;
#53428=CARTESIAN_POINT ( 'NONE',  ( 6.245083526999000156, -78.79256869612397907, -9.376985981987999708 ) ) ;
#53429=CARTESIAN_POINT ( 'NONE',  ( 3.003484176522146054, -77.25148415549074343, -8.748772631339541306 ) ) ;
#53437=DIRECTION ( 'NONE',  ( -0.7071067811865470176, -0.7071067811865470176, -3.680441369915245526E-08 ) ) ;
#53438=CARTESIAN_POINT ( 'NONE',  ( -7.632977269198000236, -79.12198591599799613, -8.138136006783000198 ) ) ;
#53449=CARTESIAN_POINT ( 'NONE',  ( -9.326074664721659246, -79.95762289869909978, 5.512178488021413969 ) ) ;
#53453=CARTESIAN_POINT ( 'NONE',  ( -9.628933692773001596, -78.70852403778498285, -0.1919528651714999812 ) ) ;
#53464=CARTESIAN_POINT ( 'NONE',  ( -10.79326785783000098, -79.44467717776498716, -1.992331681952000055 ) ) ;
#53465=CARTESIAN_POINT ( 'NONE',  ( -6.634986530482820832, -80.40442708333218036, 8.632259101794380385 ) ) ;
#53474=DIRECTION ( 'NONE',  ( -1.000000000000000000, 0.000000000000000000, 0.000000000000000000 ) ) ;
#53477=CARTESIAN_POINT ( 'NONE',  ( 6.722579162784999340, -79.56660374219698895, 8.904972230874999894 ) ) ;
#53488=DIRECTION ( 'NONE',  ( 0.000000000000000000, 1.000000000000000000, 0.000000000000000000 ) ) ;
#53489=ADVANCED_FACE ( 'NONE', ( #27644 ), #49522, .T. ) ;
#53494=B_SPLINE_CURVE_WITH_KNOTS ( 'NONE', 3,
 ( #44241, #12368, #8811, #39800, #30645, #26803, #9112, #7934, #39518, #43961, #48680, #25935, #3511, #21512, #57523, #35066, #53103, #8224 ),
 .UNSPECIFIED., .F., .F.,
 ( 4, 2, 2, 2, 2, 2, 2, 2, 4 ),
 ( 0.000000000000000000, 0.1249999999999999445, 0.2499999999999998890, 0.3749999999999999445, 0.5000000000000000000, 0.6250000000000000000, 0.7500000000000001110, 0.8750000000000000000, 1.000000000000000000 ),
 .UNSPECIFIED. ) ;
#53501=ORIENTED_EDGE ( 'NONE', *, *, #27937, .F. ) ;
#53502=CARTESIAN_POINT ( 'NONE',  ( -1.866732844877771580, -77.49119273318581236, 9.060374038664914309 ) ) ;
#53503=CARTESIAN_POINT ( 'NONE',  ( 10.71768947918000059, -78.04727784723098694, -1.656903943290000125 ) ) ;
#53506=AXIS2_PLACEMENT_3D ( 'NONE', #6324, #28747, #24341 ) ;
#53507=CARTESIAN_POINT ( 'NONE',  ( -7.707166124622999881, -77.38212234465098049, -5.896629607976000109 ) ) ;
#53511=CARTESIAN_POINT ( 'NONE',  ( -4.017143116098000455, -80.33419522547698932, 10.51352533724000082 ) ) ;
#53514=CARTESIAN_POINT ( 'NONE',  ( -1.210822168571057400, -78.61458333333332860, -9.250000000000001776 ) ) ;
#53531=ORIENTED_EDGE ( 'NONE', *, *, #5120, .F. ) ;
#53537=CARTESIAN_POINT ( 'NONE',  ( -4.692196280270000130, -79.60434362032799527, -8.173708953481000350 ) ) ;
#53548=B_SPLINE_SURFACE_WITH_KNOTS ( 'NONE', 3, 3, ( 
 ( #24814, #43119, #51700, #30378, #34228, #48417, #29795, #47277, #47571, #42829, #30083, #56404, #2679, #16826, #3252, #38960, #33944, #52264, #43697, #20673, #42539, #47850, #7380, #25381, #21242, #43396, #2958, #20106, #34515, #34808, #56973, #16535, #52546, #31542, #35378 ),
 ( #49587, #54009, #35090, #53403, #57836, #17103, #44854, #12673, #44262, #35684, #58130, #17694, #26246, #49284, #4106, #22108, #13, #53124, #12951, #30664, #48701, #40117, #45159, #57544, #13842, #53712, #39822, #44554, #3817, #49883, #36284, #13249, #31242, #8244, #21819 ),
 ( #30949, #26527, #43978, #48988, #40421, #8533, #8835, #17393, #26824, #54306, #4406, #22408, #13550, #31840, #17992, #35984, #312, #9134, #40720, #27118, #4708, #39538, #25955, #22706, #3530, #18290, #21533, #54874, #18583, #37445, #4995, #50465, #42182, #28584, #46334 ),
 ( #15011, #18868, #14424, #1751, #5860, #37154, #10017, #27995, #32418, #46043, #55169, #55764, #55463, #14132, #33004, #51051, #50761, #5568, #10306, #10599, #46627, #36572, #27417, #6158, #9717, #24166, #37741, #19746, #14711, #45452, #23576, #32709, #27705, #41592, #15310 ),
 ( #9428, #1172, #41300, #19161, #28285, #23869, #41883, #33303, #22999, #1461, #19451, #41011, #603, #50172, #54596, #32131, #45751, #5284, #23292, #884, #36861, #11756, #38033, #11189, #2614, #25033, #43053, #51635, #16185, #29448, #47506, #25320, #42475, #38319, #2044 ),
 ( #34164, #56339, #7032, #20045, #52486, #29165, #15892, #16472, #29735, #56053, #12042, #43336, #38895, #38611, #20610, #52201, #56626, #47785, #7316, #15602, #33878, #56916, #3190, #21178, #48077, #2893, #20890, #10898, #34454, #33596, #47212, #28874, #25605, #30022, #7605 ),
 ( #6447, #39181, #43628, #57196, #16764, #6741, #51917, #24752, #51339, #46920, #11477, #24463, #42768, #2327, #20323, #30890, #22339, #44203, #22642, #35312, #12609, #3465, #40354, #17326, #30604, #45087, #26756, #13479, #39757, #53056, #4338, #58363, #3753, #9066, #17042 ) ),
 .UNSPECIFIED., .F., .F., .F.,
 ( 4, 3, 4 ),
 ( 4, 1, 1, 1, 1, 1, 1, 1, 1, 1, 1, 1, 1, 1, 1, 1, 1, 1, 1, 1, 1, 1, 1, 1, 1, 1, 1, 1, 1, 1, 1, 1, 4 ),
 ( -0.4045438850609999748, 1.404543885061000141, 5.000129188560400451 ),
 ( 0.4173531076193000011, 0.4359178370333999797, 0.4544825664474999583, 0.4730472958615999923, 0.4916120252757000264, 0.5101767546897999495, 0.5287414841038999835, 0.5473062135180000176, 0.5658709429320999407, 0.5844356723461999747, 0.6030004017601999777, 0.6215651311743000118, 0.6401298605884000459, 0.6586945900024999689, 0.6772593194166000030, 0.6958240488306999261, 0.7143887782447999601, 0.7329535076588999942, 0.7515182370730000283, 0.7700829664870000313, 0.7886476959010999543, 0.8072124253151999884, 0.8257771547292999115, 0.8443418841433999456, 0.8629066135575000906, 0.8814713429716000137, 0.9000360723857000478, 0.9186008017997999708, 0.9371655312139000049, 0.9557302606279000079, 0.9742949900419999310, 0.9928597194561000761, 1.011424448870000159 ),
 .UNSPECIFIED. ) ;
#53560=CARTESIAN_POINT ( 'NONE',  ( -10.99999999999000089, -80.20000000002698926, -2.639066790267999940E-09 ) ) ;
#53568=( NAMED_UNIT ( * ) PLANE_ANGLE_UNIT ( ) SI_UNIT ( $, .RADIAN. ) );
#53574=B_SPLINE_CURVE_WITH_KNOTS ( 'NONE', 3,
 ( #17302, #48902, #48614, #9334 ),
 .UNSPECIFIED., .F., .F.,
 ( 4, 4 ),
 ( 0.000000000000000000, 1.000000000000000000 ),
 .UNSPECIFIED. ) ;
#53578=CARTESIAN_POINT ( 'NONE',  ( 5.341789944771998755, -77.68480993295618475, 9.661750877468000098 ) ) ;
#53585=CARTESIAN_POINT ( 'NONE',  ( 7.658860137760000519, -78.51216497498398894, 5.959242465009999989 ) ) ;
#53591=CARTESIAN_POINT ( 'NONE',  ( -9.119748668238788269, -78.61353292670899862, -1.546334858068346696 ) ) ;
#53618=CARTESIAN_POINT ( 'NONE',  ( -9.446372167179999835, -78.44689511346298616, 1.198511206093999970 ) ) ;
#53632=DIRECTION ( 'NONE',  ( 0.000000000000000000, 1.000000000000000000, 0.000000000000000000 ) ) ;
#53644=CARTESIAN_POINT ( 'NONE',  ( 8.083247094228855900, -79.30839652358213243, -4.658693541334342214 ) ) ;
#53661=DIRECTION ( 'NONE',  ( 0.000000000000000000, 1.000000000000000000, 0.000000000000000000 ) ) ;
#53670=DIRECTION ( 'NONE',  ( 0.000000000000000000, -1.000000000000000000, 0.000000000000000000 ) ) ;
#53676=LINE ( 'NONE', #22378, #17565 ) ;
#53682=B_SPLINE_CURVE_WITH_KNOTS ( 'NONE', 3,
 ( #21739, #21164, #39745, #34439, #25879, #35597, #57755, #58049, #12594, #57181, #16746, #38881, #17312, #52469, #7593, #57468, #3451, #47771 ),
 .UNSPECIFIED., .F., .F.,
 ( 4, 2, 2, 2, 2, 2, 2, 2, 4 ),
 ( 0.000000000000000000, 0.1249999999999999722, 0.2499999999999999445, 0.3750000000000000000, 0.5000000000000001110, 0.6250000000000001110, 0.7500000000000000000, 0.8750000000000000000, 1.000000000000000000 ),
 .UNSPECIFIED. ) ;
#53689=CARTESIAN_POINT ( 'NONE',  ( -1.186507705731999929, -78.94446787273398058, -9.667052097962999468 ) ) ;
#53697=CIRCLE ( 'NONE', #4695, 1.199999999999999956 ) ;
#53700=ADVANCED_FACE ( 'NONE', ( #43865 ), #12267, .T. ) ;
#53712=CARTESIAN_POINT ( 'NONE',  ( -9.699833017908000343, -79.26048791328599918, 1.146274062705999963 ) ) ;
#53716=DIRECTION ( 'NONE',  ( -1.000000000000000000, 0.000000000000000000, 0.000000000000000000 ) ) ;
#53721=CARTESIAN_POINT ( 'NONE',  ( -9.346673348102125800, -77.82823394297724917, 2.610272996057591666 ) ) ;
#53728=CARTESIAN_POINT ( 'NONE',  ( 7.033303429947452834, -79.90635737682303841, 6.007822180714758709 ) ) ;
#53735=B_SPLINE_SURFACE_WITH_KNOTS ( 'NONE', 3, 3, ( 
 ( #37730, #11467, #46618, #5851, #6438, #23857, #15298, #41873, #20032, #33292, #51330, #19444, #55453, #10887, #28863, #24452, #42466, #2032, #34444 ),
 ( #56908, #44477, #43618, #58057, #17035, #25311, #53048, #22034, #12601, #40040, #3181, #20883, #30598, #48630, #26454, #21747, #48069, #52477, #8457 ),
 ( #12035, #30883, #52193, #48918, #39751, #35305, #7598, #57474, #47778, #34733, #4027, #12882, #11748, #8178, #25598, #2887, #21171, #17616, #52761 ),
 ( #12318, #29727, #7309, #53335, #43329, #44197, #38887, #57187, #30013, #57762, #17319, #39175, #16753, #16463, #30304, #48345, #25885, #7884, #43913 ) ),
 .UNSPECIFIED., .F., .F., .F.,
 ( 4, 4 ),
 ( 4, 1, 1, 1, 1, 1, 1, 1, 1, 1, 1, 1, 1, 1, 1, 1, 4 ),
 ( -0.1387574078320999993, 1.138757407831999968 ),
 ( -0.007432834721512999662, 0.01672387812341000202, 0.04088059096832000194, 0.06503730381324000775, 0.08919401665815999969, 0.1133507295031000034, 0.1375074423479999974, 0.1616641551929000054, 0.1858208680378000133, 0.2099775808827999968, 0.2341342937277000047, 0.2582910065726000126, 0.2824477194174999650, 0.3066044322623999729, 0.3307611451072999809, 0.3549178579523000199, 0.3790745707971999723 ),
 .UNSPECIFIED. ) ;
#53741=CARTESIAN_POINT ( 'NONE',  ( -5.068180973607000261, -78.64441589234299101, -9.940077528656999561 ) ) ;
#53755=CARTESIAN_POINT ( 'NONE',  ( 8.881263526186000234, -77.42242364445598923, 3.434171575746000293 ) ) ;
#53766=B_SPLINE_CURVE_WITH_KNOTS ( 'NONE', 3,
 ( #32380, #1423, #45117, #22668, #271, #41260, #40679, #18830, #50424, #9974, #7502, #28542, #6409, #46590, #48252, #14968, #2006, #52952, #39374, #57087, #15267, #25789, #28831, #24424 ),
 .UNSPECIFIED., .F., .F.,
 ( 4, 2, 1, 2, 2, 2, 2, 2, 2, 2, 1, 2, 4 ),
 ( 0.000000000000000000, 0.06249999999999994449, 0.1249999999999999167, 0.1874999999999998890, 0.2499999999999998890, 0.3749999999999998890, 0.4999999999999998890, 0.6249999999999998890, 0.7499999999999998890, 0.8124999999999998890, 0.8750000000000000000, 0.9375000000000000000, 1.000000000000000000 ),
 .UNSPECIFIED. ) ;
#53767=CARTESIAN_POINT ( 'NONE',  ( -9.813193589766999736, -78.96710715410898729, -4.915816122623000162 ) ) ;
#53772=ORIENTED_EDGE ( 'NONE', *, *, #4707, .T. ) ;
#53774=CARTESIAN_POINT ( 'NONE',  ( 9.278548426423457229, -77.24995839143393539, 0.001488306988104594027 ) ) ;
#53779=CARTESIAN_POINT ( 'NONE',  ( 11.12554012740000076, -78.49909427755598301, 0.8449594846185999319 ) ) ;
#53788=EDGE_LOOP ( 'NONE', ( #51148, #18213, #24393, #30085, #42654 ) ) ;
#53792=EDGE_LOOP ( 'NONE', ( #34438, #48921, #2045, #9481 ) ) ;
#53797=CARTESIAN_POINT ( 'NONE',  ( -1.210822168571057400, -79.61458333333335702, -9.250000000000001776 ) ) ;
#53799=CARTESIAN_POINT ( 'NONE',  ( -3.859218140372036032, -78.19092744093191527, -8.411749044435275380 ) ) ;
#53804=CARTESIAN_POINT ( 'NONE',  ( 2.848152166355370163, -77.45027005925211938, 8.800485350458805200 ) ) ;
#53805=CARTESIAN_POINT ( 'NONE',  ( 10.71768947918000059, -78.16788369857198404, -1.656903943290000125 ) ) ;
#53807=CARTESIAN_POINT ( 'NONE',  ( -1.182190922889000184, -79.00573587241498785, -9.631881180458998770 ) ) ;
#53830=CARTESIAN_POINT ( 'NONE',  ( -11.00000000000000711, -80.18958333335920940, 1.439896632895276696 ) ) ;
#53838=CARTESIAN_POINT ( 'NONE',  ( -3.467202887606000150, -79.92579286116600201, 8.763830676697999422 ) ) ;
#53848=EDGE_CURVE ( 'NONE', #43630, #32566, #40800, .T. ) ;
#53859=EDGE_LOOP ( 'NONE', ( #15535, #29317, #51778, #55529, #34886 ) ) ;
#53861=CARTESIAN_POINT ( 'NONE',  ( 5.539808784079903958, -79.43333333333332291, 9.611650271896833075 ) ) ;
#53870=ORIENTED_EDGE ( 'NONE', *, *, #54792, .F. ) ;
#53880=CARTESIAN_POINT ( 'NONE',  ( -0.5413127449341000874, -77.97109731094417384, -11.02683867434999776 ) ) ;
#53888=CARTESIAN_POINT ( 'NONE',  ( -9.446433787353997857, -78.22792668369498870, -2.221620594898999990 ) ) ;
#53901=LINE ( 'NONE', #9024, #12722 ) ;
#53910=EDGE_CURVE ( 'NONE', #24152, #31999, #24710, .T. ) ;
#53919=CARTESIAN_POINT ( 'NONE',  ( -10.35570946080999910, -77.21152914414997781, -4.457041641201000104 ) ) ;
#53923=CARTESIAN_POINT ( 'NONE',  ( 9.372653703366999878, -79.27821424072898537, 0.8742135494153999709 ) ) ;
#53941=ORIENTED_EDGE ( 'NONE', *, *, #17541, .F. ) ;
#53954=AXIS2_PLACEMENT_3D ( 'NONE', #47186, #42451, #20017 ) ;
#53957=CARTESIAN_POINT ( 'NONE',  ( 6.720086853208802502, -78.78986668635583612, -6.356536187194287812 ) ) ;
#53959=CARTESIAN_POINT ( 'NONE',  ( 9.611650271896820641, -78.39166666666665151, 5.539808784079911952 ) ) ;
#53987=CARTESIAN_POINT ( 'NONE',  ( -9.190938788893999956, -78.80234872708999205, 3.222784492720999872 ) ) ;
#53990=CARTESIAN_POINT ( 'NONE',  ( 9.167980031031000010, -78.99867172123299497, -2.618862957269000091 ) ) ;
#54006=EDGE_CURVE ( 'NONE', #14347, #4408, #38690, .T. ) ;
#54008=AXIS2_PLACEMENT_3D ( 'NONE', #48541, #57392, #20517 ) ;
#54009=CARTESIAN_POINT ( 'NONE',  ( 9.523132023602000729, -80.02900749205798547, 1.108936319727999997 ) ) ;
#54021=CARTESIAN_POINT ( 'NONE',  ( -9.346518596363001308, -77.72832879406675488, 2.610229778083999808 ) ) ;
#54022=CARTESIAN_POINT ( 'NONE',  ( 5.434563164594669260, -79.92550071562423852, 7.484833654678077153 ) ) ;
#54023=CARTESIAN_POINT ( 'NONE',  ( 11.00000000000000000, -78.44999999999998863, 0.000000000000000000 ) ) ;
#54035=CARTESIAN_POINT ( 'NONE',  ( 8.429898053969001381, -78.31499867246799340, -7.120476661986999467 ) ) ;
#54060=CARTESIAN_POINT ( 'NONE',  ( -10.65673661723999999, -78.91092244544400103, 2.626400817186000047 ) ) ;
#54061=PLANE ( 'NONE',  #14735 ) ;
#54068=CARTESIAN_POINT ( 'NONE',  ( -7.582587422050910853, -77.44990485243668843, 5.494244969997139627 ) ) ;
#54072=CARTESIAN_POINT ( 'NONE',  ( -10.20553722967999910, -78.33823118367698157, -4.233781229625999565 ) ) ;
#54092=CARTESIAN_POINT ( 'NONE',  ( -3.451502316031555662, -78.19470348729451814, -8.581920319061078217 ) ) ;
#54097=CARTESIAN_POINT ( 'NONE',  ( 0.8199666693160626574, -77.46800884939443677, 9.216836058761973760 ) ) ;
#54098=CARTESIAN_POINT ( 'NONE',  ( -10.47078769031000078, -77.95581897413698869, -3.499536356729999742 ) ) ;
#54099=CARTESIAN_POINT ( 'NONE',  ( -3.907230163516999699, -77.98247802377198923, -8.882807090995999744 ) ) ;
#54103=CARTESIAN_POINT ( 'NONE',  ( -11.00000000000000000, -78.19999999999998863, 0.000000000000000000 ) ) ;
#54104=CARTESIAN_POINT ( 'NONE',  ( -9.062201444876000878, -78.88186501710097787, 6.128973919716999674 ) ) ;
#54107=CARTESIAN_POINT ( 'NONE',  ( -7.396918292183162436, -78.55208333333332860, -5.684557159767966716 ) ) ;
#54118=CARTESIAN_POINT ( 'NONE',  ( -5.148735870932999781, -80.20852921644699052, -10.17300617436000110 ) ) ;
#54128=CARTESIAN_POINT ( 'NONE',  ( 10.97550047727999889, -78.05991538145298136, 0.05101033830554000531 ) ) ;
#54136=CYLINDRICAL_SURFACE ( 'NONE', #3706, 2.600000000000000089 ) ;
#54144=CARTESIAN_POINT ( 'NONE',  ( -2.169167664939000151, -78.24083109332160291, 10.75912301088999889 ) ) ;
#54150=CARTESIAN_POINT ( 'NONE',  ( -8.796335266379998075, -79.54791666666665151, 6.760013919724039866 ) ) ;
#54161=DIRECTION ( 'NONE',  ( -1.000000000000000000, 0.000000000000000000, 0.000000000000000000 ) ) ;
#54164=EDGE_CURVE ( 'NONE', #7174, #25733, #7028, .T. ) ;
#54168=CARTESIAN_POINT ( 'NONE',  ( -4.789974786805000662, -77.93928760227905173, -9.946872946892002076 ) ) ;
#54178=CARTESIAN_POINT ( 'NONE',  ( 9.131029190779001325, -77.43205946808298279, -3.285576857342999979 ) ) ;
#54192=DIRECTION ( 'NONE',  ( 0.000000000000000000, -1.000000000000000000, 0.000000000000000000 ) ) ;
#54201=CARTESIAN_POINT ( 'NONE',  ( -1.882840341529000039, -79.93872424662198739, -9.567914882252001263 ) ) ;
#54202=B_SPLINE_CURVE_WITH_KNOTS ( 'NONE', 3,
 ( #9682, #27670, #45716, #43242, #19938, #6642, #7221, #20515, #10792, #2800, #34067, #25223, #29353, #47400, #24935, #38221, #38512, #15792, #24362 ),
 .UNSPECIFIED., .F., .F.,
 ( 4, 1, 1, 1, 1, 1, 1, 1, 1, 1, 1, 1, 1, 1, 1, 1, 4 ),
 ( 0.5000000000000000000, 0.5324999662279407131, 0.5649999184674565633, 0.5974998707067776804, 0.6299998229462931976, 0.6624997751858089368, 0.6949997274251300539, 0.7274996796646455710, 0.7599996319041613102, 0.7924995841434823163, 0.8249995363829980555, 0.8574994886225137947, 0.8899994408618348007, 0.9224993931013505399, 0.9549993453408660571, 0.9874992975801872852, 1.000000000000000000 ),
 .UNSPECIFIED. ) ;
#54212=CARTESIAN_POINT ( 'NONE',  ( 7.267019124662000173, -77.65102789785198922, -6.153113788875000267 ) ) ;
#54217=ORIENTED_EDGE ( 'NONE', *, *, #20617, .F. ) ;
#54218=EDGE_CURVE ( 'NONE', #18403, #5025, #17121, .T. ) ;
#54228=VERTEX_POINT ( 'NONE', #13565 ) ;
#54233=LINE ( 'NONE', #19381, #4430 ) ;
#54234=AXIS2_PLACEMENT_3D ( 'NONE', #19642, #46824, #1077 ) ;
#54235=EDGE_LOOP ( 'NONE', ( #57352, #48721, #52549, #28869 ) ) ;
#54237=ORIENTED_EDGE ( 'NONE', *, *, #12772, .T. ) ;
#54238=ADVANCED_FACE ( 'NONE', ( #30967 ), #31555, .F. ) ;
#54241=DIRECTION ( 'NONE',  ( -1.000000000000000000, 0.000000000000000000, 0.000000000000000000 ) ) ;
#54249=CARTESIAN_POINT ( 'NONE',  ( 7.692184310832279159, -78.80316060324501848, -5.137369332712866665 ) ) ;
#54251=CARTESIAN_POINT ( 'NONE',  ( 0.000000000000000000, -80.99999999999998579, 7.000000000000000000 ) ) ;
#54261=DIRECTION ( 'NONE',  ( 1.000000000000000000, 0.000000000000000000, 0.000000000000000000 ) ) ;
#54268=LINE ( 'NONE', #30916, #35132 ) ;
#54270=CARTESIAN_POINT ( 'NONE',  ( 1.735064171737695782, -77.31256701792597141, 10.69912951762188058 ) ) ;
#54285=CARTESIAN_POINT ( 'NONE',  ( -8.102939992022999860, -78.37599129015498534, -5.403892966383000207 ) ) ;
#54289=CYLINDRICAL_SURFACE ( 'NONE', #35722, 9.250000000000000000 ) ;
#54298=CARTESIAN_POINT ( 'NONE',  ( 9.468749999988999022, -76.98125000001098783, 2.084568677130999610E-09 ) ) ;
#54300=CARTESIAN_POINT ( 'NONE',  ( -11.18554731360999988, -77.98760464090999278, 0.7683190734677000089 ) ) ;
#54306=CARTESIAN_POINT ( 'NONE',  ( -9.687172913667000174, -79.84035337108399233, -1.248753675804000096 ) ) ;
#54317=CARTESIAN_POINT ( 'NONE',  ( -8.073459667400001649, -78.29680537664623330, -5.384232384047000330 ) ) ;
#54318=CARTESIAN_POINT ( 'NONE',  ( 5.432842449218323821, -79.92551948836533882, 7.486082547988446301 ) ) ;
#54327=CARTESIAN_POINT ( 'NONE',  ( -8.200000000000001066, -80.99999999999998579, 0.000000000000000000 ) ) ;
#54330=CARTESIAN_POINT ( 'NONE',  ( -5.407950800683633652, -80.45000000000000284, -9.358624512082498015 ) ) ;
#54335=CIRCLE ( 'NONE', #24288, 9.549999999999998934 ) ;
#54344=CARTESIAN_POINT ( 'NONE',  ( -9.737659524074000927, -78.77239977856800124, -0.1941203154314999901 ) ) ;
#54353=CARTESIAN_POINT ( 'NONE',  ( -2.928603948516999900, -78.82664538244598873, 10.57767911662999971 ) ) ;
#54364=EDGE_CURVE ( 'NONE', #55354, #49432, #31563, .T. ) ;
#54366=CARTESIAN_POINT ( 'NONE',  ( -9.878709405926999310, -78.84389356166599327, -4.948635581693999974 ) ) ;
#54371=CARTESIAN_POINT ( 'NONE',  ( 4.658475568430798575, -79.83333333333332860, 8.082524092276898386 ) ) ;
#54377=VECTOR ( 'NONE', #39370, 1000.000000000000114 ) ;
#54382=ORIENTED_EDGE ( 'NONE', *, *, #51415, .F. ) ;
#54387=CARTESIAN_POINT ( 'NONE',  ( -5.852226986938722675, -78.17054011490029097, -7.163326417538566915 ) ) ;
#54393=CARTESIAN_POINT ( 'NONE',  ( 1.477687684953830294, -77.46224935051826321, 9.131248644580814755 ) ) ;
#54394=CARTESIAN_POINT ( 'NONE',  ( -8.283402485401001769, -77.92732575713098697, -7.298588567667000149 ) ) ;
#54396=CARTESIAN_POINT ( 'NONE',  ( -5.681372509047000641, -78.46568311896498926, -7.867192369580999767 ) ) ;
#54400=DIRECTION ( 'NONE',  ( 0.000000000000000000, -1.000000000000000000, 0.000000000000000000 ) ) ;
#54401=CARTESIAN_POINT ( 'NONE',  ( -5.736605348686000028, -78.34811028477999173, 9.315534093342000332 ) ) ;
#54413=DIRECTION ( 'NONE',  ( 0.000000000000000000, 1.000000000000000000, 0.000000000000000000 ) ) ;
#54416=CARTESIAN_POINT ( 'NONE',  ( -10.93228849373000067, -80.63166320050999047, -1.499812449630000044 ) ) ;
#54423=CARTESIAN_POINT ( 'NONE',  ( -2.455355393798975605, -77.07239583334455801, 9.133204103152696263 ) ) ;
#54430=CARTESIAN_POINT ( 'NONE',  ( 10.57463602294768812, -77.20000000000000284, 2.242172298085619353 ) ) ;
#54441=CARTESIAN_POINT ( 'NONE',  ( -3.831287612370999796, -76.98242073713129230, -8.693171758988999187 ) ) ;
#54455=ORIENTED_EDGE ( 'NONE', *, *, #39188, .F. ) ;
#54465=VERTEX_POINT ( 'NONE', #3764 ) ;
#54466=VERTEX_POINT ( 'NONE', #44798 ) ;
#54472=CARTESIAN_POINT ( 'NONE',  ( -1.182190922889000184, -78.82482709540299481, -9.631881180458998770 ) ) ;
#54489=CARTESIAN_POINT ( 'NONE',  ( 7.177850223112891115, -77.20000000000000284, -8.156503725454280485 ) ) ;
#54493=CARTESIAN_POINT ( 'NONE',  ( 6.760013919724077169, -79.37708333333333144, -8.796335266379971429 ) ) ;
#54500=ORIENTED_EDGE ( 'NONE', *, *, #53159, .T. ) ;
#54502=CARTESIAN_POINT ( 'NONE',  ( -11.17232872905999841, -77.66848448279598927, 1.511624848520999764 ) ) ;
#54508=CARTESIAN_POINT ( 'NONE',  ( -7.233356275331999541, -78.96555212030999371, 6.024097567370000128 ) ) ;
#54521=EDGE_CURVE ( 'NONE', #4702, #26583, #27460, .T. ) ;
#54535=DIRECTION ( 'NONE',  ( 1.000000000000000000, 0.000000000000000000, 0.000000000000000000 ) ) ;
#54541=CARTESIAN_POINT ( 'NONE',  ( 7.984248283110355615, -78.80795658438964324, -4.671396296726914699 ) ) ;
#54547=EDGE_CURVE ( 'NONE', #36325, #40498, #1397, .T. ) ;
#54553=CARTESIAN_POINT ( 'NONE',  ( 9.489577027016325772, -79.99999999999998579, 0.7465672904055182801 ) ) ;
#54579=CARTESIAN_POINT ( 'NONE',  ( 7.811513588403999897, -79.07336703774899433, 6.067673790570999870 ) ) ;
#54596=CARTESIAN_POINT ( 'NONE',  ( 3.269429986698999979, -79.85814584891350876, 9.203886808668999109 ) ) ;
#54607=CARTESIAN_POINT ( 'NONE',  ( 8.240801834864576847, -79.88798849990462259, 4.200746768372105144 ) ) ;
#54621=CARTESIAN_POINT ( 'NONE',  ( 6.722579162784999340, -79.88047948297999312, 8.904972230874999894 ) ) ;
#54634=CARTESIAN_POINT ( 'NONE',  ( 8.381176496771999496, -77.99792830956099010, 4.744374615790000860 ) ) ;
#54641=CARTESIAN_POINT ( 'NONE',  ( -10.79326785783000098, -79.50498010343598310, -1.992331681952000055 ) ) ;
#54642=DIRECTION ( 'NONE',  ( 1.000000000000000000, 0.000000000000000000, 0.000000000000000000 ) ) ;
#54658=CARTESIAN_POINT ( 'NONE',  ( 5.330257171412455364, -78.28474862486109487, 9.594590749055214474 ) ) ;
#54664=FACE_OUTER_BOUND ( 'NONE', #18841, .T. ) ;
#54676=CARTESIAN_POINT ( 'NONE',  ( -0.01106553558703762298, -77.47524953867433339, 9.249901033550106177 ) ) ;
#54677=CARTESIAN_POINT ( 'NONE',  ( 10.71768947918000059, -78.10758077290198287, -1.656903943290000125 ) ) ;
#54685=CARTESIAN_POINT ( 'NONE',  ( -10.75843888410000027, -79.44371210375499004, -1.985902594052000092 ) ) ;
#54697=CARTESIAN_POINT ( 'NONE',  ( -3.790141024232000166, -77.67121002409098196, -8.616613344227999960 ) ) ;
#54706=CARTESIAN_POINT ( 'NONE',  ( -7.604423127187000198, -79.74545664141298573, 7.914351627518998455 ) ) ;
#54709=DIRECTION ( 'NONE',  ( 0.000000000000000000, 1.000000000000000000, 1.125025998287000022E-13 ) ) ;
#54734=EDGE_LOOP ( 'NONE', ( #25187, #4009, #42392, #24087 ) ) ;
#54737=DIRECTION ( 'NONE',  ( 0.000000000000000000, -1.000000000000000000, 0.000000000000000000 ) ) ;
#54740=CARTESIAN_POINT ( 'NONE',  ( 2.424019779656216400, -78.24625956200173960, -8.927873433679032189 ) ) ;
#54750=CARTESIAN_POINT ( 'NONE',  ( -4.814859605045999302, -78.62586029149998978, 8.425427962446999430 ) ) ;
#54770=CARTESIAN_POINT ( 'NONE',  ( 6.848120951879766771, -77.19999999999998863, -8.441927890790847044 ) ) ;
#54772=CARTESIAN_POINT ( 'NONE',  ( 5.539808784079907511, -78.36666666666667425, -9.611650271896827746 ) ) ;
#54776=CARTESIAN_POINT ( 'NONE',  ( 6.165970644978999715, -79.14971247365699014, 7.554510225358000319 ) ) ;
#54779=LINE ( 'NONE', #14322, #28218 ) ;
#54783=CARTESIAN_POINT ( 'NONE',  ( 10.91664470761000061, -77.98939760156699208, -0.5030651442900000436 ) ) ;
#54787=CARTESIAN_POINT ( 'NONE',  ( 8.191903123214999027, -78.31180405034399428, 4.637231687908999866 ) ) ;
#54792=EDGE_CURVE ( 'NONE', #1603, #39698, #4836, .T. ) ;
#54796=AXIS2_PLACEMENT_3D ( 'NONE', #2241, #6652, #33507 ) ;
#54802=DIRECTION ( 'NONE',  ( 3.675130213670998824E-09, -0.9999999999999997780, -2.168720875627999536E-08 ) ) ;
#54806=EDGE_LOOP ( 'NONE', ( #41954, #22627, #38546, #15230 ) ) ;
#54816=CARTESIAN_POINT ( 'NONE',  ( 2.867595730404614240, -77.99877691775095911, -9.270961250973028811 ) ) ;
#54820=DIRECTION ( 'NONE',  ( -0.7071067811865474617, 0.7071067811865474617, 6.547106584528433984E-10 ) ) ;
#54824=CARTESIAN_POINT ( 'NONE',  ( 5.208840937792781567, -78.77265696413414275, -7.682242898499267447 ) ) ;
#54829=CARTESIAN_POINT ( 'NONE',  ( -8.735356708122031577, -80.15212943903959797, -6.698788252584580327 ) ) ;
#54836=CARTESIAN_POINT ( 'NONE',  ( 6.108123033638238830, -80.00000000000000000, 7.128822434192190194 ) ) ;
#54842=CARTESIAN_POINT ( 'NONE',  ( 3.102135221549690236, -77.30237053728062335, 10.38336816366492243 ) ) ;
#54847=ORIENTED_EDGE ( 'NONE', *, *, #40495, .T. ) ;
#54856=CARTESIAN_POINT ( 'NONE',  ( -4.721094452241000106, -79.18541001252299338, 8.691768742354998523 ) ) ;
#54868=CARTESIAN_POINT ( 'NONE',  ( 8.064399500920000463, -77.80418109758298328, 7.789238951990999915 ) ) ;
#54874=CARTESIAN_POINT ( 'NONE',  ( -5.809791519574999619, -79.25584552244097836, 7.851562197947999699 ) ) ;
#54901=EDGE_CURVE ( 'NONE', #37657, #40036, #49356, .T. ) ;
#54911=CARTESIAN_POINT ( 'NONE',  ( 1.251117773441000169, -77.57157087262599759, 9.549236319306000809 ) ) ;
#54918=CARTESIAN_POINT ( 'NONE',  ( 8.082760247877876836, -77.89183626726020293, 4.658660117716662441 ) ) ;
#54927=AXIS2_PLACEMENT_3D ( 'NONE', #29221, #30079, #33938 ) ;
#54928=CARTESIAN_POINT ( 'NONE',  ( -9.249803168447471080, -77.49364314078148652, 0.7265176776316289997 ) ) ;
#54940=CARTESIAN_POINT ( 'NONE',  ( -3.548359637466153238, -79.54890456983206093, -10.38638352587388169 ) ) ;
#54943=VERTEX_POINT ( 'NONE', #43771 ) ;
#54956=CARTESIAN_POINT ( 'NONE',  ( 10.44963345251333919, -78.02857427158255632, -2.857245842109498835 ) ) ;
#54960=CARTESIAN_POINT ( 'NONE',  ( 9.246497739354760270, -77.35225292060245295, 0.2614339155388125113 ) ) ;
#54961=CARTESIAN_POINT ( 'NONE',  ( -7.062685404271999978, -77.80008692246998692, 8.485436034813998774 ) ) ;
#54963=CARTESIAN_POINT ( 'NONE',  ( 9.703485699160999900, -77.64139207422398670, 0.1143444355825999903 ) ) ;
#54969=CARTESIAN_POINT ( 'NONE',  ( -1.293339008660999934, -78.54475676510898552, -10.86347506762000137 ) ) ;
#54977=PLANE ( 'NONE',  #20072 ) ;
#54985=CARTESIAN_POINT ( 'NONE',  ( 5.254748191175000471, -78.75131553099198811, -7.810174947890000219 ) ) ;
#54988=CARTESIAN_POINT ( 'NONE',  ( 0.000000000000000000, -74.64999999999999147, 0.000000000000000000 ) ) ;
#54994=CARTESIAN_POINT ( 'NONE',  ( 3.915498778898000687, -79.15551720042698491, 10.25343288338999947 ) ) ;
#55006=CARTESIAN_POINT ( 'NONE',  ( 10.83613785003000096, -78.40712618243998122, -3.083350589994000135 ) ) ;
#55023=VERTEX_POINT ( 'NONE', #48487 ) ;
#55032=CARTESIAN_POINT ( 'NONE',  ( 2.003558085140010547, -78.24252397767638456, -9.030659044987556783 ) ) ;
#55036=CARTESIAN_POINT ( 'NONE',  ( -9.164162942852110305, -77.58929706276954619, 1.258628486501499610 ) ) ;
#55040=CARTESIAN_POINT ( 'NONE',  ( -7.456816947376000648, -78.71458704629999659, 6.210200510404999541 ) ) ;
#55054=VECTOR ( 'NONE', #12777, 1000.000000000000000 ) ;
#55057=CARTESIAN_POINT ( 'NONE',  ( 9.345049821197974893, -79.99999999999998579, -1.982164977907467041 ) ) ;
#55071=CARTESIAN_POINT ( 'NONE',  ( 5.571808657063000325, -77.07548692427589287, 9.401125172057000157 ) ) ;
#55072=AXIS2_PLACEMENT_3D ( 'NONE', #11990, #34399, #34104 ) ;
#55076=CARTESIAN_POINT ( 'NONE',  ( 9.227078657215999513, -78.25495639208598675, -1.863387764540999969 ) ) ;
#55091=ORIENTED_EDGE ( 'NONE', *, *, #13017, .F. ) ;
#55096=VERTEX_POINT ( 'NONE', #19224 ) ;
#55104=CARTESIAN_POINT ( 'NONE',  ( -6.766501570400897059, -77.91350543036399756, -6.956168793800119765 ) ) ;
#55112=CARTESIAN_POINT ( 'NONE',  ( 7.284053360365863483, -78.79718121070038706, -5.701434584557759422 ) ) ;
#55116=CARTESIAN_POINT ( 'NONE',  ( -10.06640125953788889, -80.13353945426578662, -4.440637828395845865 ) ) ;
#55117=EDGE_CURVE ( 'NONE', #54943, #31523, #16127, .T. ) ;
#55124=CARTESIAN_POINT ( 'NONE',  ( 4.262694164919158091, -79.99999999999998579, 8.335102471465946294 ) ) ;
#55133=CARTESIAN_POINT ( 'NONE',  ( 0.000000000000000000, -78.69999999999998863, 0.000000000000000000 ) ) ;
#55134=CARTESIAN_POINT ( 'NONE',  ( -9.091539081997000338, -78.80267817997544455, 6.148815634104000338 ) ) ;
#55139=CARTESIAN_POINT ( 'NONE',  ( 8.331241633165971550, -78.31425648247298454, -4.019023800633488186 ) ) ;
#55142=CARTESIAN_POINT ( 'NONE',  ( 9.249483092228999226, -78.85084128437098627, 0.09778817195952001218 ) ) ;
#55143=CARTESIAN_POINT ( 'NONE',  ( -7.735308924444000311, -77.38115727064098337, -5.918161214274000770 ) ) ;
#55148=DIRECTION ( 'NONE',  ( 0.000000000000000000, -1.000000000000000000, 0.000000000000000000 ) ) ;
#55155=CARTESIAN_POINT ( 'NONE',  ( -1.104817622806009147, -77.61549472473473088, -9.262197383512390303 ) ) ;
#55160=CARTESIAN_POINT ( 'NONE',  ( 7.925900958036001143, -77.18054105027188427, -7.930104832517999469 ) ) ;
#55169=CARTESIAN_POINT ( 'NONE',  ( -9.387315177295000979, -79.86818363849698699, 2.697965643110000311 ) ) ;
#55181=CARTESIAN_POINT ( 'NONE',  ( 8.281063756823000332, -76.97785287111209129, -4.978728297554999571 ) ) ;
#55204=CARTESIAN_POINT ( 'NONE',  ( -0.1527179957142000277, -78.08319979694698532, 9.629635879864999026 ) ) ;
#55212=CARTESIAN_POINT ( 'NONE',  ( 9.304500756975000897, -79.19596420577599361, -5.821536072646999571 ) ) ;
#55214=CARTESIAN_POINT ( 'NONE',  ( 7.000000000000000000, -80.99999999999998579, 0.000000000000000000 ) ) ;
#55220=CARTESIAN_POINT ( 'NONE',  ( 0.000000000000000000, -81.99999999999998579, 0.000000000000000000 ) ) ;
#55231=CARTESIAN_POINT ( 'NONE',  ( -4.277805800101380562, -79.04324219184334765, -10.10782847103924631 ) ) ;
#55235=EDGE_CURVE ( 'NONE', #57298, #52316, #36638, .T. ) ;
#55242=AXIS2_PLACEMENT_3D ( 'NONE', #1274, #18395, #13657 ) ;
#55252=CARTESIAN_POINT ( 'NONE',  ( 8.234955035280039581, -77.38774562065144380, 4.212665045149399212 ) ) ;
#55260=CARTESIAN_POINT ( 'NONE',  ( -0.5177219211888000050, -79.05041914309698825, -10.92793577709999830 ) ) ;
#55280=ORIENTED_EDGE ( 'NONE', *, *, #38805, .F. ) ;
#55283=APPLICATION_CONTEXT ( 'automotive_design' ) ;
#55285=CARTESIAN_POINT ( 'NONE',  ( 4.038786804788999873, -79.46453309808698862, -10.20549938643999965 ) ) ;
#55297=CARTESIAN_POINT ( 'NONE',  ( 8.538884422081000736, -77.98574086744999079, 7.349585687664999867 ) ) ;
#55303=LINE ( 'NONE', #14849, #43126 ) ;
#55307=ORIENTED_EDGE ( 'NONE', *, *, #18223, .F. ) ;
#55310=CARTESIAN_POINT ( 'NONE',  ( 2.799999998984000094, -78.69999999898398357, -6.819611318389000073E-10 ) ) ;
#55315=EDGE_CURVE ( 'NONE', #37657, #49174, #48144, .T. ) ;
#55323=CARTESIAN_POINT ( 'NONE',  ( 3.667343776274157197, -78.25747830790810156, -8.492070081455974417 ) ) ;
#55327=CARTESIAN_POINT ( 'NONE',  ( -9.249917423436453845, -77.59781344625758948, 0.2701611356223029836 ) ) ;
#55329=CARTESIAN_POINT ( 'NONE',  ( 10.36935812844000004, -78.17876026662598576, -2.835297515976000327 ) ) ;
#55332=CARTESIAN_POINT ( 'NONE',  ( 9.367484565636001292, -78.99882533758999159, -2.533990228858999938 ) ) ;
#55354=VERTEX_POINT ( 'NONE', #41950 ) ;
#55356=CARTESIAN_POINT ( 'NONE',  ( -6.267465111053000193, -78.04198670514499270, 9.561428071649999083 ) ) ;
#55358=B_SPLINE_CURVE_WITH_KNOTS ( 'NONE', 3,
 ( #52863, #49230, #36521, #22658, #45105, #26772, #44802, #8782, #4354, #40667, #32083, #49829, #39277, #9377, #13785, #258, #14086, #36229, #552, #57287 ),
 .UNSPECIFIED., .F., .F.,
 ( 4, 2, 2, 2, 2, 2, 2, 2, 2, 4 ),
 ( 0.000000000000000000, 0.06250000000000004163, 0.1250000000000000833, 0.2500000000000001110, 0.3750000000000001665, 0.5000000000000002220, 0.6250000000000002220, 0.7500000000000001110, 0.8750000000000001110, 1.000000000000000000 ),
 .UNSPECIFIED. ) ;
#55364=CARTESIAN_POINT ( 'NONE',  ( -9.409947959002000317, -77.72560390012598930, -6.209574706611999950 ) ) ;
#55367=CARTESIAN_POINT ( 'NONE',  ( -4.799999999999999822, -74.99999999999998579, 0.000000000000000000 ) ) ;
#55368=CARTESIAN_POINT ( 'NONE',  ( 4.061470846528000500, -78.68131382901999871, -8.492093326754000415 ) ) ;
#55373=PLANE ( 'NONE',  #15137 ) ;
#55390=ORIENTED_EDGE ( 'NONE', *, *, #27165, .F. ) ;
#55395=CARTESIAN_POINT ( 'NONE',  ( -7.707293733352901022, -77.40187650604293879, -5.896727239374860652 ) ) ;
#55397=DIRECTION ( 'NONE',  ( -1.000000000000000000, 0.000000000000000000, 0.000000000000000000 ) ) ;
#55400=CARTESIAN_POINT ( 'NONE',  ( 7.405962610586998451, -77.44409050277675988, -6.270759699041999369 ) ) ;
#55402=CARTESIAN_POINT ( 'NONE',  ( 8.624362245272223504, -79.63790916909928796, 4.474991579895456262 ) ) ;
#55407=CARTESIAN_POINT ( 'NONE',  ( -7.804500157903205171, -78.64526517801122907, -4.965041426151914905 ) ) ;
#55410=CARTESIAN_POINT ( 'NONE',  ( -3.399186938124999724, -80.19999999999998863, -10.46162167925000119 ) ) ;
#55419=ADVANCED_FACE ( 'NONE', ( #6216 ), #19811, .T. ) ;
#55430=CARTESIAN_POINT ( 'NONE',  ( 0.000000000000000000, -74.64999999999999147, 0.000000000000000000 ) ) ;
#55432=CARTESIAN_POINT ( 'NONE',  ( -6.405050160242000246, -78.77458582564257483, 8.912875463421000788 ) ) ;
#55439=CARTESIAN_POINT ( 'NONE',  ( 8.998106893723814892, -78.33155866549604696, -2.144391086070803532 ) ) ;
#55443=CARTESIAN_POINT ( 'NONE',  ( 5.376158796547000129, -79.06519127177598705, -7.990628517496999983 ) ) ;
#55453=CARTESIAN_POINT ( 'NONE',  ( -4.123528034279000387, -80.08323015146697799, 10.79195219444999942 ) ) ;
#55454=ORIENTED_EDGE ( 'NONE', *, *, #21481, .T. ) ;
#55456=CARTESIAN_POINT ( 'NONE',  ( 5.324680568677000458, -77.65744226292098062, -9.866841419866000606 ) ) ;
#55459=ORIENTED_EDGE ( 'NONE', *, *, #21089, .T. ) ;
#55460=DIRECTION ( 'NONE',  ( 0.7071067811865470176, -0.7071067811865470176, 3.680441446989245012E-08 ) ) ;
#55463=CARTESIAN_POINT ( 'NONE',  ( -4.465297566879000257, -79.80323832198099865, 8.686876450551999085 ) ) ;
#55493=CARTESIAN_POINT ( 'NONE',  ( -3.605088315526999487, -77.23446514106798588, 9.013044129564001139 ) ) ;
#55498=CARTESIAN_POINT ( 'NONE',  ( 3.223804565277000211, -78.05477596781798866, 9.075257246486000184 ) ) ;
#55502=CARTESIAN_POINT ( 'NONE',  ( -6.364729966985085419, -77.77625342220865434, -9.067865724216227719 ) ) ;
#55510=CARTESIAN_POINT ( 'NONE',  ( -8.058638732054999920, -78.54984005612499232, -7.451332657186999775 ) ) ;
#55511=CARTESIAN_POINT ( 'NONE',  ( -10.50034262194430568, -80.07607525657526537, 3.277372812034037075 ) ) ;
#55512=CARTESIAN_POINT ( 'NONE',  ( -9.084942557926000362, -79.55399766404198658, 2.975715551223999888 ) ) ;
#55514=CARTESIAN_POINT ( 'NONE',  ( -1.199999995295999877, -81.00000000470399186, 6.999999972240000368 ) ) ;
#55527=CARTESIAN_POINT ( 'NONE',  ( -10.65690479855507000, -78.93087277451306250, 2.626442266231765021 ) ) ;
#55529=ORIENTED_EDGE ( 'NONE', *, *, #33603, .F. ) ;
#55544=CARTESIAN_POINT ( 'NONE',  ( 7.483246165179296305, -77.40010939284451297, 5.437107557591821738 ) ) ;
#55547=CARTESIAN_POINT ( 'NONE',  ( -7.707166124622999881, -77.44242527032199064, -5.896629607976000109 ) ) ;
#55552=CARTESIAN_POINT ( 'NONE',  ( 7.840491480036000382, -78.80527898622098348, 7.784894796889999746 ) ) ;
#55554=DIRECTION ( 'NONE',  ( 0.000000000000000000, 0.7071067811866525998, -0.7071067811864425456 ) ) ;
#55560=CARTESIAN_POINT ( 'NONE',  ( -10.84960119849321281, -77.20000000000000284, 1.688458811413132699 ) ) ;
#55564=MANIFOLD_SOLID_BREP ( 'Stock-MAS-694-1', #31467 ) ;
#55569=CARTESIAN_POINT ( 'NONE',  ( 7.429344776774999382, -78.38180575231598368, 5.780660057059999524 ) ) ;
#55581=CARTESIAN_POINT ( 'NONE',  ( -8.631379868284000167, -78.31686478745199054, 6.779623747090999686 ) ) ;
#55604=PRESENTATION_STYLE_ASSIGNMENT (( #37586 ) ) ;
#55607=VERTEX_POINT ( 'NONE', #173 ) ;
#55608=ORIENTED_EDGE ( 'NONE', *, *, #19106, .F. ) ;
#55610=EDGE_LOOP ( 'NONE', ( #44824, #28176, #58325, #33964, #58027 ) ) ;
#55614=CARTESIAN_POINT ( 'NONE',  ( -8.744140569414998510, -80.29580545329308450, 7.086030162020000134 ) ) ;
#55617=CARTESIAN_POINT ( 'NONE',  ( 5.882476073987271015, -78.27997737893470287, -7.138446288670057704 ) ) ;
#55621=CARTESIAN_POINT ( 'NONE',  ( -9.175128499341100863, -77.59002790297775221, 1.175099295633919017 ) ) ;
#55625=CARTESIAN_POINT ( 'NONE',  ( 9.045658679128999680, -79.04619838613798777, 3.115350657311999782 ) ) ;
#55626=DIRECTION ( 'NONE',  ( 1.000000000000000000, 0.000000000000000000, 0.000000000000000000 ) ) ;
#55628=CARTESIAN_POINT ( 'NONE',  ( -8.254612054926999676, -79.75421655541097721, 6.886499823760000361 ) ) ;
#55633=DIRECTION ( 'NONE',  ( -1.000000000000000000, 0.000000000000000000, 0.000000000000000000 ) ) ;
#55643=CARTESIAN_POINT ( 'NONE',  ( 9.499999794217913518, -79.99999999999998579, -1.003825360198642880 ) ) ;
#55647=CARTESIAN_POINT ( 'NONE',  ( 8.796335266379992746, -78.39791666666666003, -6.760013919724047859 ) ) ;
#55650=CARTESIAN_POINT ( 'NONE',  ( -6.184040273379711294, -77.17951720182109909, -6.972051400811474231 ) ) ;
#55652=CARTESIAN_POINT ( 'NONE',  ( 9.457014981167999323, -79.13566112575199440, -0.8878631254947999540 ) ) ;
#55654=LINE ( 'NONE', #20795, #42199 ) ;
#55658=CARTESIAN_POINT ( 'NONE',  ( 3.913900004701999613, -77.58956168025198963, 10.45689208369000056 ) ) ;
#55659=CIRCLE ( 'NONE', #45258, 1.000000000000000000 ) ;
#55671=CARTESIAN_POINT ( 'NONE',  ( 0.000000000000000000, -81.99999999999998579, -4.299999999999968736 ) ) ;
#55680=EDGE_CURVE ( 'NONE', #43667, #54465, #40575, .T. ) ;
#55700=B_SPLINE_CURVE_WITH_KNOTS ( 'NONE', 3,
 ( #12241, #47702, #52404, #11958, #57681, #47989, #7525, #25522, #51833, #11388, #47413, #6943, #43539, #21098, #57111, #30232, #45294, #22840 ),
 .UNSPECIFIED., .F., .F.,
 ( 4, 2, 2, 2, 2, 2, 2, 2, 4 ),
 ( 0.000000000000000000, 0.1250000000000000000, 0.2500000000000000000, 0.3750000000000000000, 0.5000000000000000000, 0.6250000000000000000, 0.7500000000000000000, 0.8750000000000000000, 1.000000000000000000 ),
 .UNSPECIFIED. ) ;
#55703=CARTESIAN_POINT ( 'NONE',  ( -7.868794148055054727, -78.64422463589345114, -4.862493407595640527 ) ) ;
#55710=CARTESIAN_POINT ( 'NONE',  ( -7.774388101806787077, -80.16288445207561608, -7.781834858813881262 ) ) ;
#55718=CARTESIAN_POINT ( 'NONE',  ( 5.674932013357969041, -79.99999999999998579, 7.468275051675760778 ) ) ;
#55726=EDGE_CURVE ( 'NONE', #15959, #6548, #2635, .T. ) ;
#55729=CARTESIAN_POINT ( 'NONE',  ( 1.674065321307220300, -77.58787199535142065, -10.64115275760022605 ) ) ;
#55731=CARTESIAN_POINT ( 'NONE',  ( -9.505686244346000180, -79.30834055796346149, 5.486888517706000279 ) ) ;
#55733=EDGE_LOOP ( 'NONE', ( #55459, #41191, #21979, #32137 ) ) ;
#55737=DIRECTION ( 'NONE',  ( -1.000000000000000000, 0.000000000000000000, 0.000000000000000000 ) ) ;
#55740=CARTESIAN_POINT ( 'NONE',  ( -5.370832524224000259, -77.75066704931698780, 8.124890996387998499 ) ) ;
#55751=CARTESIAN_POINT ( 'NONE',  ( 11.01715842067999951, -78.56297001833898719, 0.8367281403419999375 ) ) ;
#55752=CARTESIAN_POINT ( 'NONE',  ( 4.714910253073366420, -77.66722752291366305, -8.048511890795102985 ) ) ;
#55757=CARTESIAN_POINT ( 'NONE',  ( 10.79265454957999992, -77.83137212970099483, 3.422111395643999909 ) ) ;
#55760=ORIENTED_EDGE ( 'NONE', *, *, #31865, .F. ) ;
#55762=EDGE_CURVE ( 'NONE', #46115, #1066, #33008, .T. ) ;
#55764=CARTESIAN_POINT ( 'NONE',  ( -7.545891804452000251, -79.83571098023898571, 6.201630566990999682 ) ) ;
#55768=EDGE_LOOP ( 'NONE', ( #52348, #38747, #5503, #21172 ) ) ;
#55771=CIRCLE ( 'NONE', #45407, 4.299999999999999822 ) ;
#55792=CARTESIAN_POINT ( 'NONE',  ( -2.858782626228999924, -76.99373160055630194, -9.043346509775000541 ) ) ;
#55806=CARTESIAN_POINT ( 'NONE',  ( -6.920341278396000106, -79.56116481210098357, -8.518972542050999408 ) ) ;
#55808=CARTESIAN_POINT ( 'NONE',  ( -0.2701109549781999797, -78.95643513191498641, 9.556054066276999492 ) ) ;
#55824=DIRECTION ( 'NONE',  ( -1.000000000000000000, 0.000000000000000000, 0.000000000000000000 ) ) ;
#55825=CARTESIAN_POINT ( 'NONE',  ( -10.81666588859962275, -79.43653515250106523, 1.862137996412334795 ) ) ;
#55844=CARTESIAN_POINT ( 'NONE',  ( 7.475510798934743129, -77.40022076363275971, 5.447743833593036378 ) ) ;
#55845=CARTESIAN_POINT ( 'NONE',  ( 9.507661145905998978, -77.69802481315399234, -5.611464101879999333 ) ) ;
#55852=CARTESIAN_POINT ( 'NONE',  ( -10.72788417900999924, -78.97383311221699387, 2.643935454766999982 ) ) ;
#55857=ORIENTED_EDGE ( 'NONE', *, *, #26817, .F. ) ;
#55859=CARTESIAN_POINT ( 'NONE',  ( -10.80118587004463393, -77.19999999999998863, 1.952987246723529413 ) ) ;
#55869=CARTESIAN_POINT ( 'NONE',  ( -8.985695946343000173, -78.61622446787298202, 3.150816496261000133 ) ) ;
#55880=CARTESIAN_POINT ( 'NONE',  ( 10.71556987377000070, -79.57690251541698956, 2.374990294079000197 ) ) ;
#55890=CARTESIAN_POINT ( 'NONE',  ( -5.907589619820999616, -78.09811028477999173, 9.593191298321000815 ) ) ;
#55900=EDGE_CURVE ( 'NONE', #11974, #26900, #39936, .T. ) ;
#55915=AXIS2_PLACEMENT_3D ( 'NONE', #32981, #36261, #19430 ) ;
#55917=CARTESIAN_POINT ( 'NONE',  ( 5.414928535605519677, -78.27494612867262447, -7.499721313425219194 ) ) ;
#55918=CARTESIAN_POINT ( 'NONE',  ( -2.460623815919318336, -79.39618386848788134, 8.998003677019603685 ) ) ;
#55925=CARTESIAN_POINT ( 'NONE',  ( 9.259046916275000427, -78.54404407152598822, 2.905298533503999803 ) ) ;
#55932=DIRECTION ( 'NONE',  ( 0.000000000000000000, -1.000000000000000000, 0.000000000000000000 ) ) ;
#55941=CARTESIAN_POINT ( 'NONE',  ( 8.724294832244513742, -79.99999999999995737, -3.890814657221138173 ) ) ;
#55944=VERTEX_POINT ( 'NONE', #49235 ) ;
#55949=CARTESIAN_POINT ( 'NONE',  ( -8.641832836834998588, -79.85648669611498462, 4.277501108045999700 ) ) ;
#55956=CARTESIAN_POINT ( 'NONE',  ( 4.360500596435000098, -77.21275830873099721, 9.871531364361999294 ) ) ;
#55967=ORIENTED_EDGE ( 'NONE', *, *, #46836, .F. ) ;
#55973=EDGE_CURVE ( 'NONE', #4702, #27444, #12628, .T. ) ;
#55993=FACE_OUTER_BOUND ( 'NONE', #51267, .T. ) ;
#55994=CARTESIAN_POINT ( 'NONE',  ( 9.512131559252001267, -77.98414325622765375, -1.920953556448999899 ) ) ;
#55997=CARTESIAN_POINT ( 'NONE',  ( -2.879226727952121312, -78.59583333333331723, 10.71369944335146052 ) ) ;
#55999=CARTESIAN_POINT ( 'NONE',  ( -8.158649804916262127, -78.63917908708265259, -4.359350819807166211 ) ) ;
#56002=CARTESIAN_POINT ( 'NONE',  ( -9.038121182379606822, -80.14837150988061865, -6.270795222358383825 ) ) ;
#56018=CARTESIAN_POINT ( 'NONE',  ( 9.943037443271171227, -78.16907139213840594, -4.146583387419329192 ) ) ;
#56020=CARTESIAN_POINT ( 'NONE',  ( -10.79326785783000098, -79.36452526662860407, -1.992331681952000055 ) ) ;
#56022=ORIENTED_EDGE ( 'NONE', *, *, #11328, .F. ) ;
#56026=CARTESIAN_POINT ( 'NONE',  ( 9.114089478082622264, -78.33640746566551627, -1.588185711488315111 ) ) ;
#56030=CARTESIAN_POINT ( 'NONE',  ( 8.977320902561999105, -79.16941197858199075, 3.091814932086999868 ) ) ;
#56033=CIRCLE ( 'NONE', #435, 4.299999999999999822 ) ;
#56040=CARTESIAN_POINT ( 'NONE',  ( -4.306297750730000651, -78.90007827033099375, -10.17515077672999979 ) ) ;
#56041=CARTESIAN_POINT ( 'NONE',  ( 1.300393966725080341, -77.63618784400628670, -9.236768800945032609 ) ) ;
#56042=CARTESIAN_POINT ( 'NONE',  ( -0.9999999970599000587, -81.20000000293998710, 6.999999982650000341 ) ) ;
#56044=ADVANCED_FACE ( 'NONE', ( #22060 ), #20765, .F. ) ;
#56046=CARTESIAN_POINT ( 'NONE',  ( 10.95487136366999970, -78.29604510612898594, -1.495655693045000012 ) ) ;
#56053=CARTESIAN_POINT ( 'NONE',  ( -9.687172913667000174, -80.14036198365600683, -1.248753675804000096 ) ) ;
#56057=EDGE_CURVE ( 'NONE', #53060, #29148, #55659, .T. ) ;
#56070=CARTESIAN_POINT ( 'NONE',  ( -9.611650271896833075, -79.64166666666665151, -5.539808784079895077 ) ) ;
#56082=CARTESIAN_POINT ( 'NONE',  ( 2.642581390489999738, -77.18224640713208373, 9.340684087520999768 ) ) ;
#56090=CARTESIAN_POINT ( 'NONE',  ( 9.462239583049713687, -76.98776041667790082, 1.239456478693297559 ) ) ;
#56092=DIRECTION ( 'NONE',  ( 0.000000000000000000, 0.000000000000000000, -1.000000000000000000 ) ) ;
#56100=CARTESIAN_POINT ( 'NONE',  ( -10.97527124375647389, -80.09511974427576320, 0.7348162751891352817 ) ) ;
#56101=CARTESIAN_POINT ( 'NONE',  ( 9.142801562799000692, -79.85277893010599826, 2.792903297447999922 ) ) ;
#56104=ORIENTED_EDGE ( 'NONE', *, *, #52241, .F. ) ;
#56116=CARTESIAN_POINT ( 'NONE',  ( -4.399313083005135461, -79.85792046749108408, 10.05553542149106150 ) ) ;
#56134=CARTESIAN_POINT ( 'NONE',  ( 8.679236020840834342, -77.37813114295693140, 3.200552027347492778 ) ) ;
#56136=CIRCLE ( 'NONE', #47689, 10.69999999999999929 ) ;
#56144=CARTESIAN_POINT ( 'NONE',  ( -7.579884289019999777, -79.86509741874499468, 7.888812675972000754 ) ) ;
#56147=CARTESIAN_POINT ( 'NONE',  ( -9.750000000000000000, -76.19999999999998863, 0.000000000000000000 ) ) ;
#56158=CARTESIAN_POINT ( 'NONE',  ( 6.852546780225999612, -78.33198617658298701, -6.611579150008999761 ) ) ;
#56170=CARTESIAN_POINT ( 'NONE',  ( 8.318585563179999198, -78.23670594145998791, 7.159970128962999780 ) ) ;
#56178=CARTESIAN_POINT ( 'NONE',  ( -7.396918292183171317, -78.05208333333331439, -5.684557159767958723 ) ) ;
#56181=CARTESIAN_POINT ( 'NONE',  ( 9.478197642333000772, -79.47463564708098716, 6.090377947633999867 ) ) ;
#56185=B_SPLINE_CURVE_WITH_KNOTS ( 'NONE', 3,
 ( #21843, #18315, #12979, #7985, #49310, #8860, #36306, #54330, #30409, #53152 ),
 .UNSPECIFIED., .F., .F.,
 ( 4, 2, 2, 2, 4 ),
 ( 0.000000000000000000, 0.2499999999999998890, 0.4999999999999997780, 0.7499999999999998890, 1.000000000000000000 ),
 .UNSPECIFIED. ) ;
#56188=AXIS2_PLACEMENT_3D ( 'NONE', #22814, #54413, #13359 ) ;
#56198=CARTESIAN_POINT ( 'NONE',  ( 5.749221480030474396, -79.92640261716472594, -7.622783030296528040 ) ) ;
#56205=CARTESIAN_POINT ( 'NONE',  ( 0.2313529605545296963, -78.22705442624081229, -9.247502900338933074 ) ) ;
#56206=CARTESIAN_POINT ( 'NONE',  ( 8.984871306655115575, -79.27160451067341285, 2.508152175999946110 ) ) ;
#56209=CARTESIAN_POINT ( 'NONE',  ( -8.798468283297333770, -77.57506182485165880, 2.854659429539475823 ) ) ;
#56212=CARTESIAN_POINT ( 'NONE',  ( -1.565122400816999937, -78.65773938804198906, 9.577113408380000692 ) ) ;
#56225=B_SPLINE_CURVE_WITH_KNOTS ( 'NONE', 3,
 ( #30988, #21573, #39578, #17143 ),
 .UNSPECIFIED., .F., .F.,
 ( 4, 4 ),
 ( 0.000000000000000000, 1.000000000000000000 ),
 .UNSPECIFIED. ) ;
#56241=CARTESIAN_POINT ( 'NONE',  ( -7.398415933695000390, -79.51124522128699823, -6.012806692959999921 ) ) ;
#56245=CARTESIAN_POINT ( 'NONE',  ( -6.760013919724056741, -77.27291666666666003, -8.796335266379987416 ) ) ;
#56247=CARTESIAN_POINT ( 'NONE',  ( -10.95675378139999978, -77.79623596436198341, 1.482457388852999935 ) ) ;
#56254=CARTESIAN_POINT ( 'NONE',  ( -6.760013919724099374, -77.52708333333332291, 8.796335266379958995 ) ) ;
#56286=CARTESIAN_POINT ( 'NONE',  ( 7.714905556308770507, -79.55033101189913225, -5.543136766205470245 ) ) ;
#56289=CARTESIAN_POINT ( 'NONE',  ( -4.767438741492489029, -78.68199087655180790, -7.927228674465881753 ) ) ;
#56307=CARTESIAN_POINT ( 'NONE',  ( -7.222015211734788664, -77.88356993406765127, 8.081286372382828986 ) ) ;
#56308=CARTESIAN_POINT ( 'NONE',  ( 4.977885330626822480, -78.26203852219340718, -9.897304379485547088 ) ) ;
#56309=CARTESIAN_POINT ( 'NONE',  ( -10.81649518602000093, -79.33643291229606120, 1.862108609190000097 ) ) ;
#56312=AXIS2_PLACEMENT_3D ( 'NONE', #707, #31357, #9536 ) ;
#56320=CARTESIAN_POINT ( 'NONE',  ( -8.711966356949998769, -77.29588578325397918, 3.874524904258000557 ) ) ;
#56335=CARTESIAN_POINT ( 'NONE',  ( -4.735947112136000392, -77.71182432715698951, -10.40542313098000093 ) ) ;
#56339=CARTESIAN_POINT ( 'NONE',  ( 9.523132023602000729, -80.38931903029605053, 1.108936319727999997 ) ) ;
#56352=CARTESIAN_POINT ( 'NONE',  ( -9.554603705186000440, -77.21387085810299311, 0.6301758013986999973 ) ) ;
#56355=CARTESIAN_POINT ( 'NONE',  ( 10.71369944335147473, -79.82916666666666572, -2.879226727952063580 ) ) ;
#56375=CARTESIAN_POINT ( 'NONE',  ( -9.721291027688000241, -77.26593683473198837, 0.5965459135819000114 ) ) ;
#56377=CARTESIAN_POINT ( 'NONE',  ( 7.174506471390958318, -77.88110187774557858, -8.441707957340309321 ) ) ;
#56382=CARTESIAN_POINT ( 'NONE',  ( 9.499178638196321245, -79.00092112126561972, 0.1004274591880019996 ) ) ;
#56386=CARTESIAN_POINT ( 'NONE',  ( -10.95656768982416374, -80.09333027791306847, 0.9740957217062806706 ) ) ;
#56387=CARTESIAN_POINT ( 'NONE',  ( -6.834812918901999268, -79.58052574656798583, 6.841065568902999772 ) ) ;
#56389=CARTESIAN_POINT ( 'NONE',  ( -8.796335266379978535, -78.65208333333333712, -6.760013919724068288 ) ) ;
#56404=CARTESIAN_POINT ( 'NONE',  ( -7.545891804452000251, -79.65480220322699267, 6.201630566990999682 ) ) ;
#56409=ORIENTED_EDGE ( 'NONE', *, *, #22500, .T. ) ;
#56412=CARTESIAN_POINT ( 'NONE',  ( -9.022399766209378669, -78.87991562074994079, -3.573531901437693392 ) ) ;
#56423=CARTESIAN_POINT ( 'NONE',  ( 8.103228132958101071, -77.31002185566839557, -4.473611354302846621 ) ) ;
#56430=CARTESIAN_POINT ( 'NONE',  ( 9.499549289235639904, -79.50042064254546403, 0.05021470316550929319 ) ) ;
#56433=CARTESIAN_POINT ( 'NONE',  ( -9.839875214663999614, -79.89318977307699754, 4.781661263485999847 ) ) ;
#56438=CARTESIAN_POINT ( 'NONE',  ( -8.905521014750718223, -77.20000000000000284, 6.316176128476434393 ) ) ;
#56446=CARTESIAN_POINT ( 'NONE',  ( -9.520207861471000399, -78.64464829700199289, -0.1897854149113999966 ) ) ;
#56458=CARTESIAN_POINT ( 'NONE',  ( -10.96673197750000206, -78.37304949611799998, -0.4413686857046000278 ) ) ;
#56468=CARTESIAN_POINT ( 'NONE',  ( -10.98029981754000062, -79.67128212740999516, 1.094250890400999987 ) ) ;
#56484=EDGE_LOOP ( 'NONE', ( #15606, #47933, #458, #38173, #7244 ) ) ;
#56493=CARTESIAN_POINT ( 'NONE',  ( -9.010884632761600344, -79.47923677369759332, 2.413026703165237041 ) ) ;
#56496=VERTEX_POINT ( 'NONE', #16150 ) ;
#56497=CARTESIAN_POINT ( 'NONE',  ( -5.966983627959768555, -77.53090078892917347, 7.069611082095726751 ) ) ;
#56500=CARTESIAN_POINT ( 'NONE',  ( 9.512131559252001267, -78.06429424374599080, -1.920953556448999899 ) ) ;
#56517=CARTESIAN_POINT ( 'NONE',  ( -8.926170656458999986, -80.10939231032499208, -6.915662452114000658 ) ) ;
#56522=FACE_OUTER_BOUND ( 'NONE', #14417, .T. ) ;
#56525=CARTESIAN_POINT ( 'NONE',  ( -8.708088497213999801, -79.42357724651299122, 3.880669710089999835 ) ) ;
#56533=CARTESIAN_POINT ( 'NONE',  ( -6.437501231206999464, -77.94579083114099660, -8.855128588742999796 ) ) ;
#56563=AXIS2_PLACEMENT_3D ( 'NONE', #23422, #14263, #2171 ) ;
#56571=CARTESIAN_POINT ( 'NONE',  ( -9.351608161489666671, -79.87169043516298927, -2.636777050789346433 ) ) ;
#56575=CARTESIAN_POINT ( 'NONE',  ( -5.134245522647685078, -78.67830135142374104, -7.694191572061213513 ) ) ;
#56577=CARTESIAN_POINT ( 'NONE',  ( -10.40480953490025762, -80.12661506326949734, -3.571040318220447318 ) ) ;
#56594=CARTESIAN_POINT ( 'NONE',  ( -5.104594291233171433, -78.03651714374842641, -9.559420401355287922 ) ) ;
#56604=CARTESIAN_POINT ( 'NONE',  ( -8.705161348369998109, -77.92823810661599282, -4.119875709756000148 ) ) ;
#56608=ORIENTED_EDGE ( 'NONE', *, *, #14950, .F. ) ;
#56613=EDGE_LOOP ( 'NONE', ( #28447, #33357, #52614, #37301 ) ) ;
#56614=CARTESIAN_POINT ( 'NONE',  ( -10.64215094251999894, -79.78966949086598959, 2.340290094375000240 ) ) ;
#56617=ORIENTED_EDGE ( 'NONE', *, *, #27096, .F. ) ;
#56619=CARTESIAN_POINT ( 'NONE',  ( 11.18830539140000013, -77.79468742103497902, -1.736105152156000031 ) ) ;
#56626=CARTESIAN_POINT ( 'NONE',  ( 8.944729675425000082, -79.91305337584603308, 3.923329690209000908 ) ) ;
#56637=CYLINDRICAL_SURFACE ( 'NONE', #19467, 1.000000000000000000 ) ;
#56656=CARTESIAN_POINT ( 'NONE',  ( -8.075449341071999854, -77.47831109735399480, 4.776159278919000606 ) ) ;
#56662=CARTESIAN_POINT ( 'NONE',  ( 9.738918081334000831, -77.52175129689300093, 0.1147619655163999997 ) ) ;
#56663=DIRECTION ( 'NONE',  ( 0.000000000000000000, 1.000000000000000000, 0.000000000000000000 ) ) ;
#56669=CARTESIAN_POINT ( 'NONE',  ( 2.375899324488051523, -79.10491627289971461, 9.218980594236693804 ) ) ;
#56674=CARTESIAN_POINT ( 'NONE',  ( -4.562954320814999853, -78.99378279017300031, 8.400624927051000057 ) ) ;
#56676=CARTESIAN_POINT ( 'NONE',  ( 2.879226727952094222, -78.74583333333333712, -10.71369944335146940 ) ) ;
#56686=AXIS2_PLACEMENT_3D ( 'NONE', #5642, #50829, #18659 ) ;
#56691=ADVANCED_FACE ( 'NONE', ( #28476 ), #44627, .F. ) ;
#56693=EDGE_LOOP ( 'NONE', ( #52130, #54847, #9651, #46251 ) ) ;
#56708=CARTESIAN_POINT ( 'NONE',  ( 3.536272283845561581, -79.94387417217693326, 8.547291296781429182 ) ) ;
#56713=CARTESIAN_POINT ( 'NONE',  ( 7.485102092340309987, -77.30010087969016297, -5.434593418087672489 ) ) ;
#56724=CARTESIAN_POINT ( 'NONE',  ( -7.069392057028999865, -79.42331078153999613, 8.491265488204000178 ) ) ;
#56729=CARTESIAN_POINT ( 'NONE',  ( -2.952210844699811432, -77.20000000000000284, 10.42826508716522227 ) ) ;
#56734=CARTESIAN_POINT ( 'NONE',  ( -9.469606800734000629, -80.05752053325198858, 5.597012331546999953 ) ) ;
#56735=AXIS2_PLACEMENT_3D ( 'NONE', #31167, #18216, #9934 ) ;
#56739=CARTESIAN_POINT ( 'NONE',  ( -6.639445101857000431, -77.70666193574498948, -6.825550891425999467 ) ) ;
#56745=CARTESIAN_POINT ( 'NONE',  ( -9.250000000000007105, -78.98958333333331439, 1.210822168571027868 ) ) ;
#56748=CARTESIAN_POINT ( 'NONE',  ( -9.505686244346000180, -79.32818954342899076, 5.486888517706000279 ) ) ;
#56758=CARTESIAN_POINT ( 'NONE',  ( 0.000000000000000000, -78.49999999999998579, 0.000000000000000000 ) ) ;
#56760=CARTESIAN_POINT ( 'NONE',  ( -1.319038368507000181, -78.35863250589198969, -11.07933831235000177 ) ) ;
#56766=DIRECTION ( 'NONE',  ( -1.000000000000000000, 0.000000000000000000, 0.000000000000000000 ) ) ;
#56778=CARTESIAN_POINT ( 'NONE',  ( 0.000000000000000000, -74.99999999999998579, 0.000000000000000000 ) ) ;
#56784=CARTESIAN_POINT ( 'NONE',  ( -7.230939086545548733, -77.54644391223615685, 5.768963832296065242 ) ) ;
#56788=CARTESIAN_POINT ( 'NONE',  ( 9.690463944985998168, -78.57592316806800170, -0.5153813127049999832 ) ) ;
#56793=CARTESIAN_POINT ( 'NONE',  ( -1.870137171474999915, -80.04186706810699548, -11.09839649295000008 ) ) ;
#56805=CARTESIAN_POINT ( 'NONE',  ( 9.105092338905999227, -80.29234472691199187, 6.490636970390999849 ) ) ;
#56810=ORIENTED_EDGE ( 'NONE', *, *, #11460, .F. ) ;
#56816=CARTESIAN_POINT ( 'NONE',  ( -4.800609161379000511, -79.47659213876198692, -8.362561951962998563 ) ) ;
#56822=CARTESIAN_POINT ( 'NONE',  ( 10.71369944335147828, -77.42916666666667425, -2.879226727952064913 ) ) ;
#56825=CARTESIAN_POINT ( 'NONE',  ( -3.891189893006000045, -77.71055683836598860, 10.34924028849999900 ) ) ;
#56829=CARTESIAN_POINT ( 'NONE',  ( -6.294203684166999935, -77.14093373070529935, 7.343715272572999275 ) ) ;
#56831=CARTESIAN_POINT ( 'NONE',  ( 2.879226727952049814, -77.45416666666666572, 10.71369944335148183 ) ) ;
#56861=CARTESIAN_POINT ( 'NONE',  ( -9.611650271896857944, -78.65833333333331723, 5.539808784079855997 ) ) ;
#56867=CARTESIAN_POINT ( 'NONE',  ( -10.31854526085034252, -80.12852127511105493, -3.810993520750592278 ) ) ;
#56886=CARTESIAN_POINT ( 'NONE',  ( -9.247932426686000795, -77.50168256874098915, -0.1955654147372000162 ) ) ;
#56895=CARTESIAN_POINT ( 'NONE',  ( -7.316919381717999826, -78.90167637952698954, 6.093690752987000359 ) ) ;
#56901=CARTESIAN_POINT ( 'NONE',  ( -5.706217103757095011, -79.02772280010032091, 7.378253461501310007 ) ) ;
#56905=CARTESIAN_POINT ( 'NONE',  ( 3.197825632618000125, -79.65857183731299074, 10.57600109144000022 ) ) ;
#56908=CARTESIAN_POINT ( 'NONE',  ( -8.391469517572000214, -79.68773307352599033, 7.000674649436000152 ) ) ;
#56914=AXIS2_PLACEMENT_3D ( 'NONE', #33723, #15726, #34297 ) ;
#56916=CARTESIAN_POINT ( 'NONE',  ( -0.5483576180056000116, -79.75069008456101471, -9.751923335751000010 ) ) ;
#56939=CARTESIAN_POINT ( 'NONE',  ( -9.146705800622001448, -77.53052983129099118, -1.122373973676000114 ) ) ;
#56944=CARTESIAN_POINT ( 'NONE',  ( -9.662137344075999223, -78.26077085424698510, 1.225886475437000023 ) ) ;
#56949=VERTEX_POINT ( 'NONE', #13228 ) ;
#56950=ADVANCED_FACE ( 'NONE', ( #14116 ), #31418, .F. ) ;
#56953=CARTESIAN_POINT ( 'NONE',  ( 5.720594865934685025, -79.07369316860736319, 7.609982227002291211 ) ) ;
#56954=FACE_OUTER_BOUND ( 'NONE', #34825, .T. ) ;
#56957=CARTESIAN_POINT ( 'NONE',  ( -4.510937018225000372, -79.79379212038298874, -8.678390893359001268 ) ) ;
#56960=ORIENTED_EDGE ( 'NONE', *, *, #55235, .F. ) ;
#56968=VERTEX_POINT ( 'NONE', #28782 ) ;
#56973=CARTESIAN_POINT ( 'NONE',  ( 5.411006671257999834, -79.03782169632599164, 8.131518144102999557 ) ) ;
#56981=CARTESIAN_POINT ( 'NONE',  ( -11.00000000000000000, -77.69999999999998863, 0.000000000000000000 ) ) ;
#56988=CARTESIAN_POINT ( 'NONE',  ( 5.266508667217213890, -79.92729844318292010, 7.604169021590073463 ) ) ;
#56992=CARTESIAN_POINT ( 'NONE',  ( 4.757299607910999484, -78.96112282211998945, 10.21259197296000032 ) ) ;
#56993=CARTESIAN_POINT ( 'NONE',  ( 7.610095849401467660, -77.30199033518762519, -5.258407757687174389 ) ) ;
#56999=CARTESIAN_POINT ( 'NONE',  ( -4.100000000000000533, -75.19999999999998863, 0.000000000000000000 ) ) ;
#57002=CARTESIAN_POINT ( 'NONE',  ( -8.774483958462999666, -78.50395412067899770, 6.892026619272999532 ) ) ;
#57004=FACE_OUTER_BOUND ( 'NONE', #7543, .T. ) ;
#57011=DIRECTION ( 'NONE',  ( -1.000000000000000000, 0.000000000000000000, 0.000000000000000000 ) ) ;
#57015=DIRECTION ( 'NONE',  ( 1.000000000000000000, 0.000000000000000000, 0.000000000000000000 ) ) ;
#57017=CARTESIAN_POINT ( 'NONE',  ( 9.403616370364000332, -77.90562873964798030, 1.497456306884999977 ) ) ;
#57024=B_SPLINE_CURVE_WITH_KNOTS ( 'NONE', 3,
 ( #51095, #10647, #33920, #29773, #34205, #12081, #47549, #12650, #38936, #48113, #11798, #48678, #52524, #52242, #38651, #16802, #30063, #7645, #7074, #11516, #16513, #47829, #43375, #52811, #34495, #25076, #57521, #25645, #15933, #43671, #30643, #43100, #30352, #7360, #20367, #3229, #21218, #17082, #12363, #48395, #25359, #39225, #21510, #8222, #34786, #35063, #20934, #2933, #2657, #42806, #56669, #39516, #57238, #56953, #7932, #25933, #43959, #16225, #3508, #53100, #2369, #20651, #38360, #56382 ),
 .UNSPECIFIED., .F., .F.,
 ( 4, 2, 2, 2, 2, 2, 2, 2, 2, 2, 2, 2, 2, 2, 1, 1, 1, 1, 1, 2, 2, 2, 2, 2, 2, 2, 2, 2, 1, 2, 2, 2, 2, 2, 4 ),
 ( 0.5000000000000000000, 0.5312499999999996669, 0.5624999999999993339, 0.5937499999999990008, 0.6249999999999986677, 0.6406249999999985567, 0.6562499999999983347, 0.6718749999999982236, 0.6874999999999980016, 0.7031249999999977796, 0.7187499999999976685, 0.7343749999999975575, 0.7421874999999974465, 0.7460937499999973355, 0.7480468749999973355, 0.7490234374999973355, 0.7495117187499973355, 0.7497558593749973355, 0.7498779296874973355, 0.7499389648437473355, 0.7499999999999973355, 0.7812499999999976685, 0.8124999999999980016, 0.8281249999999982236, 0.8437499999999983347, 0.8593749999999984457, 0.8749999999999986677, 0.8906249999999987788, 0.9062499999999988898, 0.9218749999999991118, 0.9374999999999993339, 0.9531249999999994449, 0.9687499999999995559, 0.9843749999999997780, 1.000000000000000000 ),
 .UNSPECIFIED. ) ;
#57032=CARTESIAN_POINT ( 'NONE',  ( 0.2613587267741000475, -79.49674366942500114, -10.97249781033000104 ) ) ;
#57038=ORIENTED_EDGE ( 'NONE', *, *, #34529, .F. ) ;
#57043=CARTESIAN_POINT ( 'NONE',  ( 0.1325202778310999863, -79.05325033209098251, 11.26549478459000042 ) ) ;
#57053=ORIENTED_EDGE ( 'NONE', *, *, #47840, .T. ) ;
#57068=CARTESIAN_POINT ( 'NONE',  ( -2.588076551402957115, -77.49760603155162642, 8.885074677331601833 ) ) ;
#57069=CARTESIAN_POINT ( 'NONE',  ( -1.776188306762000124, -77.42168691014599347, -10.89629776253999971 ) ) ;
#57072=CARTESIAN_POINT ( 'NONE',  ( -8.771427373352999268, -77.86532743984299998, -4.151237309591000013 ) ) ;
#57075=CARTESIAN_POINT ( 'NONE',  ( 1.791008777272000030, -80.23213113446799127, 11.11143388882000060 ) ) ;
#57080=LINE ( 'NONE', #16067, #55054 ) ;
#57084=LINE ( 'NONE', #7207, #54377 ) ;
#57085=CARTESIAN_POINT ( 'NONE',  ( -5.099062320646999602, -80.14465347566299158, -10.07485988244000019 ) ) ;
#57087=CARTESIAN_POINT ( 'NONE',  ( -8.599842724110780878, -79.63167486684267260, -3.562057441230364052 ) ) ;
#57089=ORIENTED_EDGE ( 'NONE', *, *, #44844, .F. ) ;
#57096=CARTESIAN_POINT ( 'NONE',  ( 3.771615891982000424, -80.17905589940099276, -8.483472276358000386 ) ) ;
#57101=CARTESIAN_POINT ( 'NONE',  ( -2.935661446561999899, -76.94999999999998863, -9.035036904803998681 ) ) ;
#57103=CARTESIAN_POINT ( 'NONE',  ( 3.875771953607000331, -77.65343742103499380, 10.35502414757000089 ) ) ;
#57110=CARTESIAN_POINT ( 'NONE',  ( 2.309272084855999996, -76.85373069405538615, -9.392260232199999948 ) ) ;
#57111=CARTESIAN_POINT ( 'NONE',  ( 8.082524092276894834, -78.29166666666665719, 4.658475568430803904 ) ) ;
#57125=EDGE_CURVE ( 'NONE', #40036, #27720, #47216, .T. ) ;
#57134=CARTESIAN_POINT ( 'NONE',  ( 9.250000000000000000, -79.74999999999998579, 1.907449677260999760E-14 ) ) ;
#57146=CARTESIAN_POINT ( 'NONE',  ( -8.796335266380014062, -78.64791666666667425, 6.760013919724027431 ) ) ;
#57162=CARTESIAN_POINT ( 'NONE',  ( 1.684372618195999927, -78.17228479878399128, 10.84559388857000073 ) ) ;
#57165=ORIENTED_EDGE ( 'NONE', *, *, #34683, .F. ) ;
#57173=CARTESIAN_POINT ( 'NONE',  ( 4.108390852610000366, -78.61743808823698032, -8.590197950816000017 ) ) ;
#57181=CARTESIAN_POINT ( 'NONE',  ( -1.439896632895337980, -78.81458333333334565, -11.00000000000000178 ) ) ;
#57187=CARTESIAN_POINT ( 'NONE',  ( 8.665370346175000904, -80.06605154712399042, -7.125084804452000320 ) ) ;
#57196=CARTESIAN_POINT ( 'NONE',  ( 8.249323304235000265, -80.45505077665451665, -5.229696851825000437 ) ) ;
#57197=ORIENTED_EDGE ( 'NONE', *, *, #45373, .F. ) ;
#57212=CARTESIAN_POINT ( 'NONE',  ( -9.250000000000007105, -77.98958333333334281, 1.210822168571027868 ) ) ;
#57223=CARTESIAN_POINT ( 'NONE',  ( 7.618592589353999855, -77.25777915476199098, 5.659247346374999488 ) ) ;
#57238=CARTESIAN_POINT ( 'NONE',  ( 4.680902262334169173, -79.08410081236472422, 8.289971767921159085 ) ) ;
#57239=CARTESIAN_POINT ( 'NONE',  ( -3.924507919822526780, -80.00000000000002842, -8.550991966546336087 ) ) ;
#57242=CARTESIAN_POINT ( 'NONE',  ( -6.990927307832999205, -79.70827722813399419, 6.997322775002999151 ) ) ;
#57252=CARTESIAN_POINT ( 'NONE',  ( 9.067898462393999992, -77.63025123080397805, -6.404597993423999824 ) ) ;
#57255=CONICAL_SURFACE ( 'NONE', #12949, 5.249999999862000166, 0.7853981633972997312 ) ;
#57260=ORIENTED_EDGE ( 'NONE', *, *, #1000, .T. ) ;
#57266=CIRCLE ( 'NONE', #33715, 1.000000000000000000 ) ;
#57278=DIRECTION ( 'NONE',  ( 1.776356839400000238E-14, 1.000000000000000000, 2.516505522483999811E-14 ) ) ;
#57280=CARTESIAN_POINT ( 'NONE',  ( -8.272053489104999713, -78.68019927879299757, -7.648664291178000063 ) ) ;
#57281=CARTESIAN_POINT ( 'NONE',  ( 7.645574991865955461, -77.30253601357824778, -5.206776502330282774 ) ) ;
#57287=CARTESIAN_POINT ( 'NONE',  ( -9.250000000000000000, -77.59999999999999432, 0.000000000000000000 ) ) ;
#57291=CARTESIAN_POINT ( 'NONE',  ( -10.97221500190000043, -79.57146358532099839, -2.025363574538999956 ) ) ;
#57293=DIRECTION ( 'NONE',  ( -1.000000000000000000, 0.000000000000000000, 0.000000000000000000 ) ) ;
#57297=DIRECTION ( 'NONE',  ( -0.3090169943748909409, 0.000000000000000000, -0.9510565162951718499 ) ) ;
#57298=VERTEX_POINT ( 'NONE', #45739 ) ;
#57299=CARTESIAN_POINT ( 'NONE',  ( -4.245633743941748861, -77.20000000000000284, 9.989790920463677892 ) ) ;
#57305=DIRECTION ( 'NONE',  ( 0.000000000000000000, -1.000000000000000000, 0.000000000000000000 ) ) ;
#57315=VECTOR ( 'NONE', #10367, 1000.000000000000000 ) ;
#57318=CARTESIAN_POINT ( 'NONE',  ( -2.928603948516999900, -78.76634245677499280, 10.57767911662999971 ) ) ;
#57321=CARTESIAN_POINT ( 'NONE',  ( -10.86862532138029458, -79.68584017775069128, 1.957230818804138517 ) ) ;
#57323=ORIENTED_EDGE ( 'NONE', *, *, #36891, .F. ) ;
#57327=CARTESIAN_POINT ( 'NONE',  ( -8.796335266380014062, -78.14791666666667425, 6.760013919724027431 ) ) ;
#57328=CARTESIAN_POINT ( 'NONE',  ( 9.178372771442999678, -77.94661130901299373, -6.069379357596000446 ) ) ;
#57335=CARTESIAN_POINT ( 'NONE',  ( 0.000000000000000000, -76.29999999995945359, -10.59999999995999964 ) ) ;
#57337=DIRECTION ( 'NONE',  ( 1.000000000000000000, 0.000000000000000000, 0.000000000000000000 ) ) ;
#57342=CARTESIAN_POINT ( 'NONE',  ( -4.435886197818010857, -79.83672437013201773, -8.483855872844232593 ) ) ;
#57350=CARTESIAN_POINT ( 'NONE',  ( -1.407736081117633375, -78.21296968607886413, -9.142491334826452487 ) ) ;
#57352=ORIENTED_EDGE ( 'NONE', *, *, #26031, .F. ) ;
#57355=CARTESIAN_POINT ( 'NONE',  ( -4.388972190985573008, -77.51444041639624061, 8.142476534846730729 ) ) ;
#57359=CARTESIAN_POINT ( 'NONE',  ( -2.183112477083999803, -77.72320829419898303, 9.455407409464999802 ) ) ;
#57361=CIRCLE ( 'NONE', #39450, 10.50000000000000000 ) ;
#57364=CARTESIAN_POINT ( 'NONE',  ( -4.017143116098000455, -80.21358937413599222, 10.51352533724000082 ) ) ;
#57365=DIRECTION ( 'NONE',  ( 0.000000000000000000, 1.000000000000000000, 0.000000000000000000 ) ) ;
#57374=CARTESIAN_POINT ( 'NONE',  ( 8.081978225942579641, -78.39170613804414245, 4.658214607401315988 ) ) ;
#57388=CARTESIAN_POINT ( 'NONE',  ( 7.653972382670000130, -79.72123425335998093, -5.499357303777000716 ) ) ;
#57390=CARTESIAN_POINT ( 'NONE',  ( 9.873180114738437041, -77.20000000000000284, 4.400785053488170284 ) ) ;
#57392=DIRECTION ( 'NONE',  ( 0.000000000000000000, -1.000000000000000000, 0.000000000000000000 ) ) ;
#57397=CARTESIAN_POINT ( 'NONE',  ( 10.64494183963000040, -78.10762918024498447, -1.773784135661999883 ) ) ;
#57402=CARTESIAN_POINT ( 'NONE',  ( -3.591972190522999764, -77.11482436373709959, 8.980252640667000463 ) ) ;
#57413=CARTESIAN_POINT ( 'NONE',  ( 0.000000000000000000, -81.10000000285099020, 5.900000002850999792 ) ) ;
#57426=EDGE_CURVE ( 'NONE', #40455, #1033, #25022, .T. ) ;
#57439=CARTESIAN_POINT ( 'NONE',  ( -9.156831961090404093, -78.61148368715173262, -1.313898468327503899 ) ) ;
#57450=CARTESIAN_POINT ( 'NONE',  ( -9.250000000000000000, -79.49999999999998579, 1.813240672189999963E-14 ) ) ;
#57462=CARTESIAN_POINT ( 'NONE',  ( 4.710185975415000392, -77.55872832793998839, -8.400437955132002088 ) ) ;
#57466=ORIENTED_EDGE ( 'NONE', *, *, #2361, .F. ) ;
#57467=EDGE_CURVE ( 'NONE', #409, #16887, #15274, .T. ) ;
#57468=CARTESIAN_POINT ( 'NONE',  ( -10.71369944335147117, -78.72083333333330302, -2.879226727952077791 ) ) ;
#57472=CARTESIAN_POINT ( 'NONE',  ( -9.781527233834999890, -78.90776930244898324, -4.899953194656999855 ) ) ;
#57474=CARTESIAN_POINT ( 'NONE',  ( 8.751463191605999725, -80.00217580634098624, -7.195874488014000647 ) ) ;
#57476=AXIS2_PLACEMENT_3D ( 'NONE', #8895, #35153, #8021 ) ;
#57488=CARTESIAN_POINT ( 'NONE',  ( -7.000000000000000000, -81.99999999999998579, 0.000000000000000000 ) ) ;
#57493=CARTESIAN_POINT ( 'NONE',  ( 8.617899982024150418, -78.82053113868873595, -3.361248075313672423 ) ) ;
#57506=CARTESIAN_POINT ( 'NONE',  ( 2.240069435031999845, -77.16499869373629394, -9.110799550206998276 ) ) ;
#57521=CARTESIAN_POINT ( 'NONE',  ( -9.450981695478892775, -79.25824793529314150, -0.9830935124726688512 ) ) ;
#57522=CARTESIAN_POINT ( 'NONE',  ( 2.220128896776556893, -80.00000000000000000, -9.233834223992447576 ) ) ;
#57523=CARTESIAN_POINT ( 'NONE',  ( -9.611650271896857944, -79.05833333333333712, 5.539808784079855997 ) ) ;
#57525=CARTESIAN_POINT ( 'NONE',  ( 9.363799758325001221, -78.88336945908598352, -1.158156830125999903 ) ) ;
#57528=ORIENTED_EDGE ( 'NONE', *, *, #51094, .T. ) ;
#57530=FACE_OUTER_BOUND ( 'NONE', #10821, .T. ) ;
#57541=ORIENTED_EDGE ( 'NONE', *, *, #30039, .F. ) ;
#57544=CARTESIAN_POINT ( 'NONE',  ( -7.479908383216000267, -79.32543322980198752, -6.281056869080000382 ) ) ;
#57552=CARTESIAN_POINT ( 'NONE',  ( -4.100000000000000533, -78.69999999999998863, 0.000000000000000000 ) ) ;
#57559=CARTESIAN_POINT ( 'NONE',  ( 3.483691356461174227, -79.94435685530504543, 8.568905828578699868 ) ) ;
#57560=CARTESIAN_POINT ( 'NONE',  ( 0.000000000000000000, -74.64999999999999147, 0.000000000000000000 ) ) ;
#57561=ORIENTED_EDGE ( 'NONE', *, *, #51735, .T. ) ;
#57562=CARTESIAN_POINT ( 'NONE',  ( 4.019191877497999776, -79.46678520010797797, 10.52497178225999974 ) ) ;
#57563=CARTESIAN_POINT ( 'NONE',  ( 6.634060730155967534, -77.28871036968435249, -6.446087520221595923 ) ) ;
#57572=CARTESIAN_POINT ( 'NONE',  ( -10.83342013959000028, -79.03770885299998383, 2.669945268378000058 ) ) ;
#57579=CARTESIAN_POINT ( 'NONE',  ( -1.608404438602769160, -77.20000000000000284, 10.70099509088003487 ) ) ;
#57588=CARTESIAN_POINT ( 'NONE',  ( -1.173259754689000234, -78.82221935430098370, -9.559114633834001395 ) ) ;
#57598=CARTESIAN_POINT ( 'NONE',  ( 6.612939829087000732, -79.75369307542398190, 8.759739992124000452 ) ) ;
#57609=CARTESIAN_POINT ( 'NONE',  ( 9.855576673225998618, -79.45423432486698800, -5.230603033304000782 ) ) ;
#57627=CARTESIAN_POINT ( 'NONE',  ( -9.113568214466768680, -79.77523700399514439, -2.981120847293889486 ) ) ;
#57632=CARTESIAN_POINT ( 'NONE',  ( -8.411043104783766822, -78.13496630202740789, -3.922096619641943782 ) ) ;
#57636=CARTESIAN_POINT ( 'NONE',  ( -6.541840594602032155, -77.53768247343118958, 6.539477767634727101 ) ) ;
#57638=CARTESIAN_POINT ( 'NONE',  ( 9.391860901740999523, -77.16389274916278396, 5.803232400709999794 ) ) ;
#57641=CARTESIAN_POINT ( 'NONE',  ( -9.446433787353997857, -78.34853253503598580, -2.221620594898999990 ) ) ;
#57644=CARTESIAN_POINT ( 'NONE',  ( -9.254388464354001087, -79.80752053325198858, 5.469807505829999528 ) ) ;
#57645=CARTESIAN_POINT ( 'NONE',  ( -11.09141466634999951, -79.79597772074998829, 1.909950515085000022 ) ) ;
#57657=CARTESIAN_POINT ( 'NONE',  ( 11.11690205930000097, -80.32095930235598757, 1.979307181865000098 ) ) ;
#57681=CARTESIAN_POINT ( 'NONE',  ( -7.396918292183181975, -78.44791666666665719, 5.684557159767943624 ) ) ;
#57694=ORIENTED_EDGE ( 'NONE', *, *, #2262, .T. ) ;
#57719=CARTESIAN_POINT ( 'NONE',  ( -9.219307557399826436, -78.60653449301742057, -0.7524715728064156339 ) ) ;
#57731=ORIENTED_EDGE ( 'NONE', *, *, #33558, .T. ) ;
#57743=B_SPLINE_CURVE_WITH_KNOTS ( 'NONE', 3,
 ( #35289, #8161, #58337, #53319, #35888, #8441 ),
 .UNSPECIFIED., .F., .F.,
 ( 4, 2, 4 ),
 ( 0.000000000000000000, 0.5000000000000000000, 1.000000000000000000 ),
 .UNSPECIFIED. ) ;
#57749=CARTESIAN_POINT ( 'NONE',  ( -3.877711979005999954, -77.98508576487398614, -8.815699619024998768 ) ) ;
#57755=CARTESIAN_POINT ( 'NONE',  ( 5.539808784079872872, -78.86666666666668846, -9.611650271896849063 ) ) ;
#57759=CARTESIAN_POINT ( 'NONE',  ( -5.736605348686000028, -78.28973750712998481, 9.315534093342000332 ) ) ;
#57762=CARTESIAN_POINT ( 'NONE',  ( 10.49379773601000032, -80.14957387780098941, 3.966822966890999780 ) ) ;
#57784=CARTESIAN_POINT ( 'NONE',  ( 7.000000000000000000, -81.19999999999998863, 0.000000000000000000 ) ) ;
#57791=CARTESIAN_POINT ( 'NONE',  ( -5.539808784079933268, -78.01666666666665151, 9.611650271896811759 ) ) ;
#57799=FACE_OUTER_BOUND ( 'NONE', #29730, .T. ) ;
#57804=CARTESIAN_POINT ( 'NONE',  ( 0.000000000000000000, -80.99999999999998579, -7.000000000000000000 ) ) ;
#57816=CARTESIAN_POINT ( 'NONE',  ( -4.131840341030999397, -80.11747182528499422, 8.602031057089000399 ) ) ;
#57824=AXIS2_PLACEMENT_3D ( 'NONE', #44537, #48122, #25653 ) ;
#57836=CARTESIAN_POINT ( 'NONE',  ( 5.496668217546000434, -79.94241373670298856, -8.073860231047000013 ) ) ;
#57837=VERTEX_POINT ( 'NONE', #11394 ) ;
#57843=CARTESIAN_POINT ( 'NONE',  ( -5.351380825403158958, -77.77138628471922743, 8.095464844688041950 ) ) ;
#57853=CARTESIAN_POINT ( 'NONE',  ( 0.2479736929933408496, -79.97326530669452893, 9.253379769800089250 ) ) ;
#57856=CARTESIAN_POINT ( 'NONE',  ( -10.07307375010999984, -79.15776930244898324, -5.046000355766999235 ) ) ;
#57867=CARTESIAN_POINT ( 'NONE',  ( -2.205131412320000095, -78.44776941201399723, 10.93750404997000025 ) ) ;
#57881=CARTESIAN_POINT ( 'NONE',  ( -8.954089450906998593, -78.73694786691399372, -3.546476007522999740 ) ) ;
#57892=CARTESIAN_POINT ( 'NONE',  ( -10.90760146693999921, -78.93901479977699864, -1.219937219691999974 ) ) ;
#57900=CARTESIAN_POINT ( 'NONE',  ( 11.00000000000000178, -77.94292008887532575, -0.9786566581934403874 ) ) ;
#57904=CARTESIAN_POINT ( 'NONE',  ( 10.89322882296999850, -79.51041903353198848, 2.414366480783999958 ) ) ;
#57913=ORIENTED_EDGE ( 'NONE', *, *, #7840, .T. ) ;
#57924=CARTESIAN_POINT ( 'NONE',  ( -5.860166239445133485, -78.17045350272391602, -7.156831644022663141 ) ) ;
#57927=VECTOR ( 'NONE', #33252, 1000.000000000000000 ) ;
#57931=CARTESIAN_POINT ( 'NONE',  ( 1.731393780109722336, -77.46006980321932645, 9.086687499499138454 ) ) ;
#57932=CARTESIAN_POINT ( 'NONE',  ( -11.00724581733999941, -77.80340341412998839, 0.8512868710715000287 ) ) ;
#57937=CARTESIAN_POINT ( 'NONE',  ( 10.52776997023000050, -80.14860880379099228, 3.979665013433000720 ) ) ;
#57940=AXIS2_PLACEMENT_3D ( 'NONE', #31092, #448, #44997 ) ;
#57942=CARTESIAN_POINT ( 'NONE',  ( 9.250000000000001776, -78.73958333333334281, -1.210822168571047186 ) ) ;
#57964=CARTESIAN_POINT ( 'NONE',  ( 9.366332946604000398, -79.77967956987598086, 1.047869802319999932 ) ) ;
#57966=CARTESIAN_POINT ( 'NONE',  ( 8.030130101452463975, -77.19999999999998863, 7.236483772011231608 ) ) ;
#57981=CARTESIAN_POINT ( 'NONE',  ( 0.000000000000000000, -81.19999999999998863, -7.000000000000000000 ) ) ;
#57984=CIRCLE ( 'NONE', #15563, 5.000000000000000000 ) ;
#57989=EDGE_LOOP ( 'NONE', ( #12264, #32642, #6808, #33565 ) ) ;
#58008=CARTESIAN_POINT ( 'NONE',  ( 7.256139241522999939, -77.51733095546998698, 6.443535727668999513 ) ) ;
#58016=CARTESIAN_POINT ( 'NONE',  ( -9.247438236293723079, -78.60230166250890704, -0.2676552778266205190 ) ) ;
#58027=ORIENTED_EDGE ( 'NONE', *, *, #4555, .T. ) ;
#58028=CARTESIAN_POINT ( 'NONE',  ( 9.249769291450279596, -78.85065788838248579, 0.06519237146997462762 ) ) ;
#58038=CARTESIAN_POINT ( 'NONE',  ( -2.049109721976000387, -77.06873060082338611, 11.08635720663000157 ) ) ;
#58041=CARTESIAN_POINT ( 'NONE',  ( -5.250896469870999006, -77.87841853088399091, 7.943454065752000304 ) ) ;
#58049=CARTESIAN_POINT ( 'NONE',  ( 2.879226727952061360, -78.84583333333328881, -10.71369944335147650 ) ) ;
#58054=CARTESIAN_POINT ( 'NONE',  ( 7.294482259529999624, -79.55389345209998453, -8.153425347847999660 ) ) ;
#58057=CARTESIAN_POINT ( 'NONE',  ( -10.73093511375999753, -79.77125540420298933, -3.969369046568999693 ) ) ;
#58067=DIRECTION ( 'NONE',  ( 0.000000000000000000, -1.000000000000000000, 0.000000000000000000 ) ) ;
#58079=DIRECTION ( 'NONE',  ( -1.000000000000000000, 0.000000000000000000, 0.000000000000000000 ) ) ;
#58090=EDGE_CURVE ( 'NONE', #33386, #31248, #43263, .T. ) ;
#58110=CARTESIAN_POINT ( 'NONE',  ( 7.919085842678998510, -79.02973936012098477, -5.669895566145999766 ) ) ;
#58130=CARTESIAN_POINT ( 'NONE',  ( -9.387315177295000979, -79.74757778715598988, 2.697965643110000311 ) ) ;
#58139=CARTESIAN_POINT ( 'NONE',  ( -3.907294856124924110, -77.94192925949296580, -8.882954164993476454 ) ) ;
#58158=CARTESIAN_POINT ( 'NONE',  ( 6.657089793739999983, -79.81660374219698895, 8.818222636911000833 ) ) ;
#58174=CARTESIAN_POINT ( 'NONE',  ( 1.236990682704000033, -77.50769513184299342, 9.441410396910001168 ) ) ;
#58185=CARTESIAN_POINT ( 'NONE',  ( 8.212410987726999068, -78.18463944979998814, -6.936771999183999782 ) ) ;
#58193=CARTESIAN_POINT ( 'NONE',  ( 9.022184164167814657, -77.23121341071495749, -2.164508873546484580 ) ) ;
#58197=CARTESIAN_POINT ( 'NONE',  ( 7.917622607290999426, -78.55527898622098348, 7.861478989701000231 ) ) ;
#58212=CARTESIAN_POINT ( 'NONE',  ( 3.367278140553823462, -79.59625721410608890, 8.916401300557922127 ) ) ;
#58216=DIRECTION ( 'NONE',  ( -0.7071067811865470176, -0.7071067811865470176, -3.680441204124245327E-08 ) ) ;
#58224=CARTESIAN_POINT ( 'NONE',  ( 2.425090211683515573, -77.45404813181065151, 8.927162646165987425 ) ) ;
#58225=CARTESIAN_POINT ( 'NONE',  ( 2.386167682861000117, -77.28781509216399570, 10.77916482977000001 ) ) ;
#58226=CONICAL_SURFACE ( 'NONE', #24272, 4.199999999630000147, 0.7853981633972997312 ) ;
#58227=CARTESIAN_POINT ( 'NONE',  ( 5.927986824875999261, -78.06774951115899341, -7.683077610609999830 ) ) ;
#58231=CARTESIAN_POINT ( 'NONE',  ( 1.791008777272000030, -80.35273698580898838, 11.11143388882000060 ) ) ;
#58260=CARTESIAN_POINT ( 'NONE',  ( -9.384564006317999585, -80.01346083593999481, 0.8695881376670999696 ) ) ;
#58261=CARTESIAN_POINT ( 'NONE',  ( 7.000000000000000000, -81.10000000285099020, 0.000000000000000000 ) ) ;
#58281=DIRECTION ( 'NONE',  ( 0.000000000000000000, 0.000000000000000000, -1.000000000000000000 ) ) ;
#58282=CARTESIAN_POINT ( 'NONE',  ( 8.796335266379987416, -79.40208333333335133, 6.760013919724053189 ) ) ;
#58288=EDGE_LOOP ( 'NONE', ( #46143, #34965, #15470, #54382 ) ) ;
#58292=CARTESIAN_POINT ( 'NONE',  ( 8.693423296916000353, -80.04523846126194542, -7.148151291522000683 ) ) ;
#58300=CARTESIAN_POINT ( 'NONE',  ( 2.993649408183152616, -77.20255476765863989, 10.33029624542498226 ) ) ;
#58303=ORIENTED_EDGE ( 'NONE', *, *, #10059, .T. ) ;
#58308=CARTESIAN_POINT ( 'NONE',  ( 7.405962610586999340, -77.40363563895398613, -6.270759699041999369 ) ) ;
#58325=ORIENTED_EDGE ( 'NONE', *, *, #22348, .F. ) ;
#58326=CARTESIAN_POINT ( 'NONE',  ( 9.249938314532530015, -78.85038283385668478, 0.03259585398855812527 ) ) ;
#58337=CARTESIAN_POINT ( 'NONE',  ( 8.718213946484933530, -76.96041666667038328, -3.877033208488974925 ) ) ;
#58340=CARTESIAN_POINT ( 'NONE',  ( 7.120006596302999924, -77.76472321436799007, 6.322648361264000094 ) ) ;
#58349=ORIENTED_EDGE ( 'NONE', *, *, #23912, .T. ) ;
#58352=CARTESIAN_POINT ( 'NONE',  ( 6.591600424694998850, -79.69435522376399206, 8.731473042948000085 ) ) ;
#58354=CARTESIAN_POINT ( 'NONE',  ( -2.600000000000000089, -77.49999999999998579, 0.000000000000000000 ) ) ;
#58355=VERTEX_POINT ( 'NONE', #53560 ) ;
#58360=AXIS2_PLACEMENT_3D ( 'NONE', #25341, #39780, #21201 ) ;
#58361=EDGE_CURVE ( 'NONE', #13326, #9068, #1108, .T. ) ;
#58363=CARTESIAN_POINT ( 'NONE',  ( 8.193575559979001000, -79.54581634543151836, 5.316613930189999948 ) ) ;
#58374=CARTESIAN_POINT ( 'NONE',  ( 7.258298179997606958, -78.79682822265634456, -5.734190774355525377 ) ) ;
#58377=EDGE_CURVE ( 'NONE', #21227, #55354, #4610, .T. ) ;
#58381=CARTESIAN_POINT ( 'NONE',  ( -11.00000000000000888, -78.08958333333330870, 1.439896632895276252 ) ) ;
#58383=CARTESIAN_POINT ( 'NONE',  ( -3.023821996898440112, -79.99699371105347723, 10.64354645710085023 ) ) ;
#58397=CARTESIAN_POINT ( 'NONE',  ( 0.000000000000000000, -81.89999999962999766, 0.000000000000000000 ) ) ;
ENDSEC;
END-ISO-10303-21;
